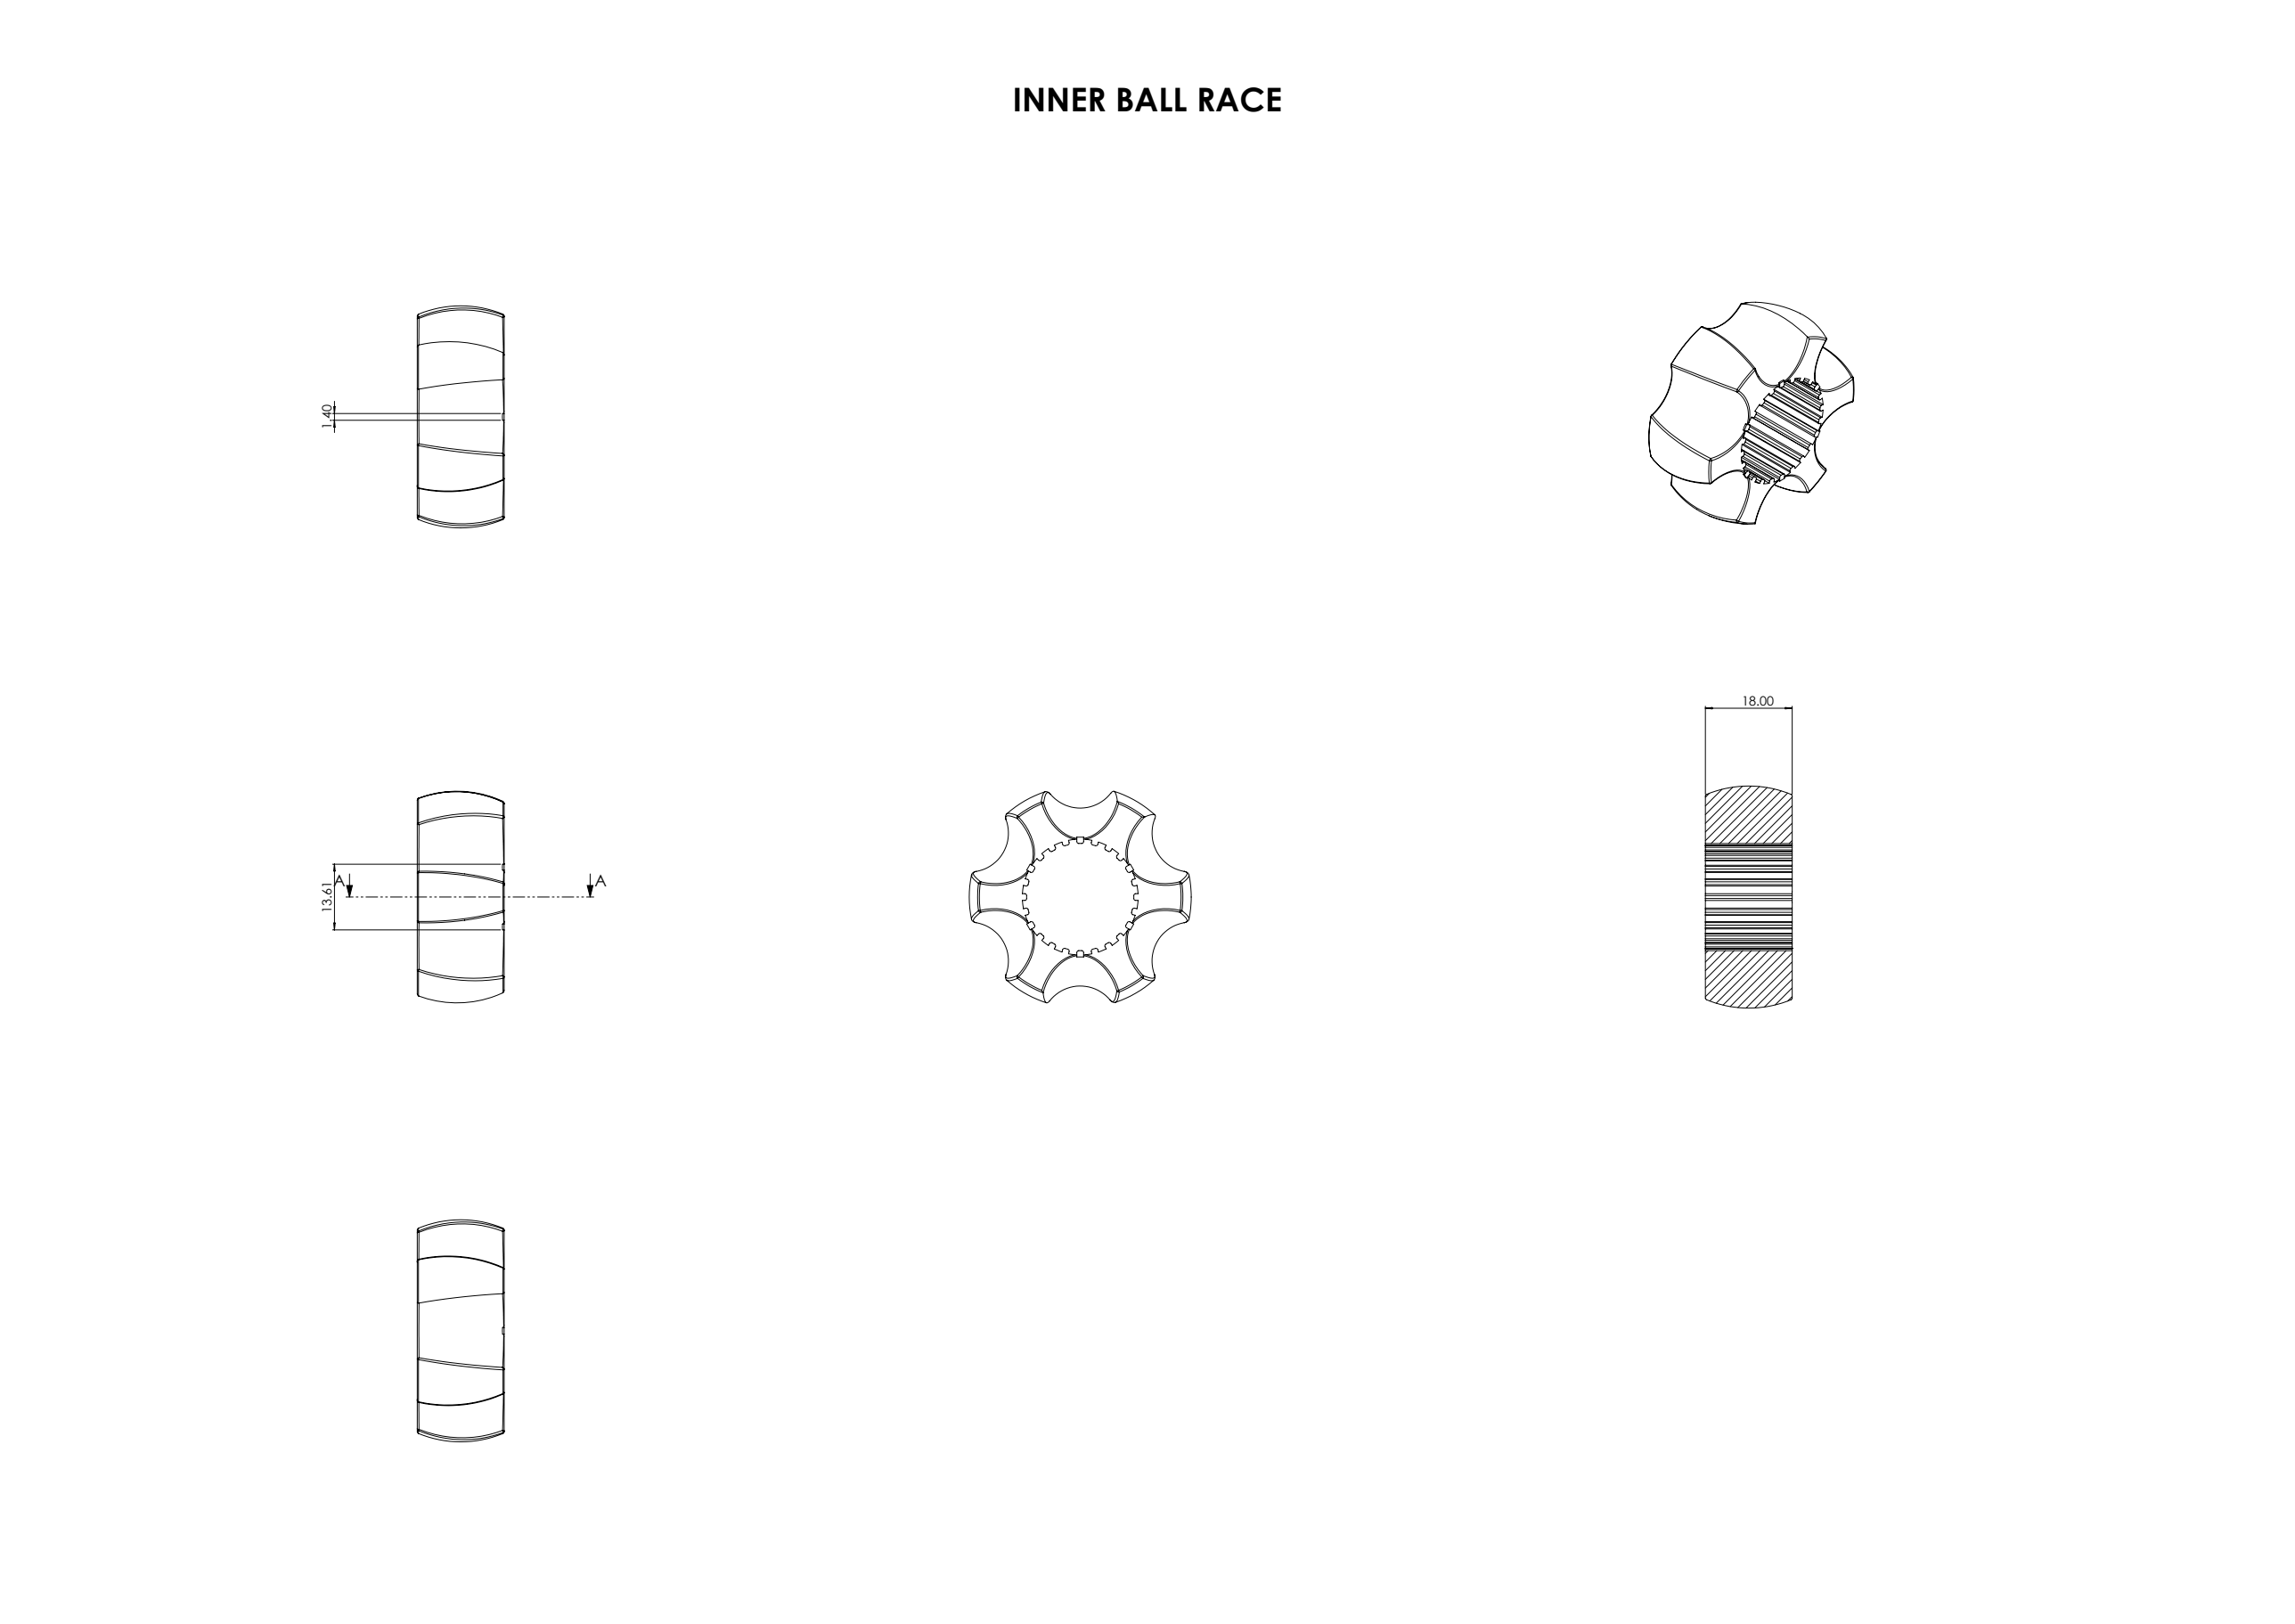
ISO-10303-21;
HEADER;
/* Generated by software containing ST-Developer
 * from STEP Tools, Inc. (www.steptools.com) 
 */

FILE_DESCRIPTION(
/* description */ (''),
/* implementation_level */ '2;1');

FILE_NAME(
/* name */ '04_Inner_Ball_Race.step',
/* time_stamp */ '2026-10-11T12:57:03-07:00',
/* author */ (''),
/* organization */ (''),
/* preprocessor_version */ 'ST-DEVELOPER v20.2',
/* originating_system */ 'Autodesk Translation Framework v15.15.0.0',
/* authorisation */ '');

FILE_SCHEMA (('AUTOMOTIVE_DESIGN { 1 0 10303 214 3 1 1 }'));
ENDSEC;

DATA;
#10=MECHANICAL_DESIGN_GEOMETRIC_PRESENTATION_REPRESENTATION('',(#259),#90374);
#225=SHAPE_REPRESENTATION_RELATIONSHIP('SRR','None',#90444,#242);
#242=ADVANCED_BREP_SHAPE_REPRESENTATION('',(#276),#90360);
#259=STYLED_ITEM('',(#90680),#276);
#276=MANIFOLD_SOLID_BREP('Body1',#40348);
#533=SPHERICAL_SURFACE('',#43538,0.4);
#534=SPHERICAL_SURFACE('',#43541,0.4);
#535=SPHERICAL_SURFACE('',#43552,0.4);
#536=SPHERICAL_SURFACE('',#43555,0.4);
#537=SPHERICAL_SURFACE('',#43561,23.);
#538=SPHERICAL_SURFACE('',#43563,0.4);
#539=SPHERICAL_SURFACE('',#43569,0.4);
#540=SPHERICAL_SURFACE('',#43581,0.4);
#541=SPHERICAL_SURFACE('',#43589,0.4);
#542=SPHERICAL_SURFACE('',#43591,0.4);
#543=SPHERICAL_SURFACE('',#43600,0.4);
#544=SPHERICAL_SURFACE('',#43603,0.4);
#545=SPHERICAL_SURFACE('',#43607,23.);
#546=SPHERICAL_SURFACE('',#43612,0.4);
#547=SPHERICAL_SURFACE('',#43616,0.399999999999991);
#548=SPHERICAL_SURFACE('',#43619,0.4);
#549=SPHERICAL_SURFACE('',#43625,0.4);
#550=SPHERICAL_SURFACE('',#43629,0.4);
#551=SPHERICAL_SURFACE('',#43632,23.);
#552=SPHERICAL_SURFACE('',#43635,0.4);
#553=SPHERICAL_SURFACE('',#43638,23.);
#554=SPHERICAL_SURFACE('',#43641,0.4);
#555=SPHERICAL_SURFACE('',#43650,23.);
#556=SPHERICAL_SURFACE('',#43653,23.);
#973=TOROIDAL_SURFACE('',#43544,20.899760764181,0.4);
#974=TOROIDAL_SURFACE('',#43547,26.4764045897475,8.05);
#975=TOROIDAL_SURFACE('',#43558,20.899760764181,0.4);
#976=TOROIDAL_SURFACE('',#43566,20.899760764181,0.4);
#977=TOROIDAL_SURFACE('',#43573,20.899760764181,0.4);
#978=TOROIDAL_SURFACE('',#43578,26.4764045897475,8.05);
#979=TOROIDAL_SURFACE('',#43584,20.899760764181,0.4);
#980=TOROIDAL_SURFACE('',#43593,20.899760764181,0.4);
#981=TOROIDAL_SURFACE('',#43596,26.4764045897475,8.05);
#982=TOROIDAL_SURFACE('',#43605,20.899760764181,0.4);
#983=TOROIDAL_SURFACE('',#43609,20.899760764181,0.4);
#984=TOROIDAL_SURFACE('',#43610,20.899760764181,0.4);
#985=TOROIDAL_SURFACE('',#43615,26.4764045897475,8.05);
#986=TOROIDAL_SURFACE('',#43623,20.899760764181,0.4);
#987=TOROIDAL_SURFACE('',#43634,26.4764045897475,8.05);
#988=TOROIDAL_SURFACE('',#43645,20.899760764181,0.4);
#989=TOROIDAL_SURFACE('',#43647,26.4764045897475,8.05);
#990=TOROIDAL_SURFACE('',#43651,20.899760764181,0.4);
#1052=FACE_BOUND('',#5964,.T.);
#1329=PLANE('',#43279);
#1330=PLANE('',#43281);
#1331=PLANE('',#43287);
#1332=PLANE('',#43288);
#1333=PLANE('',#43366);
#1334=PLANE('',#43367);
#1335=PLANE('',#43378);
#1336=PLANE('',#43381);
#1337=PLANE('',#43385);
#1338=PLANE('',#43387);
#1339=PLANE('',#43391);
#1340=PLANE('',#43402);
#1341=PLANE('',#43405);
#1342=PLANE('',#43407);
#1343=PLANE('',#43409);
#1344=PLANE('',#43411);
#1345=PLANE('',#43414);
#1346=PLANE('',#43418);
#1347=PLANE('',#43420);
#1348=PLANE('',#43423);
#1349=PLANE('',#43434);
#1350=PLANE('',#43437);
#1351=PLANE('',#43439);
#1352=PLANE('',#43441);
#1353=PLANE('',#43443);
#1354=PLANE('',#43446);
#1355=PLANE('',#43450);
#1356=PLANE('',#43452);
#1357=PLANE('',#43455);
#1358=PLANE('',#43466);
#1359=PLANE('',#43469);
#1360=PLANE('',#43471);
#1361=PLANE('',#43473);
#1362=PLANE('',#43475);
#1363=PLANE('',#43478);
#1364=PLANE('',#43482);
#1365=PLANE('',#43484);
#1366=PLANE('',#43487);
#1367=PLANE('',#43498);
#1368=PLANE('',#43501);
#1369=PLANE('',#43503);
#1370=PLANE('',#43505);
#1371=PLANE('',#43507);
#1372=PLANE('',#43510);
#1373=PLANE('',#43514);
#1374=PLANE('',#43516);
#1375=PLANE('',#43519);
#1376=PLANE('',#43530);
#1377=PLANE('',#43533);
#1378=PLANE('',#43535);
#1379=PLANE('',#43655);
#1380=PLANE('',#43657);
#1381=PLANE('',#43658);
#1382=PLANE('',#43660);
#1383=PLANE('',#43663);
#1384=PLANE('',#43664);
#1385=PLANE('',#43665);
#1386=PLANE('',#43666);
#1387=PLANE('',#43668);
#1388=PLANE('',#43670);
#1389=PLANE('',#43673);
#1390=PLANE('',#43674);
#1391=PLANE('',#43675);
#1392=PLANE('',#43676);
#1393=PLANE('',#43678);
#1394=PLANE('',#43680);
#1395=PLANE('',#43682);
#1396=PLANE('',#43683);
#1397=PLANE('',#43684);
#1398=PLANE('',#43685);
#1399=PLANE('',#43687);
#1400=PLANE('',#43689);
#1401=PLANE('',#43692);
#1402=PLANE('',#43693);
#1403=PLANE('',#43694);
#1404=PLANE('',#43695);
#1405=PLANE('',#43697);
#1406=PLANE('',#43699);
#1407=PLANE('',#43702);
#1408=PLANE('',#43703);
#1409=PLANE('',#43704);
#1410=PLANE('',#43705);
#1411=PLANE('',#43706);
#1412=PLANE('',#43708);
#1413=PLANE('',#43709);
#1414=PLANE('',#43710);
#1415=PLANE('',#43711);
#1416=PLANE('',#43713);
#1417=PLANE('',#43716);
#1418=PLANE('',#43717);
#1419=PLANE('',#43718);
#2106=B_SPLINE_SURFACE_WITH_KNOTS('',3,3,((#79480,#79481,#79482,#79483,
#79484),(#79485,#79486,#79487,#79488,#79489),(#79490,#79491,#79492,#79493,
#79494),(#79495,#79496,#79497,#79498,#79499),(#79500,#79501,#79502,#79503,
#79504)),.UNSPECIFIED.,.F.,.F.,.F.,(4,1,4),(4,1,4),(0.,0.5,1.),(0.,0.763473638149737,
1.78143848901605),.UNSPECIFIED.);
#2107=B_SPLINE_SURFACE_WITH_KNOTS('',3,3,((#79531,#79532,#79533,#79534,
#79535,#79536),(#79537,#79538,#79539,#79540,#79541,#79542),(#79543,#79544,
#79545,#79546,#79547,#79548),(#79549,#79550,#79551,#79552,#79553,#79554),
(#79555,#79556,#79557,#79558,#79559,#79560)),.UNSPECIFIED.,.F.,.F.,.F.,
(4,1,4),(4,1,1,4),(0.,0.5,1.),(0.285566041444528,0.852705185028571,1.23079794741793,
1.6088907098073),.UNSPECIFIED.);
#2108=B_SPLINE_SURFACE_WITH_KNOTS('',3,3,((#79645,#79646,#79647,#79648,
#79649),(#79650,#79651,#79652,#79653,#79654),(#79655,#79656,#79657,#79658,
#79659),(#79660,#79661,#79662,#79663,#79664),(#79665,#79666,#79667,#79668,
#79669)),.UNSPECIFIED.,.F.,.F.,.F.,(4,1,4),(4,1,4),(0.,0.5,1.),(0.,0.763473638150805,
1.78143848901855),.UNSPECIFIED.);
#2109=B_SPLINE_SURFACE_WITH_KNOTS('',3,3,((#79692,#79693,#79694,#79695,
#79696,#79697),(#79698,#79699,#79700,#79701,#79702,#79703),(#79704,#79705,
#79706,#79707,#79708,#79709),(#79710,#79711,#79712,#79713,#79714,#79715),
(#79716,#79717,#79718,#79719,#79720,#79721)),.UNSPECIFIED.,.F.,.F.,.F.,
(4,1,4),(4,1,1,4),(0.,0.5,1.),(1.29377116963159,1.60639339394931,1.91901561826703,
2.38794895474362),.UNSPECIFIED.);
#2110=B_SPLINE_SURFACE_WITH_KNOTS('',3,3,((#79782,#79783,#79784,#79785,
#79786,#79787),(#79788,#79789,#79790,#79791,#79792,#79793),(#79794,#79795,
#79796,#79797,#79798,#79799),(#79800,#79801,#79802,#79803,#79804,#79805),
(#79806,#79807,#79808,#79809,#79810,#79811)),.UNSPECIFIED.,.F.,.F.,.F.,
(4,1,4),(4,1,1,4),(0.,0.5,1.),(0.738839250765249,1.30597756136174,1.68406976842606,
2.06216197549039),.UNSPECIFIED.);
#2111=B_SPLINE_SURFACE_WITH_KNOTS('',3,3,((#79835,#79836,#79837,#79838,
#79839,#79840),(#79841,#79842,#79843,#79844,#79845,#79846),(#79847,#79848,
#79849,#79850,#79851,#79852),(#79853,#79854,#79855,#79856,#79857,#79858),
(#79859,#79860,#79861,#79862,#79863,#79864)),.UNSPECIFIED.,.F.,.F.,.F.,
(4,1,4),(4,1,1,4),(0.,0.5,1.),(0.263863277597402,0.819957327863798,1.19068669470806,
1.56141606155233),.UNSPECIFIED.);
#2112=B_SPLINE_SURFACE_WITH_KNOTS('',3,3,((#79879,#79880,#79881,#79882,
#79883),(#79884,#79885,#79886,#79887,#79888),(#79889,#79890,#79891,#79892,
#79893),(#79894,#79895,#79896,#79897,#79898),(#79899,#79900,#79901,#79902,
#79903)),.UNSPECIFIED.,.F.,.F.,.F.,(4,1,4),(4,1,4),(0.,0.5,1.),(0.805732136131231,
1.56919017940703,2.5871342371081),.UNSPECIFIED.);
#2113=B_SPLINE_SURFACE_WITH_KNOTS('',3,3,((#79949,#79950,#79951,#79952,
#79953),(#79954,#79955,#79956,#79957,#79958),(#79959,#79960,#79961,#79962,
#79963),(#79964,#79965,#79966,#79967,#79968),(#79969,#79970,#79971,#79972,
#79973)),.UNSPECIFIED.,.F.,.F.,.F.,(4,1,4),(4,1,4),(0.,0.5,1.),(0.,0.763473508304906,
1.78143818604478),.UNSPECIFIED.);
#2114=B_SPLINE_SURFACE_WITH_KNOTS('',3,3,((#80008,#80009,#80010,#80011,
#80012,#80013),(#80014,#80015,#80016,#80017,#80018,#80019),(#80020,#80021,
#80022,#80023,#80024,#80025),(#80026,#80027,#80028,#80029,#80030,#80031),
(#80032,#80033,#80034,#80035,#80036,#80037)),.UNSPECIFIED.,.F.,.F.,.F.,
(4,1,4),(4,1,1,4),(0.,0.5,1.),(0.232788919908364,0.858032407070129,1.01434327886057,
1.32696502244145),.UNSPECIFIED.);
#2115=B_SPLINE_SURFACE_WITH_KNOTS('',3,3,((#80074,#80075,#80076,#80077,
#80078,#80079),(#80080,#80081,#80082,#80083,#80084,#80085),(#80086,#80087,
#80088,#80089,#80090,#80091),(#80092,#80093,#80094,#80095,#80096,#80097),
(#80098,#80099,#80100,#80101,#80102,#80103)),.UNSPECIFIED.,.F.,.F.,.F.,
(4,1,4),(4,1,1,4),(0.,0.5,1.),(0.764611228840875,1.32070527910915,1.69143464595466,
2.06216401280017),.UNSPECIFIED.);
#2116=B_SPLINE_SURFACE_WITH_KNOTS('',3,3,((#80105,#80106,#80107,#80108,
#80109),(#80110,#80111,#80112,#80113,#80114),(#80115,#80116,#80117,#80118,
#80119),(#80120,#80121,#80122,#80123,#80124),(#80125,#80126,#80127,#80128,
#80129)),.UNSPECIFIED.,.F.,.F.,.F.,(4,1,4),(4,1,4),(0.,0.5,1.),(0.,0.763473564994705,
1.78143831832098),.UNSPECIFIED.);
#2117=B_SPLINE_SURFACE_WITH_KNOTS('',3,3,((#80144,#80145,#80146,#80147,
#80148,#80149),(#80150,#80151,#80152,#80153,#80154,#80155),(#80156,#80157,
#80158,#80159,#80160,#80161),(#80162,#80163,#80164,#80165,#80166,#80167),
(#80168,#80169,#80170,#80171,#80172,#80173)),.UNSPECIFIED.,.F.,.F.,.F.,
(4,1,4),(4,1,1,4),(0.,0.5,1.),(1.46996194814535,1.78258352306356,2.09520509798177,
2.56413746035908),.UNSPECIFIED.);
#2118=B_SPLINE_SURFACE_WITH_KNOTS('',3,3,((#80260,#80261,#80262,#80263,
#80264,#80265),(#80266,#80267,#80268,#80269,#80270,#80271),(#80272,#80273,
#80274,#80275,#80276,#80277),(#80278,#80279,#80280,#80281,#80282,#80283),
(#80284,#80285,#80286,#80287,#80288,#80289)),.UNSPECIFIED.,.F.,.F.,.F.,
(4,1,4),(4,1,1,4),(0.,0.5,1.),(0.285566041444524,0.663658803833889,1.04175156622325,
1.6088907098073),.UNSPECIFIED.);
#2119=B_SPLINE_SURFACE_WITH_KNOTS('',3,3,((#80312,#80313,#80314,#80315,
#80316,#80317),(#80318,#80319,#80320,#80321,#80322,#80323),(#80324,#80325,
#80326,#80327,#80328,#80329),(#80330,#80331,#80332,#80333,#80334,#80335),
(#80336,#80337,#80338,#80339,#80340,#80341)),.UNSPECIFIED.,.F.,.F.,.F.,
(4,1,4),(4,1,1,4),(0.,0.5,1.),(0.232788566406526,0.70171854409386,1.01433852921875,
1.32695851434364),.UNSPECIFIED.);
#2120=B_SPLINE_SURFACE_WITH_KNOTS('',3,3,((#80358,#80359,#80360,#80361,
#80362,#80363),(#80364,#80365,#80366,#80367,#80368,#80369),(#80370,#80371,
#80372,#80373,#80374,#80375),(#80376,#80377,#80378,#80379,#80380,#80381),
(#80382,#80383,#80384,#80385,#80386,#80387)),.UNSPECIFIED.,.F.,.F.,.F.,
(4,1,4),(4,1,1,4),(0.,0.5,1.),(0.263863277598129,0.819957327864215,1.19068669470827,
1.56141606155233),.UNSPECIFIED.);
#2121=B_SPLINE_SURFACE_WITH_KNOTS('',3,3,((#80394,#80395,#80396,#80397,
#80398,#80399),(#80400,#80401,#80402,#80403,#80404,#80405),(#80406,#80407,
#80408,#80409,#80410,#80411),(#80412,#80413,#80414,#80415,#80416,#80417),
(#80418,#80419,#80420,#80421,#80422,#80423)),.UNSPECIFIED.,.F.,.F.,.F.,
(4,1,4),(4,1,1,4),(0.,0.5,1.),(1.38151698616895,1.53782715631916,1.85044749661957,
2.47568817722038),.UNSPECIFIED.);
#2122=B_SPLINE_SURFACE_WITH_KNOTS('',3,3,((#80434,#80435,#80436,#80437,
#80438),(#80439,#80440,#80441,#80442,#80443),(#80444,#80445,#80446,#80447,
#80448),(#80449,#80450,#80451,#80452,#80453),(#80454,#80455,#80456,#80457,
#80458)),.UNSPECIFIED.,.F.,.F.,.F.,(4,1,4),(4,1,4),(0.,0.5,1.),(0.836467246372547,
1.5999252909985,2.61786935049977),.UNSPECIFIED.);
#2123=B_SPLINE_SURFACE_WITH_KNOTS('',3,3,((#80469,#80470,#80471,#80472,
#80473),(#80474,#80475,#80476,#80477,#80478),(#80479,#80480,#80481,#80482,
#80483),(#80484,#80485,#80486,#80487,#80488),(#80489,#80490,#80491,#80492,
#80493)),.UNSPECIFIED.,.F.,.F.,.F.,(4,1,4),(4,1,4),(0.,0.5,1.),(0.733284842491785,
1.49674691578015,2.51469634683131),.UNSPECIFIED.);
#2124=B_SPLINE_SURFACE_WITH_KNOTS('',3,3,((#80508,#80509,#80510,#80511,
#80512,#80513),(#80514,#80515,#80516,#80517,#80518,#80519),(#80520,#80521,
#80522,#80523,#80524,#80525),(#80526,#80527,#80528,#80529,#80530,#80531),
(#80532,#80533,#80534,#80535,#80536,#80537)),.UNSPECIFIED.,.F.,.F.,.F.,
(4,1,4),(4,1,1,4),(0.,0.5,1.),(1.11836314594235,1.58729550831966,1.89991708323787,
2.21253865815608),.UNSPECIFIED.);
#2125=B_SPLINE_SURFACE_WITH_KNOTS('',3,3,((#80555,#80556,#80557,#80558,
#80559,#80560),(#80561,#80562,#80563,#80564,#80565,#80566),(#80567,#80568,
#80569,#80570,#80571,#80572),(#80573,#80574,#80575,#80576,#80577,#80578),
(#80579,#80580,#80581,#80582,#80583,#80584)),.UNSPECIFIED.,.F.,.F.,.F.,
(4,1,4),(4,1,1,4),(0.,0.5,1.),(0.261933028354804,0.750578938128915,1.07634287797832,
1.40210681782773),.UNSPECIFIED.);
#2126=B_SPLINE_SURFACE_WITH_KNOTS('',3,3,((#80601,#80602,#80603,#80604,
#80605),(#80606,#80607,#80608,#80609,#80610),(#80611,#80612,#80613,#80614,
#80615),(#80616,#80617,#80618,#80619,#80620),(#80621,#80622,#80623,#80624,
#80625)),.UNSPECIFIED.,.F.,.F.,.F.,(4,1,4),(4,1,4),(0.,0.5,1.),(0.836467246372557,
1.59992529099851,2.61786935049979),.UNSPECIFIED.);
#2127=B_SPLINE_SURFACE_WITH_KNOTS('',3,3,((#80631,#80632,#80633,#80634,
#80635,#80636),(#80637,#80638,#80639,#80640,#80641,#80642),(#80643,#80644,
#80645,#80646,#80647,#80648),(#80649,#80650,#80651,#80652,#80653,#80654),
(#80655,#80656,#80657,#80658,#80659,#80660)),.UNSPECIFIED.,.F.,.F.,.F.,
(4,1,4),(4,1,1,4),(0.,0.5,1.),(1.38152124201424,1.53783209167054,1.85045379098313,
2.47569718960832),.UNSPECIFIED.);
#2128=B_SPLINE_SURFACE_WITH_KNOTS('',3,3,((#80686,#80687,#80688,#80689,
#80690),(#80691,#80692,#80693,#80694,#80695),(#80696,#80697,#80698,#80699,
#80700),(#80701,#80702,#80703,#80704,#80705),(#80706,#80707,#80708,#80709,
#80710)),.UNSPECIFIED.,.F.,.F.,.F.,(4,1,4),(4,1,4),(0.,0.5,1.),(0.733284842491785,
1.49674691578015,2.51469634683131),.UNSPECIFIED.);
#2129=B_SPLINE_SURFACE_WITH_KNOTS('',3,3,((#80730,#80731,#80732,#80733,
#80734,#80735),(#80736,#80737,#80738,#80739,#80740,#80741),(#80742,#80743,
#80744,#80745,#80746,#80747),(#80748,#80749,#80750,#80751,#80752,#80753),
(#80754,#80755,#80756,#80757,#80758,#80759)),.UNSPECIFIED.,.F.,.F.,.F.,
(4,1,4),(4,1,1,4),(0.,0.5,1.),(1.11836314594235,1.58729550831966,1.89991708323787,
2.21253865815608),.UNSPECIFIED.);
#2130=B_SPLINE_SURFACE_WITH_KNOTS('',3,3,((#80787,#80788,#80789,#80790,
#80791,#80792),(#80793,#80794,#80795,#80796,#80797,#80798),(#80799,#80800,
#80801,#80802,#80803,#80804),(#80805,#80806,#80807,#80808,#80809,#80810),
(#80811,#80812,#80813,#80814,#80815,#80816)),.UNSPECIFIED.,.F.,.F.,.F.,
(4,1,4),(4,1,1,4),(0.,0.5,1.),(1.54510505491245,1.70141616706786,2.0140383913787,
2.63928284000037),.UNSPECIFIED.);
#2131=B_SPLINE_SURFACE_WITH_KNOTS('',3,3,((#80847,#80848,#80849,#80850,
#80851,#80852),(#80853,#80854,#80855,#80856,#80857,#80858),(#80859,#80860,
#80861,#80862,#80863,#80864),(#80865,#80866,#80867,#80868,#80869,#80870),
(#80871,#80872,#80873,#80874,#80875,#80876)),.UNSPECIFIED.,.F.,.F.,.F.,
(4,1,4),(4,1,1,4),(0.,0.5,1.),(0.261933028354807,0.750578938128917,1.07634287797832,
1.40210681782773),.UNSPECIFIED.);
#2132=B_SPLINE_SURFACE_WITH_KNOTS('',3,3,((#80926,#80927,#80928,#80929,
#80930,#80931),(#80932,#80933,#80934,#80935,#80936,#80937),(#80938,#80939,
#80940,#80941,#80942,#80943),(#80944,#80945,#80946,#80947,#80948,#80949),
(#80950,#80951,#80952,#80953,#80954,#80955)),.UNSPECIFIED.,.F.,.F.,.F.,
(4,1,4),(4,1,1,4),(0.,0.5,1.),(1.46996194814535,1.79572424429708,1.95860539237294,
2.6101299846764),.UNSPECIFIED.);
#3548=FACE_OUTER_BOUND('',#5957,.T.);
#3549=FACE_OUTER_BOUND('',#5958,.T.);
#3550=FACE_OUTER_BOUND('',#5959,.T.);
#3551=FACE_OUTER_BOUND('',#5960,.T.);
#3552=FACE_OUTER_BOUND('',#5961,.T.);
#3553=FACE_OUTER_BOUND('',#5962,.T.);
#3554=FACE_OUTER_BOUND('',#5963,.T.);
#3555=FACE_OUTER_BOUND('',#5965,.T.);
#3556=FACE_OUTER_BOUND('',#5966,.T.);
#3557=FACE_OUTER_BOUND('',#5967,.T.);
#3558=FACE_OUTER_BOUND('',#5968,.T.);
#3559=FACE_OUTER_BOUND('',#5969,.T.);
#3560=FACE_OUTER_BOUND('',#5970,.T.);
#3561=FACE_OUTER_BOUND('',#5971,.T.);
#3562=FACE_OUTER_BOUND('',#5972,.T.);
#3563=FACE_OUTER_BOUND('',#5973,.T.);
#3564=FACE_OUTER_BOUND('',#5974,.T.);
#3565=FACE_OUTER_BOUND('',#5975,.T.);
#3566=FACE_OUTER_BOUND('',#5976,.T.);
#3567=FACE_OUTER_BOUND('',#5977,.T.);
#3568=FACE_OUTER_BOUND('',#5978,.T.);
#3569=FACE_OUTER_BOUND('',#5979,.T.);
#3570=FACE_OUTER_BOUND('',#5980,.T.);
#3571=FACE_OUTER_BOUND('',#5981,.T.);
#3572=FACE_OUTER_BOUND('',#5982,.T.);
#3573=FACE_OUTER_BOUND('',#5983,.T.);
#3574=FACE_OUTER_BOUND('',#5984,.T.);
#3575=FACE_OUTER_BOUND('',#5985,.T.);
#3576=FACE_OUTER_BOUND('',#5986,.T.);
#3577=FACE_OUTER_BOUND('',#5987,.T.);
#3578=FACE_OUTER_BOUND('',#5988,.T.);
#3579=FACE_OUTER_BOUND('',#5989,.T.);
#3580=FACE_OUTER_BOUND('',#5990,.T.);
#3581=FACE_OUTER_BOUND('',#5991,.T.);
#3582=FACE_OUTER_BOUND('',#5992,.T.);
#3583=FACE_OUTER_BOUND('',#5993,.T.);
#3584=FACE_OUTER_BOUND('',#5994,.T.);
#3585=FACE_OUTER_BOUND('',#5995,.T.);
#3586=FACE_OUTER_BOUND('',#5996,.T.);
#3587=FACE_OUTER_BOUND('',#5997,.T.);
#3588=FACE_OUTER_BOUND('',#5998,.T.);
#3589=FACE_OUTER_BOUND('',#5999,.T.);
#3590=FACE_OUTER_BOUND('',#6000,.T.);
#3591=FACE_OUTER_BOUND('',#6001,.T.);
#3592=FACE_OUTER_BOUND('',#6002,.T.);
#3593=FACE_OUTER_BOUND('',#6003,.T.);
#3594=FACE_OUTER_BOUND('',#6004,.T.);
#3595=FACE_OUTER_BOUND('',#6005,.T.);
#3596=FACE_OUTER_BOUND('',#6006,.T.);
#3597=FACE_OUTER_BOUND('',#6007,.T.);
#3598=FACE_OUTER_BOUND('',#6008,.T.);
#3599=FACE_OUTER_BOUND('',#6009,.T.);
#3600=FACE_OUTER_BOUND('',#6010,.T.);
#3601=FACE_OUTER_BOUND('',#6011,.T.);
#3602=FACE_OUTER_BOUND('',#6012,.T.);
#3603=FACE_OUTER_BOUND('',#6013,.T.);
#3604=FACE_OUTER_BOUND('',#6014,.T.);
#3605=FACE_OUTER_BOUND('',#6015,.T.);
#3606=FACE_OUTER_BOUND('',#6016,.T.);
#3607=FACE_OUTER_BOUND('',#6017,.T.);
#3608=FACE_OUTER_BOUND('',#6018,.T.);
#3609=FACE_OUTER_BOUND('',#6019,.T.);
#3610=FACE_OUTER_BOUND('',#6020,.T.);
#3611=FACE_OUTER_BOUND('',#6021,.T.);
#3612=FACE_OUTER_BOUND('',#6022,.T.);
#3613=FACE_OUTER_BOUND('',#6023,.T.);
#3614=FACE_OUTER_BOUND('',#6024,.T.);
#3615=FACE_OUTER_BOUND('',#6025,.T.);
#3616=FACE_OUTER_BOUND('',#6026,.T.);
#3617=FACE_OUTER_BOUND('',#6027,.T.);
#3618=FACE_OUTER_BOUND('',#6028,.T.);
#3619=FACE_OUTER_BOUND('',#6029,.T.);
#3620=FACE_OUTER_BOUND('',#6030,.T.);
#3621=FACE_OUTER_BOUND('',#6031,.T.);
#3622=FACE_OUTER_BOUND('',#6032,.T.);
#3623=FACE_OUTER_BOUND('',#6033,.T.);
#3624=FACE_OUTER_BOUND('',#6034,.T.);
#3625=FACE_OUTER_BOUND('',#6035,.T.);
#3626=FACE_OUTER_BOUND('',#6036,.T.);
#3627=FACE_OUTER_BOUND('',#6037,.T.);
#3628=FACE_OUTER_BOUND('',#6038,.T.);
#3629=FACE_OUTER_BOUND('',#6039,.T.);
#3630=FACE_OUTER_BOUND('',#6040,.T.);
#3631=FACE_OUTER_BOUND('',#6041,.T.);
#3632=FACE_OUTER_BOUND('',#6042,.T.);
#3633=FACE_OUTER_BOUND('',#6043,.T.);
#3634=FACE_OUTER_BOUND('',#6044,.T.);
#3635=FACE_OUTER_BOUND('',#6045,.T.);
#3636=FACE_OUTER_BOUND('',#6046,.T.);
#3637=FACE_OUTER_BOUND('',#6047,.T.);
#3638=FACE_OUTER_BOUND('',#6048,.T.);
#3639=FACE_OUTER_BOUND('',#6049,.T.);
#3640=FACE_OUTER_BOUND('',#6050,.T.);
#3641=FACE_OUTER_BOUND('',#6051,.T.);
#3642=FACE_OUTER_BOUND('',#6052,.T.);
#3643=FACE_OUTER_BOUND('',#6053,.T.);
#3644=FACE_OUTER_BOUND('',#6054,.T.);
#3645=FACE_OUTER_BOUND('',#6055,.T.);
#3646=FACE_OUTER_BOUND('',#6056,.T.);
#3647=FACE_OUTER_BOUND('',#6057,.T.);
#3648=FACE_OUTER_BOUND('',#6058,.T.);
#3649=FACE_OUTER_BOUND('',#6059,.T.);
#3650=FACE_OUTER_BOUND('',#6060,.T.);
#3651=FACE_OUTER_BOUND('',#6061,.T.);
#3652=FACE_OUTER_BOUND('',#6062,.T.);
#3653=FACE_OUTER_BOUND('',#6063,.T.);
#3654=FACE_OUTER_BOUND('',#6064,.T.);
#3655=FACE_OUTER_BOUND('',#6065,.T.);
#3656=FACE_OUTER_BOUND('',#6066,.T.);
#3657=FACE_OUTER_BOUND('',#6067,.T.);
#3658=FACE_OUTER_BOUND('',#6068,.T.);
#3659=FACE_OUTER_BOUND('',#6069,.T.);
#3660=FACE_OUTER_BOUND('',#6070,.T.);
#3661=FACE_OUTER_BOUND('',#6071,.T.);
#3662=FACE_OUTER_BOUND('',#6072,.T.);
#3663=FACE_OUTER_BOUND('',#6073,.T.);
#3664=FACE_OUTER_BOUND('',#6074,.T.);
#3665=FACE_OUTER_BOUND('',#6075,.T.);
#3666=FACE_OUTER_BOUND('',#6076,.T.);
#3667=FACE_OUTER_BOUND('',#6077,.T.);
#3668=FACE_OUTER_BOUND('',#6078,.T.);
#3669=FACE_OUTER_BOUND('',#6079,.T.);
#3670=FACE_OUTER_BOUND('',#6080,.T.);
#3671=FACE_OUTER_BOUND('',#6081,.T.);
#3672=FACE_OUTER_BOUND('',#6082,.T.);
#3673=FACE_OUTER_BOUND('',#6083,.T.);
#3674=FACE_OUTER_BOUND('',#6084,.T.);
#3675=FACE_OUTER_BOUND('',#6085,.T.);
#3676=FACE_OUTER_BOUND('',#6086,.T.);
#3677=FACE_OUTER_BOUND('',#6087,.T.);
#3678=FACE_OUTER_BOUND('',#6088,.T.);
#3679=FACE_OUTER_BOUND('',#6089,.T.);
#3680=FACE_OUTER_BOUND('',#6090,.T.);
#3681=FACE_OUTER_BOUND('',#6091,.T.);
#3682=FACE_OUTER_BOUND('',#6092,.T.);
#3683=FACE_OUTER_BOUND('',#6093,.T.);
#3684=FACE_OUTER_BOUND('',#6094,.T.);
#3685=FACE_OUTER_BOUND('',#6095,.T.);
#3686=FACE_OUTER_BOUND('',#6096,.T.);
#3687=FACE_OUTER_BOUND('',#6097,.T.);
#3688=FACE_OUTER_BOUND('',#6098,.T.);
#3689=FACE_OUTER_BOUND('',#6099,.T.);
#3690=FACE_OUTER_BOUND('',#6100,.T.);
#3691=FACE_OUTER_BOUND('',#6101,.T.);
#3692=FACE_OUTER_BOUND('',#6102,.T.);
#3693=FACE_OUTER_BOUND('',#6103,.T.);
#3694=FACE_OUTER_BOUND('',#6104,.T.);
#3695=FACE_OUTER_BOUND('',#6105,.T.);
#3696=FACE_OUTER_BOUND('',#6106,.T.);
#3697=FACE_OUTER_BOUND('',#6107,.T.);
#3698=FACE_OUTER_BOUND('',#6108,.T.);
#3699=FACE_OUTER_BOUND('',#6109,.T.);
#3700=FACE_OUTER_BOUND('',#6110,.T.);
#3701=FACE_OUTER_BOUND('',#6111,.T.);
#3702=FACE_OUTER_BOUND('',#6112,.T.);
#3703=FACE_OUTER_BOUND('',#6113,.T.);
#3704=FACE_OUTER_BOUND('',#6114,.T.);
#3705=FACE_OUTER_BOUND('',#6115,.T.);
#3706=FACE_OUTER_BOUND('',#6116,.T.);
#3707=FACE_OUTER_BOUND('',#6117,.T.);
#3708=FACE_OUTER_BOUND('',#6118,.T.);
#3709=FACE_OUTER_BOUND('',#6119,.T.);
#3710=FACE_OUTER_BOUND('',#6120,.T.);
#3711=FACE_OUTER_BOUND('',#6121,.T.);
#3712=FACE_OUTER_BOUND('',#6122,.T.);
#3713=FACE_OUTER_BOUND('',#6123,.T.);
#3714=FACE_OUTER_BOUND('',#6124,.T.);
#3715=FACE_OUTER_BOUND('',#6125,.T.);
#3716=FACE_OUTER_BOUND('',#6126,.T.);
#3717=FACE_OUTER_BOUND('',#6127,.T.);
#3718=FACE_OUTER_BOUND('',#6128,.T.);
#3719=FACE_OUTER_BOUND('',#6129,.T.);
#3720=FACE_OUTER_BOUND('',#6130,.T.);
#3721=FACE_OUTER_BOUND('',#6131,.T.);
#3722=FACE_OUTER_BOUND('',#6132,.T.);
#3723=FACE_OUTER_BOUND('',#6133,.T.);
#3724=FACE_OUTER_BOUND('',#6134,.T.);
#3725=FACE_OUTER_BOUND('',#6135,.T.);
#3726=FACE_OUTER_BOUND('',#6136,.T.);
#3727=FACE_OUTER_BOUND('',#6137,.T.);
#3728=FACE_OUTER_BOUND('',#6138,.T.);
#3729=FACE_OUTER_BOUND('',#6139,.T.);
#3730=FACE_OUTER_BOUND('',#6140,.T.);
#3731=FACE_OUTER_BOUND('',#6141,.T.);
#3732=FACE_OUTER_BOUND('',#6142,.T.);
#3733=FACE_OUTER_BOUND('',#6143,.T.);
#3734=FACE_OUTER_BOUND('',#6144,.T.);
#3735=FACE_OUTER_BOUND('',#6145,.T.);
#3736=FACE_OUTER_BOUND('',#6146,.T.);
#3737=FACE_OUTER_BOUND('',#6147,.T.);
#3738=FACE_OUTER_BOUND('',#6148,.T.);
#3739=FACE_OUTER_BOUND('',#6149,.T.);
#3740=FACE_OUTER_BOUND('',#6150,.T.);
#3741=FACE_OUTER_BOUND('',#6151,.T.);
#3742=FACE_OUTER_BOUND('',#6152,.T.);
#3743=FACE_OUTER_BOUND('',#6153,.T.);
#3744=FACE_OUTER_BOUND('',#6154,.T.);
#3745=FACE_OUTER_BOUND('',#6155,.T.);
#3746=FACE_OUTER_BOUND('',#6156,.T.);
#3747=FACE_OUTER_BOUND('',#6157,.T.);
#3748=FACE_OUTER_BOUND('',#6158,.T.);
#3749=FACE_OUTER_BOUND('',#6159,.T.);
#3750=FACE_OUTER_BOUND('',#6160,.T.);
#3751=FACE_OUTER_BOUND('',#6161,.T.);
#3752=FACE_OUTER_BOUND('',#6162,.T.);
#3753=FACE_OUTER_BOUND('',#6163,.T.);
#3754=FACE_OUTER_BOUND('',#6164,.T.);
#3755=FACE_OUTER_BOUND('',#6165,.T.);
#3756=FACE_OUTER_BOUND('',#6166,.T.);
#3757=FACE_OUTER_BOUND('',#6167,.T.);
#3758=FACE_OUTER_BOUND('',#6168,.T.);
#3759=FACE_OUTER_BOUND('',#6169,.T.);
#3760=FACE_OUTER_BOUND('',#6170,.T.);
#3761=FACE_OUTER_BOUND('',#6171,.T.);
#3762=FACE_OUTER_BOUND('',#6172,.T.);
#3763=FACE_OUTER_BOUND('',#6173,.T.);
#3764=FACE_OUTER_BOUND('',#6174,.T.);
#3765=FACE_OUTER_BOUND('',#6175,.T.);
#3766=FACE_OUTER_BOUND('',#6176,.T.);
#3767=FACE_OUTER_BOUND('',#6177,.T.);
#3768=FACE_OUTER_BOUND('',#6178,.T.);
#3769=FACE_OUTER_BOUND('',#6179,.T.);
#3770=FACE_OUTER_BOUND('',#6180,.T.);
#3771=FACE_OUTER_BOUND('',#6181,.T.);
#3772=FACE_OUTER_BOUND('',#6182,.T.);
#3773=FACE_OUTER_BOUND('',#6183,.T.);
#3774=FACE_OUTER_BOUND('',#6184,.T.);
#3775=FACE_OUTER_BOUND('',#6185,.T.);
#3776=FACE_OUTER_BOUND('',#6186,.T.);
#3777=FACE_OUTER_BOUND('',#6187,.T.);
#3778=FACE_OUTER_BOUND('',#6188,.T.);
#3779=FACE_OUTER_BOUND('',#6189,.T.);
#5957=EDGE_LOOP('',(#31813,#31814,#31815,#31816));
#5958=EDGE_LOOP('',(#31817,#31818,#31819,#31820,#31821,#31822));
#5959=EDGE_LOOP('',(#31823,#31824,#31825,#31826));
#5960=EDGE_LOOP('',(#31827,#31828,#31829,#31830));
#5961=EDGE_LOOP('',(#31831,#31832,#31833,#31834));
#5962=EDGE_LOOP('',(#31835,#31836,#31837,#31838));
#5963=EDGE_LOOP('',(#31839,#31840,#31841,#31842,#31843,#31844,#31845,#31846,
#31847,#31848,#31849,#31850));
#5964=EDGE_LOOP('',(#31851,#31852,#31853,#31854,#31855,#31856,#31857,#31858,
#31859,#31860,#31861,#31862,#31863,#31864,#31865,#31866,#31867,#31868,#31869,
#31870,#31871,#31872,#31873,#31874,#31875,#31876,#31877,#31878,#31879,#31880,
#31881,#31882,#31883,#31884,#31885,#31886,#31887,#31888,#31889,#31890,#31891,
#31892,#31893,#31894,#31895,#31896,#31897,#31898,#31899,#31900,#31901,#31902,
#31903,#31904,#31905,#31906,#31907,#31908,#31909,#31910,#31911,#31912,#31913,
#31914,#31915,#31916,#31917,#31918,#31919,#31920,#31921,#31922,#31923,#31924,
#31925,#31926,#31927,#31928,#31929,#31930,#31931,#31932,#31933,#31934,#31935,
#31936,#31937,#31938,#31939,#31940,#31941,#31942,#31943,#31944,#31945,#31946,
#31947,#31948,#31949,#31950,#31951,#31952,#31953,#31954,#31955,#31956,#31957,
#31958,#31959,#31960,#31961,#31962,#31963,#31964,#31965,#31966,#31967,#31968,
#31969,#31970,#31971,#31972,#31973,#31974,#31975,#31976,#31977,#31978,#31979,
#31980,#31981,#31982,#31983,#31984,#31985,#31986,#31987,#31988,#31989,#31990,
#31991,#31992,#31993,#31994));
#5965=EDGE_LOOP('',(#31995,#31996,#31997,#31998));
#5966=EDGE_LOOP('',(#31999,#32000,#32001,#32002));
#5967=EDGE_LOOP('',(#32003,#32004,#32005,#32006,#32007,#32008,#32009,#32010,
#32011,#32012,#32013,#32014,#32015,#32016,#32017,#32018,#32019,#32020,#32021,
#32022,#32023,#32024));
#5968=EDGE_LOOP('',(#32025,#32026,#32027,#32028));
#5969=EDGE_LOOP('',(#32029,#32030,#32031,#32032));
#5970=EDGE_LOOP('',(#32033,#32034,#32035,#32036));
#5971=EDGE_LOOP('',(#32037,#32038,#32039,#32040));
#5972=EDGE_LOOP('',(#32041,#32042,#32043,#32044));
#5973=EDGE_LOOP('',(#32045,#32046,#32047,#32048));
#5974=EDGE_LOOP('',(#32049,#32050,#32051,#32052));
#5975=EDGE_LOOP('',(#32053,#32054,#32055,#32056,#32057,#32058));
#5976=EDGE_LOOP('',(#32059,#32060,#32061,#32062));
#5977=EDGE_LOOP('',(#32063,#32064,#32065,#32066));
#5978=EDGE_LOOP('',(#32067,#32068,#32069,#32070));
#5979=EDGE_LOOP('',(#32071,#32072,#32073,#32074,#32075,#32076,#32077,#32078,
#32079,#32080,#32081,#32082,#32083,#32084,#32085,#32086,#32087,#32088,#32089,
#32090,#32091,#32092));
#5980=EDGE_LOOP('',(#32093,#32094,#32095,#32096));
#5981=EDGE_LOOP('',(#32097,#32098,#32099,#32100));
#5982=EDGE_LOOP('',(#32101,#32102,#32103,#32104));
#5983=EDGE_LOOP('',(#32105,#32106,#32107,#32108));
#5984=EDGE_LOOP('',(#32109,#32110,#32111,#32112));
#5985=EDGE_LOOP('',(#32113,#32114,#32115,#32116));
#5986=EDGE_LOOP('',(#32117,#32118,#32119,#32120));
#5987=EDGE_LOOP('',(#32121,#32122,#32123,#32124));
#5988=EDGE_LOOP('',(#32125,#32126,#32127,#32128));
#5989=EDGE_LOOP('',(#32129,#32130,#32131,#32132));
#5990=EDGE_LOOP('',(#32133,#32134,#32135,#32136));
#5991=EDGE_LOOP('',(#32137,#32138,#32139,#32140,#32141,#32142,#32143));
#5992=EDGE_LOOP('',(#32144,#32145,#32146,#32147));
#5993=EDGE_LOOP('',(#32148,#32149,#32150,#32151,#32152,#32153,#32154));
#5994=EDGE_LOOP('',(#32155,#32156,#32157,#32158,#32159,#32160));
#5995=EDGE_LOOP('',(#32161,#32162,#32163,#32164));
#5996=EDGE_LOOP('',(#32165,#32166,#32167,#32168,#32169,#32170,#32171,#32172,
#32173,#32174,#32175,#32176,#32177,#32178,#32179,#32180,#32181,#32182,#32183,
#32184,#32185,#32186));
#5997=EDGE_LOOP('',(#32187,#32188,#32189,#32190));
#5998=EDGE_LOOP('',(#32191,#32192,#32193,#32194));
#5999=EDGE_LOOP('',(#32195,#32196,#32197,#32198));
#6000=EDGE_LOOP('',(#32199,#32200,#32201,#32202));
#6001=EDGE_LOOP('',(#32203,#32204,#32205,#32206));
#6002=EDGE_LOOP('',(#32207,#32208,#32209,#32210));
#6003=EDGE_LOOP('',(#32211,#32212,#32213,#32214));
#6004=EDGE_LOOP('',(#32215,#32216,#32217,#32218));
#6005=EDGE_LOOP('',(#32219,#32220,#32221,#32222));
#6006=EDGE_LOOP('',(#32223,#32224,#32225,#32226));
#6007=EDGE_LOOP('',(#32227,#32228,#32229,#32230));
#6008=EDGE_LOOP('',(#32231,#32232,#32233,#32234,#32235,#32236,#32237));
#6009=EDGE_LOOP('',(#32238,#32239,#32240,#32241));
#6010=EDGE_LOOP('',(#32242,#32243,#32244,#32245,#32246,#32247,#32248));
#6011=EDGE_LOOP('',(#32249,#32250,#32251,#32252,#32253,#32254));
#6012=EDGE_LOOP('',(#32255,#32256,#32257,#32258));
#6013=EDGE_LOOP('',(#32259,#32260,#32261,#32262,#32263,#32264,#32265,#32266,
#32267,#32268,#32269,#32270,#32271,#32272,#32273,#32274,#32275,#32276,#32277,
#32278,#32279,#32280));
#6014=EDGE_LOOP('',(#32281,#32282,#32283,#32284));
#6015=EDGE_LOOP('',(#32285,#32286,#32287,#32288));
#6016=EDGE_LOOP('',(#32289,#32290,#32291,#32292));
#6017=EDGE_LOOP('',(#32293,#32294,#32295,#32296));
#6018=EDGE_LOOP('',(#32297,#32298,#32299,#32300));
#6019=EDGE_LOOP('',(#32301,#32302,#32303,#32304));
#6020=EDGE_LOOP('',(#32305,#32306,#32307,#32308));
#6021=EDGE_LOOP('',(#32309,#32310,#32311,#32312));
#6022=EDGE_LOOP('',(#32313,#32314,#32315,#32316));
#6023=EDGE_LOOP('',(#32317,#32318,#32319,#32320));
#6024=EDGE_LOOP('',(#32321,#32322,#32323,#32324));
#6025=EDGE_LOOP('',(#32325,#32326,#32327,#32328,#32329,#32330,#32331));
#6026=EDGE_LOOP('',(#32332,#32333,#32334,#32335));
#6027=EDGE_LOOP('',(#32336,#32337,#32338,#32339,#32340,#32341,#32342));
#6028=EDGE_LOOP('',(#32343,#32344,#32345,#32346,#32347,#32348));
#6029=EDGE_LOOP('',(#32349,#32350,#32351,#32352));
#6030=EDGE_LOOP('',(#32353,#32354,#32355,#32356,#32357,#32358,#32359,#32360,
#32361,#32362,#32363,#32364,#32365,#32366,#32367,#32368,#32369,#32370,#32371,
#32372,#32373,#32374));
#6031=EDGE_LOOP('',(#32375,#32376,#32377,#32378));
#6032=EDGE_LOOP('',(#32379,#32380,#32381,#32382));
#6033=EDGE_LOOP('',(#32383,#32384,#32385,#32386));
#6034=EDGE_LOOP('',(#32387,#32388,#32389,#32390));
#6035=EDGE_LOOP('',(#32391,#32392,#32393,#32394));
#6036=EDGE_LOOP('',(#32395,#32396,#32397,#32398));
#6037=EDGE_LOOP('',(#32399,#32400,#32401,#32402));
#6038=EDGE_LOOP('',(#32403,#32404,#32405,#32406));
#6039=EDGE_LOOP('',(#32407,#32408,#32409,#32410));
#6040=EDGE_LOOP('',(#32411,#32412,#32413,#32414));
#6041=EDGE_LOOP('',(#32415,#32416,#32417,#32418));
#6042=EDGE_LOOP('',(#32419,#32420,#32421,#32422,#32423,#32424,#32425));
#6043=EDGE_LOOP('',(#32426,#32427,#32428,#32429));
#6044=EDGE_LOOP('',(#32430,#32431,#32432,#32433,#32434,#32435,#32436));
#6045=EDGE_LOOP('',(#32437,#32438,#32439,#32440,#32441,#32442));
#6046=EDGE_LOOP('',(#32443,#32444,#32445,#32446));
#6047=EDGE_LOOP('',(#32447,#32448,#32449,#32450,#32451,#32452,#32453,#32454,
#32455,#32456,#32457,#32458,#32459,#32460,#32461,#32462,#32463,#32464,#32465,
#32466,#32467,#32468));
#6048=EDGE_LOOP('',(#32469,#32470,#32471,#32472));
#6049=EDGE_LOOP('',(#32473,#32474,#32475,#32476));
#6050=EDGE_LOOP('',(#32477,#32478,#32479,#32480));
#6051=EDGE_LOOP('',(#32481,#32482,#32483,#32484));
#6052=EDGE_LOOP('',(#32485,#32486,#32487,#32488));
#6053=EDGE_LOOP('',(#32489,#32490,#32491,#32492));
#6054=EDGE_LOOP('',(#32493,#32494,#32495,#32496));
#6055=EDGE_LOOP('',(#32497,#32498,#32499));
#6056=EDGE_LOOP('',(#32500,#32501,#32502));
#6057=EDGE_LOOP('',(#32503,#32504,#32505,#32506));
#6058=EDGE_LOOP('',(#32507,#32508,#32509,#32510,#32511));
#6059=EDGE_LOOP('',(#32512,#32513,#32514,#32515,#32516,#32517,#32518,#32519));
#6060=EDGE_LOOP('',(#32520,#32521,#32522,#32523));
#6061=EDGE_LOOP('',(#32524,#32525,#32526));
#6062=EDGE_LOOP('',(#32527,#32528,#32529));
#6063=EDGE_LOOP('',(#32530,#32531,#32532,#32533,#32534));
#6064=EDGE_LOOP('',(#32535,#32536,#32537,#32538));
#6065=EDGE_LOOP('',(#32539,#32540,#32541,#32542));
#6066=EDGE_LOOP('',(#32543,#32544,#32545));
#6067=EDGE_LOOP('',(#32546,#32547,#32548,#32549));
#6068=EDGE_LOOP('',(#32550,#32551,#32552,#32553,#32554));
#6069=EDGE_LOOP('',(#32555,#32556,#32557));
#6070=EDGE_LOOP('',(#32558,#32559,#32560,#32561));
#6071=EDGE_LOOP('',(#32562,#32563,#32564,#32565,#32566));
#6072=EDGE_LOOP('',(#32567,#32568,#32569,#32570));
#6073=EDGE_LOOP('',(#32571,#32572,#32573,#32574,#32575,#32576,#32577,#32578));
#6074=EDGE_LOOP('',(#32579,#32580,#32581,#32582));
#6075=EDGE_LOOP('',(#32583,#32584,#32585));
#6076=EDGE_LOOP('',(#32586,#32587,#32588,#32589,#32590));
#6077=EDGE_LOOP('',(#32591,#32592,#32593));
#6078=EDGE_LOOP('',(#32594,#32595,#32596));
#6079=EDGE_LOOP('',(#32597,#32598,#32599,#32600));
#6080=EDGE_LOOP('',(#32601,#32602,#32603,#32604,#32605));
#6081=EDGE_LOOP('',(#32606,#32607,#32608,#32609,#32610,#32611,#32612,#32613));
#6082=EDGE_LOOP('',(#32614,#32615,#32616,#32617));
#6083=EDGE_LOOP('',(#32618,#32619,#32620,#32621));
#6084=EDGE_LOOP('',(#32622,#32623,#32624));
#6085=EDGE_LOOP('',(#32625,#32626,#32627));
#6086=EDGE_LOOP('',(#32628,#32629,#32630,#32631,#32632));
#6087=EDGE_LOOP('',(#32633,#32634,#32635,#32636));
#6088=EDGE_LOOP('',(#32637,#32638,#32639,#32640,#32641,#32642));
#6089=EDGE_LOOP('',(#32643,#32644,#32645,#32646));
#6090=EDGE_LOOP('',(#32647,#32648,#32649,#32650));
#6091=EDGE_LOOP('',(#32651,#32652,#32653));
#6092=EDGE_LOOP('',(#32654,#32655,#32656,#32657,#32658));
#6093=EDGE_LOOP('',(#32659,#32660,#32661,#32662,#32663,#32664,#32665,#32666));
#6094=EDGE_LOOP('',(#32667,#32668,#32669));
#6095=EDGE_LOOP('',(#32670,#32671,#32672,#32673,#32674));
#6096=EDGE_LOOP('',(#32675,#32676,#32677));
#6097=EDGE_LOOP('',(#32678,#32679,#32680,#32681));
#6098=EDGE_LOOP('',(#32682,#32683,#32684));
#6099=EDGE_LOOP('',(#32685,#32686,#32687,#32688));
#6100=EDGE_LOOP('',(#32689,#32690,#32691,#32692,#32693));
#6101=EDGE_LOOP('',(#32694,#32695,#32696,#32697));
#6102=EDGE_LOOP('',(#32698,#32699,#32700,#32701));
#6103=EDGE_LOOP('',(#32702,#32703,#32704));
#6104=EDGE_LOOP('',(#32705,#32706,#32707,#32708,#32709));
#6105=EDGE_LOOP('',(#32710,#32711,#32712,#32713,#32714,#32715,#32716));
#6106=EDGE_LOOP('',(#32717,#32718,#32719,#32720,#32721));
#6107=EDGE_LOOP('',(#32722,#32723,#32724,#32725,#32726,#32727,#32728,#32729));
#6108=EDGE_LOOP('',(#32730,#32731,#32732,#32733,#32734,#32735));
#6109=EDGE_LOOP('',(#32736,#32737,#32738));
#6110=EDGE_LOOP('',(#32739,#32740,#32741,#32742,#32743,#32744,#32745));
#6111=EDGE_LOOP('',(#32746,#32747,#32748,#32749));
#6112=EDGE_LOOP('',(#32750,#32751,#32752,#32753,#32754));
#6113=EDGE_LOOP('',(#32755,#32756,#32757,#32758));
#6114=EDGE_LOOP('',(#32759,#32760,#32761));
#6115=EDGE_LOOP('',(#32762,#32763,#32764,#32765,#32766));
#6116=EDGE_LOOP('',(#32767,#32768,#32769,#32770,#32771));
#6117=EDGE_LOOP('',(#32772,#32773,#32774,#32775));
#6118=EDGE_LOOP('',(#32776,#32777,#32778,#32779,#32780));
#6119=EDGE_LOOP('',(#32781,#32782,#32783,#32784,#32785,#32786,#32787,#32788));
#6120=EDGE_LOOP('',(#32789,#32790,#32791,#32792));
#6121=EDGE_LOOP('',(#32793,#32794,#32795,#32796,#32797,#32798));
#6122=EDGE_LOOP('',(#32799,#32800,#32801,#32802));
#6123=EDGE_LOOP('',(#32803,#32804,#32805,#32806,#32807,#32808));
#6124=EDGE_LOOP('',(#32809,#32810,#32811,#32812,#32813,#32814,#32815,#32816));
#6125=EDGE_LOOP('',(#32817,#32818,#32819,#32820));
#6126=EDGE_LOOP('',(#32821,#32822,#32823,#32824));
#6127=EDGE_LOOP('',(#32825,#32826,#32827,#32828));
#6128=EDGE_LOOP('',(#32829,#32830,#32831,#32832));
#6129=EDGE_LOOP('',(#32833,#32834,#32835,#32836));
#6130=EDGE_LOOP('',(#32837,#32838,#32839,#32840));
#6131=EDGE_LOOP('',(#32841,#32842,#32843,#32844));
#6132=EDGE_LOOP('',(#32845,#32846,#32847,#32848,#32849));
#6133=EDGE_LOOP('',(#32850,#32851,#32852,#32853));
#6134=EDGE_LOOP('',(#32854,#32855,#32856,#32857));
#6135=EDGE_LOOP('',(#32858,#32859,#32860,#32861));
#6136=EDGE_LOOP('',(#32862,#32863,#32864,#32865));
#6137=EDGE_LOOP('',(#32866,#32867,#32868,#32869));
#6138=EDGE_LOOP('',(#32870,#32871,#32872,#32873,#32874));
#6139=EDGE_LOOP('',(#32875,#32876,#32877,#32878));
#6140=EDGE_LOOP('',(#32879,#32880,#32881,#32882));
#6141=EDGE_LOOP('',(#32883,#32884,#32885,#32886));
#6142=EDGE_LOOP('',(#32887,#32888,#32889,#32890,#32891));
#6143=EDGE_LOOP('',(#32892,#32893,#32894,#32895));
#6144=EDGE_LOOP('',(#32896,#32897,#32898,#32899));
#6145=EDGE_LOOP('',(#32900,#32901,#32902,#32903));
#6146=EDGE_LOOP('',(#32904,#32905,#32906,#32907));
#6147=EDGE_LOOP('',(#32908,#32909,#32910,#32911));
#6148=EDGE_LOOP('',(#32912,#32913,#32914,#32915,#32916));
#6149=EDGE_LOOP('',(#32917,#32918,#32919,#32920));
#6150=EDGE_LOOP('',(#32921,#32922,#32923,#32924));
#6151=EDGE_LOOP('',(#32925,#32926,#32927,#32928));
#6152=EDGE_LOOP('',(#32929,#32930,#32931,#32932));
#6153=EDGE_LOOP('',(#32933,#32934,#32935,#32936));
#6154=EDGE_LOOP('',(#32937,#32938,#32939,#32940));
#6155=EDGE_LOOP('',(#32941,#32942,#32943,#32944));
#6156=EDGE_LOOP('',(#32945,#32946,#32947,#32948));
#6157=EDGE_LOOP('',(#32949,#32950,#32951,#32952,#32953));
#6158=EDGE_LOOP('',(#32954,#32955,#32956,#32957));
#6159=EDGE_LOOP('',(#32958,#32959,#32960,#32961));
#6160=EDGE_LOOP('',(#32962,#32963,#32964,#32965));
#6161=EDGE_LOOP('',(#32966,#32967,#32968,#32969,#32970));
#6162=EDGE_LOOP('',(#32971,#32972,#32973,#32974));
#6163=EDGE_LOOP('',(#32975,#32976,#32977,#32978));
#6164=EDGE_LOOP('',(#32979,#32980,#32981,#32982));
#6165=EDGE_LOOP('',(#32983,#32984,#32985,#32986));
#6166=EDGE_LOOP('',(#32987,#32988,#32989,#32990));
#6167=EDGE_LOOP('',(#32991,#32992,#32993,#32994,#32995));
#6168=EDGE_LOOP('',(#32996,#32997,#32998,#32999));
#6169=EDGE_LOOP('',(#33000,#33001,#33002,#33003));
#6170=EDGE_LOOP('',(#33004,#33005,#33006,#33007));
#6171=EDGE_LOOP('',(#33008,#33009,#33010,#33011,#33012));
#6172=EDGE_LOOP('',(#33013,#33014,#33015,#33016));
#6173=EDGE_LOOP('',(#33017,#33018,#33019,#33020));
#6174=EDGE_LOOP('',(#33021,#33022,#33023,#33024));
#6175=EDGE_LOOP('',(#33025,#33026,#33027,#33028));
#6176=EDGE_LOOP('',(#33029,#33030,#33031,#33032,#33033,#33034,#33035));
#6177=EDGE_LOOP('',(#33036,#33037,#33038,#33039,#33040,#33041,#33042));
#6178=EDGE_LOOP('',(#33043,#33044,#33045,#33046,#33047));
#6179=EDGE_LOOP('',(#33048,#33049,#33050,#33051));
#6180=EDGE_LOOP('',(#33052,#33053,#33054,#33055));
#6181=EDGE_LOOP('',(#33056,#33057,#33058,#33059));
#6182=EDGE_LOOP('',(#33060,#33061,#33062,#33063));
#6183=EDGE_LOOP('',(#33064,#33065,#33066,#33067));
#6184=EDGE_LOOP('',(#33068,#33069,#33070,#33071));
#6185=EDGE_LOOP('',(#33072,#33073,#33074,#33075));
#6186=EDGE_LOOP('',(#33076,#33077,#33078,#33079,#33080));
#6187=EDGE_LOOP('',(#33081,#33082,#33083,#33084,#33085,#33086,#33087));
#6188=EDGE_LOOP('',(#33088,#33089,#33090,#33091));
#6189=EDGE_LOOP('',(#33092,#33093,#33094,#33095,#33096,#33097,#33098));
#8393=CIRCLE('',#43277,0.4);
#8394=CIRCLE('',#43278,0.4);
#8395=CIRCLE('',#43280,0.4);
#8396=CIRCLE('',#43283,0.4);
#8397=CIRCLE('',#43285,0.4);
#8398=CIRCLE('',#43286,0.4);
#8399=CIRCLE('',#43289,20.899760764181);
#8400=CIRCLE('',#43290,20.899760764181);
#8401=CIRCLE('',#43291,20.899760764181);
#8402=CIRCLE('',#43292,20.899760764181);
#8403=CIRCLE('',#43293,20.899760764181);
#8404=CIRCLE('',#43294,20.899760764181);
#8405=CIRCLE('',#43295,12.);
#8406=CIRCLE('',#43296,0.4);
#8407=CIRCLE('',#43297,12.);
#8408=CIRCLE('',#43298,0.4);
#8409=CIRCLE('',#43299,0.4);
#8410=CIRCLE('',#43300,12.);
#8411=CIRCLE('',#43301,0.4);
#8412=CIRCLE('',#43302,0.4);
#8413=CIRCLE('',#43303,12.);
#8414=CIRCLE('',#43304,0.4);
#8415=CIRCLE('',#43305,0.4);
#8416=CIRCLE('',#43306,12.);
#8417=CIRCLE('',#43307,0.4);
#8418=CIRCLE('',#43308,0.4);
#8419=CIRCLE('',#43309,12.);
#8420=CIRCLE('',#43310,0.4);
#8421=CIRCLE('',#43311,0.4);
#8422=CIRCLE('',#43312,12.);
#8423=CIRCLE('',#43313,0.4);
#8424=CIRCLE('',#43314,0.4);
#8425=CIRCLE('',#43315,12.);
#8426=CIRCLE('',#43316,0.4);
#8427=CIRCLE('',#43317,0.4);
#8428=CIRCLE('',#43318,12.);
#8429=CIRCLE('',#43319,0.4);
#8430=CIRCLE('',#43320,0.4);
#8431=CIRCLE('',#43321,12.);
#8432=CIRCLE('',#43322,0.4);
#8433=CIRCLE('',#43323,0.4);
#8434=CIRCLE('',#43324,12.);
#8435=CIRCLE('',#43325,0.4);
#8436=CIRCLE('',#43326,0.4);
#8437=CIRCLE('',#43327,12.);
#8438=CIRCLE('',#43328,0.4);
#8439=CIRCLE('',#43329,0.4);
#8440=CIRCLE('',#43330,12.);
#8441=CIRCLE('',#43331,0.4);
#8442=CIRCLE('',#43332,0.4);
#8443=CIRCLE('',#43333,12.);
#8444=CIRCLE('',#43334,0.4);
#8445=CIRCLE('',#43335,0.4);
#8446=CIRCLE('',#43336,12.);
#8447=CIRCLE('',#43337,0.4);
#8448=CIRCLE('',#43338,0.4);
#8449=CIRCLE('',#43339,12.);
#8450=CIRCLE('',#43340,0.4);
#8451=CIRCLE('',#43341,0.4);
#8452=CIRCLE('',#43342,12.);
#8453=CIRCLE('',#43343,0.4);
#8454=CIRCLE('',#43344,0.4);
#8455=CIRCLE('',#43345,12.);
#8456=CIRCLE('',#43346,0.4);
#8457=CIRCLE('',#43347,0.4);
#8458=CIRCLE('',#43348,12.);
#8459=CIRCLE('',#43349,0.4);
#8460=CIRCLE('',#43350,0.4);
#8461=CIRCLE('',#43351,12.);
#8462=CIRCLE('',#43352,0.4);
#8463=CIRCLE('',#43353,0.4);
#8464=CIRCLE('',#43354,12.);
#8465=CIRCLE('',#43355,0.4);
#8466=CIRCLE('',#43356,0.4);
#8467=CIRCLE('',#43357,12.);
#8468=CIRCLE('',#43358,0.4);
#8469=CIRCLE('',#43359,0.4);
#8470=CIRCLE('',#43360,12.);
#8471=CIRCLE('',#43361,0.4);
#8472=CIRCLE('',#43362,0.4);
#8473=CIRCLE('',#43363,12.);
#8474=CIRCLE('',#43365,0.4);
#8475=CIRCLE('',#43368,12.);
#8476=CIRCLE('',#43369,20.899760764181);
#8477=CIRCLE('',#43370,12.);
#8478=CIRCLE('',#43371,0.4);
#8479=CIRCLE('',#43372,0.4);
#8480=CIRCLE('',#43373,12.);
#8481=CIRCLE('',#43374,0.4);
#8482=CIRCLE('',#43375,0.4);
#8483=CIRCLE('',#43376,12.);
#8484=CIRCLE('',#43384,0.4);
#8485=CIRCLE('',#43386,0.4);
#8486=CIRCLE('',#43390,0.4);
#8487=CIRCLE('',#43392,0.4);
#8488=CIRCLE('',#43393,12.);
#8489=CIRCLE('',#43394,20.899760764181);
#8490=CIRCLE('',#43395,12.);
#8491=CIRCLE('',#43396,0.4);
#8492=CIRCLE('',#43397,0.4);
#8493=CIRCLE('',#43398,12.);
#8494=CIRCLE('',#43399,0.4);
#8495=CIRCLE('',#43400,0.4);
#8496=CIRCLE('',#43401,12.);
#8497=CIRCLE('',#43413,0.4);
#8498=CIRCLE('',#43415,18.4568971235747);
#8499=CIRCLE('',#43417,0.4);
#8500=CIRCLE('',#43419,18.4568971235747);
#8501=CIRCLE('',#43422,0.4);
#8502=CIRCLE('',#43424,0.4);
#8503=CIRCLE('',#43425,12.);
#8504=CIRCLE('',#43426,20.899760764181);
#8505=CIRCLE('',#43427,12.);
#8506=CIRCLE('',#43428,0.4);
#8507=CIRCLE('',#43429,0.4);
#8508=CIRCLE('',#43430,12.);
#8509=CIRCLE('',#43431,0.4);
#8510=CIRCLE('',#43432,0.4);
#8511=CIRCLE('',#43433,12.);
#8512=CIRCLE('',#43445,0.4);
#8513=CIRCLE('',#43447,18.4568971235747);
#8514=CIRCLE('',#43449,0.4);
#8515=CIRCLE('',#43451,18.4568971235747);
#8516=CIRCLE('',#43454,0.4);
#8517=CIRCLE('',#43456,0.4);
#8518=CIRCLE('',#43457,12.);
#8519=CIRCLE('',#43458,20.899760764181);
#8520=CIRCLE('',#43459,12.);
#8521=CIRCLE('',#43460,0.4);
#8522=CIRCLE('',#43461,0.4);
#8523=CIRCLE('',#43462,12.);
#8524=CIRCLE('',#43463,0.4);
#8525=CIRCLE('',#43464,0.4);
#8526=CIRCLE('',#43465,12.);
#8527=CIRCLE('',#43477,0.4);
#8528=CIRCLE('',#43479,18.4568971235747);
#8529=CIRCLE('',#43481,0.4);
#8530=CIRCLE('',#43483,18.4568971235747);
#8531=CIRCLE('',#43486,0.4);
#8532=CIRCLE('',#43488,0.4);
#8533=CIRCLE('',#43489,12.);
#8534=CIRCLE('',#43490,20.899760764181);
#8535=CIRCLE('',#43491,12.);
#8536=CIRCLE('',#43492,0.4);
#8537=CIRCLE('',#43493,0.4);
#8538=CIRCLE('',#43494,12.);
#8539=CIRCLE('',#43495,0.4);
#8540=CIRCLE('',#43496,0.4);
#8541=CIRCLE('',#43497,12.);
#8542=CIRCLE('',#43509,0.4);
#8543=CIRCLE('',#43511,18.4568971235747);
#8544=CIRCLE('',#43513,0.4);
#8545=CIRCLE('',#43515,18.4568971235747);
#8546=CIRCLE('',#43518,0.4);
#8547=CIRCLE('',#43520,0.4);
#8548=CIRCLE('',#43521,12.);
#8549=CIRCLE('',#43522,20.899760764181);
#8550=CIRCLE('',#43523,12.);
#8551=CIRCLE('',#43524,0.4);
#8552=CIRCLE('',#43525,0.4);
#8553=CIRCLE('',#43526,12.);
#8554=CIRCLE('',#43527,0.4);
#8555=CIRCLE('',#43528,0.4);
#8556=CIRCLE('',#43529,12.);
#8557=CIRCLE('',#43536,0.399999999999998);
#8558=CIRCLE('',#43537,0.400000000004375);
#8559=CIRCLE('',#43539,0.4);
#8560=CIRCLE('',#43540,0.399999999999995);
#8561=CIRCLE('',#43542,0.400000000000001);
#8562=CIRCLE('',#43543,0.4);
#8563=CIRCLE('',#43545,0.399999999999991);
#8564=CIRCLE('',#43546,21.2696680343435);
#8565=CIRCLE('',#43548,18.4568971235747);
#8566=CIRCLE('',#43549,18.4568971235747);
#8567=CIRCLE('',#43550,0.399999999999998);
#8568=CIRCLE('',#43551,0.40000000000001);
#8569=CIRCLE('',#43553,0.4);
#8570=CIRCLE('',#43554,0.399999999999997);
#8571=CIRCLE('',#43556,0.400000000000002);
#8572=CIRCLE('',#43557,0.4);
#8573=CIRCLE('',#43559,21.2696680343435);
#8574=CIRCLE('',#43560,0.4);
#8575=CIRCLE('',#43562,21.2696680343435);
#8576=CIRCLE('',#43564,0.399999999999996);
#8577=CIRCLE('',#43565,0.4);
#8578=CIRCLE('',#43567,21.2696680343435);
#8579=CIRCLE('',#43568,0.399999999999999);
#8580=CIRCLE('',#43570,0.399999999999999);
#8581=CIRCLE('',#43571,0.4);
#8582=CIRCLE('',#43572,0.399999999999999);
#8583=CIRCLE('',#43574,21.2696680343435);
#8584=CIRCLE('',#43575,21.2696680343435);
#8585=CIRCLE('',#43576,0.400000000000009);
#8586=CIRCLE('',#43577,0.400000000000003);
#8587=CIRCLE('',#43579,0.399999999999998);
#8588=CIRCLE('',#43580,0.399999999999998);
#8589=CIRCLE('',#43582,0.399999999999999);
#8590=CIRCLE('',#43583,0.4);
#8591=CIRCLE('',#43585,0.399999999999991);
#8592=CIRCLE('',#43586,21.2696680343435);
#8593=CIRCLE('',#43587,21.2696680343435);
#8594=CIRCLE('',#43588,0.400000000000002);
#8595=CIRCLE('',#43590,0.399999999999999);
#8596=CIRCLE('',#43592,0.399999999999999);
#8597=CIRCLE('',#43594,0.399999999999993);
#8598=CIRCLE('',#43595,21.2696680343435);
#8599=CIRCLE('',#43597,0.4);
#8600=CIRCLE('',#43598,0.399999999999998);
#8601=CIRCLE('',#43599,0.400000000000004);
#8602=CIRCLE('',#43601,0.4);
#8603=CIRCLE('',#43602,0.399999999999994);
#8604=CIRCLE('',#43604,0.4);
#8605=CIRCLE('',#43606,21.2696680343435);
#8606=CIRCLE('',#43608,21.2696680343435);
#8607=CIRCLE('',#43611,0.399999999999991);
#8608=CIRCLE('',#43613,0.4);
#8609=CIRCLE('',#43614,0.400000000000003);
#8610=CIRCLE('',#43617,0.399999999999991);
#8611=CIRCLE('',#43618,0.400000000000003);
#8612=CIRCLE('',#43620,0.399999999999993);
#8613=CIRCLE('',#43621,0.399999999999997);
#8614=CIRCLE('',#43622,0.399999999999998);
#8615=CIRCLE('',#43624,21.2696680343435);
#8616=CIRCLE('',#43626,0.4);
#8617=CIRCLE('',#43627,0.400000000000001);
#8618=CIRCLE('',#43628,0.399999999999999);
#8619=CIRCLE('',#43630,0.399999999999999);
#8620=CIRCLE('',#43633,23.);
#8621=CIRCLE('',#43636,0.399999999999996);
#8622=CIRCLE('',#43637,0.399999999999998);
#8623=CIRCLE('',#43639,23.);
#8624=CIRCLE('',#43640,0.399999999999994);
#8625=CIRCLE('',#43642,0.399999999999999);
#8626=CIRCLE('',#43643,0.4);
#8627=CIRCLE('',#43646,21.2696680343435);
#8628=CIRCLE('',#43648,18.4568971235747);
#8629=CIRCLE('',#43649,18.4568971235747);
#8630=CIRCLE('',#43652,21.2696680343435);
#10135=B_SPLINE_CURVE_WITH_KNOTS('',3,(#78429,#78430,#78431,#78432,#78433,
#78434),.UNSPECIFIED.,.F.,.F.,(4,1,1,4),(-1.58311731128069,-1.23079794741793,
-0.852705185028571,-0.285566041444528),.UNSPECIFIED.);
#10136=B_SPLINE_CURVE_WITH_KNOTS('',3,(#78438,#78439,#78440,#78441,#78442,
#78443),.UNSPECIFIED.,.F.,.F.,(4,1,1,4),(-2.06216197549039,-1.68406976842606,
-1.30597756136174,-0.764611866701079),.UNSPECIFIED.);
#10137=B_SPLINE_CURVE_WITH_KNOTS('',3,(#78447,#78448,#78449,#78450,#78451,
#78452),.UNSPECIFIED.,.F.,.F.,(4,1,1,4),(-1.56141606155233,-1.19068669470827,
-0.819957327864215,-0.263863277598129),.UNSPECIFIED.);
#10138=B_SPLINE_CURVE_WITH_KNOTS('',3,(#78456,#78457,#78458,#78459,#78460,
#78461),.UNSPECIFIED.,.F.,.F.,(4,1,1,4),(-1.58311823332826,-1.04175156622325,
-0.663658803833889,-0.285566041444524),.UNSPECIFIED.);
#10139=B_SPLINE_CURVE_WITH_KNOTS('',3,(#78465,#78466,#78467,#78468,#78469,
#78470),.UNSPECIFIED.,.F.,.F.,(4,1,1,4),(-2.06216401280017,-1.69143464595466,
-1.32070527910915,-0.764611228840875),.UNSPECIFIED.);
#10140=B_SPLINE_CURVE_WITH_KNOTS('',3,(#78473,#78474,#78475,#78476,#78477,
#78478),.UNSPECIFIED.,.F.,.F.,(4,1,1,4),(-1.56141606155233,-1.19068669470806,
-0.819957327863798,-0.263863277597402),.UNSPECIFIED.);
#10141=B_SPLINE_CURVE_WITH_KNOTS('',3,(#78769,#78770,#78771,#78772,#78773,
#78774),.UNSPECIFIED.,.F.,.F.,(4,1,1,4),(-2.63928284000037,-2.0140383913787,
-1.70141616706786,-1.58720231920435),.UNSPECIFIED.);
#10142=B_SPLINE_CURVE_WITH_KNOTS('',3,(#78778,#78779,#78780,#78781,#78782,
#78783),.UNSPECIFIED.,.F.,.F.,(4,1,1,4),(-2.17034568593159,-1.89991708323787,
-1.58729550831966,-1.11836314594235),.UNSPECIFIED.);
#10143=B_SPLINE_CURVE_WITH_KNOTS('',3,(#78860,#78861,#78862,#78863,#78864,
#78865),.UNSPECIFIED.,.F.,.F.,(4,1,1,4),(-2.47569718960832,-1.85045379098313,
-1.53783209167054,-1.42361855687056),.UNSPECIFIED.);
#10144=B_SPLINE_CURVE_WITH_KNOTS('',3,(#78869,#78870,#78871,#78872,#78873,
#78874),.UNSPECIFIED.,.F.,.F.,(4,1,1,4),(-1.284775479628,-1.01434327886057,
-0.858032407070129,-0.232788919908364),.UNSPECIFIED.);
#10145=B_SPLINE_CURVE_WITH_KNOTS('',3,(#78936,#78937,#78938,#78939,#78940,
#78941,#78942,#78943,#78944,#78945,#78946,#78947,#78948),.UNSPECIFIED.,
 .F.,.F.,(4,3,3,3,4),(0.0105027337450474,0.0145912333590045,0.0213180081986026,
0.0280164960752336,0.0291731591110207),.UNSPECIFIED.);
#10146=B_SPLINE_CURVE_WITH_KNOTS('',3,(#78968,#78969,#78970,#78971,#78972,
#78973,#78974,#78975,#78976,#78977,#78978,#78979,#78980),.UNSPECIFIED.,
 .F.,.F.,(4,3,3,3,4),(0.,0.00668972973726014,0.0134212533757443,0.0145801248518802,
0.0186681351907681),.UNSPECIFIED.);
#10147=B_SPLINE_CURVE_WITH_KNOTS('',3,(#79001,#79002,#79003,#79004,#79005,
#79006),.UNSPECIFIED.,.F.,.F.,(4,1,1,4),(-2.56413746035908,-2.09520509798177,
-1.78258352306356,-1.51215492036984),.UNSPECIFIED.);
#10148=B_SPLINE_CURVE_WITH_KNOTS('',3,(#79010,#79011,#79012,#79013,#79014,
#79015),.UNSPECIFIED.,.F.,.F.,(4,1,1,4),(-1.3599071057515,-1.07634287797832,
-0.750578938128915,-0.307931612733822),.UNSPECIFIED.);
#10149=B_SPLINE_CURVE_WITH_KNOTS('',3,(#79077,#79078,#79079,#79080,#79081,
#79082,#79083,#79084,#79085,#79086,#79087,#79088,#79089),.UNSPECIFIED.,
 .F.,.F.,(4,3,3,3,4),(0.0104839491302103,0.0145705936737829,0.0194264046381681,
0.026158009214639,0.0291307560165951),.UNSPECIFIED.);
#10150=B_SPLINE_CURVE_WITH_KNOTS('',3,(#79109,#79110,#79111,#79112,#79113,
#79114,#79115,#79116,#79117,#79118,#79119,#79120,#79121),.UNSPECIFIED.,
 .F.,.F.,(4,3,3,3,4),(0.,0.00668973417377084,0.0134212540675091,0.0145801130032157,
0.0186681351443382),.UNSPECIFIED.);
#10151=B_SPLINE_CURVE_WITH_KNOTS('',3,(#79142,#79143,#79144,#79145,#79146,
#79147),.UNSPECIFIED.,.F.,.F.,(4,1,1,4),(-2.38794895474362,-1.91901561826703,
-1.60639339394931,-1.33596409609193),.UNSPECIFIED.);
#10152=B_SPLINE_CURVE_WITH_KNOTS('',3,(#79151,#79152,#79153,#79154,#79155,
#79156),.UNSPECIFIED.,.F.,.F.,(4,1,1,4),(-2.17034568593159,-1.89991708323787,
-1.58729550831966,-1.11836314594235),.UNSPECIFIED.);
#10153=B_SPLINE_CURVE_WITH_KNOTS('',3,(#79218,#79219,#79220,#79221,#79222,
#79223,#79224,#79225,#79226,#79227,#79228,#79229,#79230),.UNSPECIFIED.,
 .F.,.F.,(4,3,3,3,4),(0.0105027337450297,0.0145912333589661,0.0213179561731519,
0.0280163477738522,0.0291731591109597),.UNSPECIFIED.);
#10154=B_SPLINE_CURVE_WITH_KNOTS('',3,(#79250,#79251,#79252,#79253,#79254,
#79255,#79256,#79257,#79258,#79259,#79260,#79261,#79262),.UNSPECIFIED.,
 .F.,.F.,(4,3,3,3,4),(0.,0.00668995938833792,0.0134216137859652,0.0145801214848642,
0.0186681351775866),.UNSPECIFIED.);
#10155=B_SPLINE_CURVE_WITH_KNOTS('',3,(#79283,#79284,#79285,#79286,#79287,
#79288),.UNSPECIFIED.,.F.,.F.,(4,1,1,4),(-2.47568817722038,-1.85044749661957,
-1.53782715631916,-1.42361433373037),.UNSPECIFIED.);
#10156=B_SPLINE_CURVE_WITH_KNOTS('',3,(#79292,#79293,#79294,#79295,#79296,
#79297),.UNSPECIFIED.,.F.,.F.,(4,1,1,4),(-1.2847655540421,-1.01433852921875,
-0.70171854409386,-0.232788566406526),.UNSPECIFIED.);
#10157=B_SPLINE_CURVE_WITH_KNOTS('',3,(#79359,#79360,#79361,#79362,#79363,
#79364,#79365,#79366,#79367,#79368,#79369,#79370,#79371),.UNSPECIFIED.,
 .F.,.F.,(4,3,3,3,4),(0.0105027337276142,0.0145912289237958,0.0213179515980425,
0.0280163554588487,0.0291731591115961),.UNSPECIFIED.);
#10158=B_SPLINE_CURVE_WITH_KNOTS('',3,(#79391,#79392,#79393,#79394,#79395,
#79396,#79397,#79398,#79399,#79400,#79401,#79402,#79403),.UNSPECIFIED.,
 .F.,.F.,(4,3,3,3,4),(0.,0.00668980548898492,0.0134213909862664,0.0145801248518791,
0.0186681351907661),.UNSPECIFIED.);
#10159=B_SPLINE_CURVE_WITH_KNOTS('',3,(#79424,#79425,#79426,#79427,#79428,
#79429),.UNSPECIFIED.,.F.,.F.,(4,1,1,4),(-2.56415695446836,-1.95860539237294,
-1.79572424429708,-1.51215685703286),.UNSPECIFIED.);
#10160=B_SPLINE_CURVE_WITH_KNOTS('',3,(#79433,#79434,#79435,#79436,#79437,
#79438),.UNSPECIFIED.,.F.,.F.,(4,1,1,4),(-1.35990710575149,-1.07634287797832,
-0.750578938128917,-0.307931612733825),.UNSPECIFIED.);
#10161=B_SPLINE_CURVE_WITH_KNOTS('',3,(#79509,#79510,#79511,#79512,#79513),
 .UNSPECIFIED.,.F.,.F.,(4,1,4),(-1.78143848901605,-0.763473638149737,0.),
 .UNSPECIFIED.);
#10162=B_SPLINE_CURVE_WITH_KNOTS('',3,(#79516,#79517,#79518,#79519,#79520),
 .UNSPECIFIED.,.F.,.F.,(4,1,4),(0.,0.763473638149737,1.78143848901605),
 .UNSPECIFIED.);
#10163=B_SPLINE_CURVE_WITH_KNOTS('',3,(#79562,#79563,#79564,#79565,#79566,
#79567),.UNSPECIFIED.,.F.,.F.,(4,1,1,4),(0.285566041444528,0.852705185028571,
1.23079794741793,1.6088907098073),.UNSPECIFIED.);
#10164=B_SPLINE_CURVE_WITH_KNOTS('',3,(#79569,#79570,#79571,#79572,#79573,
#79574,#79575),.UNSPECIFIED.,.F.,.F.,(4,3,4),(0.,0.00663328573812816,0.0112828850428469),
 .UNSPECIFIED.);
#10165=B_SPLINE_CURVE_WITH_KNOTS('',3,(#79576,#79577,#79578,#79579,#79580,
#79581,#79582,#79583,#79584,#79585,#79586,#79587,#79588,#79589,#79590,#79591,
#79592,#79593,#79594,#79595,#79596,#79597,#79598,#79599,#79600,#79601,#79602,
#79603,#79604,#79605,#79606),.UNSPECIFIED.,.F.,.F.,(4,3,3,3,3,3,3,3,3,3,
4),(0.,0.00637154645979595,0.0131156955971514,0.0148241842185563,0.0193928616961542,
0.0261518983038848,0.0320292760531256,0.0394205065706234,0.0470086761742551,
0.0518402511587753,0.0521489961176007),.UNSPECIFIED.);
#10166=B_SPLINE_CURVE_WITH_KNOTS('',3,(#79609,#79610,#79611,#79612,#79613,
#79614),.UNSPECIFIED.,.F.,.F.,(4,1,1,4),(1.54728972325333,1.70141616706786,
2.0140383913787,2.63928284000037),.UNSPECIFIED.);
#10167=B_SPLINE_CURVE_WITH_KNOTS('',3,(#79618,#79619,#79620,#79621,#79622,
#79623),.UNSPECIFIED.,.F.,.F.,(4,2,4),(2.49842406090827,2.56616169967075,
2.63389933843322),.UNSPECIFIED.);
#10168=B_SPLINE_CURVE_WITH_KNOTS('',3,(#79627,#79628,#79629,#79630,#79631,
#79632),.UNSPECIFIED.,.F.,.F.,(4,1,1,4),(0.261933028354807,0.750578938128917,
1.07634287797832,1.39992181764611),.UNSPECIFIED.);
#10169=B_SPLINE_CURVE_WITH_KNOTS('',3,(#79633,#79634,#79635,#79636,#79637,
#79638,#79639,#79640,#79641,#79642,#79643,#79644),.UNSPECIFIED.,.F.,.F.,
(4,2,2,2,2,4),(19.4435968556707,19.7442925972667,20.064736080688,20.4210982332895,
20.7774603858911,21.1293548879221),.UNSPECIFIED.);
#10170=B_SPLINE_CURVE_WITH_KNOTS('',3,(#79674,#79675,#79676,#79677,#79678),
 .UNSPECIFIED.,.F.,.F.,(4,1,4),(-1.78143848901855,-0.763473638150805,0.),
 .UNSPECIFIED.);
#10171=B_SPLINE_CURVE_WITH_KNOTS('',3,(#79681,#79682,#79683,#79684,#79685),
 .UNSPECIFIED.,.F.,.F.,(4,1,4),(0.,0.763473638150805,1.78143848901855),
 .UNSPECIFIED.);
#10172=B_SPLINE_CURVE_WITH_KNOTS('',3,(#79722,#79723,#79724,#79725),
 .UNSPECIFIED.,.F.,.F.,(4,4),(0.,0.0418633800522656),.UNSPECIFIED.);
#10173=B_SPLINE_CURVE_WITH_KNOTS('',3,(#79726,#79727,#79728,#79729,#79730,
#79731),.UNSPECIFIED.,.F.,.F.,(4,1,1,4),(1.29595614936969,1.60639339394931,
1.91901561826703,2.38794895474362),.UNSPECIFIED.);
#10174=B_SPLINE_CURVE_WITH_KNOTS('',3,(#79739,#79740,#79741,#79742,#79743),
 .UNSPECIFIED.,.F.,.F.,(4,1,4),(-2.51469634683131,-1.49674691578015,-0.733284842491785),
 .UNSPECIFIED.);
#10175=B_SPLINE_CURVE_WITH_KNOTS('',3,(#79751,#79752,#79753,#79754,#79755,
#79756,#79757,#79758,#79759,#79760,#79761,#79762,#79763,#79764,#79765,#79766,
#79767,#79768,#79769,#79770,#79771,#79772,#79773,#79774,#79775,#79776,#79777,
#79778,#79779,#79780,#79781),.UNSPECIFIED.,.F.,.F.,(4,3,3,3,3,3,3,3,3,3,
4),(-0.0520947056315157,-0.0456917383750113,-0.0389151295335283,-0.0371977052785187,
-0.0326066524906523,-0.0258157677072658,-0.0199080821245583,-0.0124819132463451,
-0.00485717179978691,0.,0.000310267175257624),.UNSPECIFIED.);
#10176=B_SPLINE_CURVE_WITH_KNOTS('',3,(#79814,#79815,#79816,#79817,#79818,
#79819),.UNSPECIFIED.,.F.,.F.,(4,1,1,4),(0.738839250765249,1.30597756136174,
1.68406976842606,2.06216197549039),.UNSPECIFIED.);
#10177=B_SPLINE_CURVE_WITH_KNOTS('',3,(#79821,#79822,#79823,#79824,#79825,
#79826,#79827,#79828,#79829,#79830),.UNSPECIFIED.,.F.,.F.,(4,3,3,4),(0.0492862965832315,
0.0519911064607945,0.0586129067543968,0.0605552986795682),.UNSPECIFIED.);
#10178=B_SPLINE_CURVE_WITH_KNOTS('',3,(#79867,#79868,#79869,#79870,#79871,
#79872),.UNSPECIFIED.,.F.,.F.,(4,1,1,4),(0.263863277597402,0.819957327863798,
1.19068669470806,1.56141606155233),.UNSPECIFIED.);
#10179=B_SPLINE_CURVE_WITH_KNOTS('',3,(#79905,#79906,#79907,#79908,#79909),
 .UNSPECIFIED.,.F.,.F.,(4,1,4),(0.805732136131231,1.56919017940703,2.5871342371081),
 .UNSPECIFIED.);
#10180=B_SPLINE_CURVE_WITH_KNOTS('',3,(#79912,#79913,#79914,#79915,#79916),
 .UNSPECIFIED.,.F.,.F.,(4,1,4),(-2.5871342371081,-1.56919017940703,-0.805732136131231),
 .UNSPECIFIED.);
#10181=B_SPLINE_CURVE_WITH_KNOTS('',3,(#79919,#79920,#79921,#79922,#79923,
#79924,#79925,#79926,#79927,#79928,#79929,#79930),.UNSPECIFIED.,.F.,.F.,
(4,2,2,2,2,4),(14.0969491012437,14.4488436032748,14.8052057558763,15.1615679084779,
15.4820113918991,15.7827071334951),.UNSPECIFIED.);
#10182=B_SPLINE_CURVE_WITH_KNOTS('',3,(#79931,#79932,#79933,#79934,#79935,
#79936),.UNSPECIFIED.,.F.,.F.,(4,1,1,4),(1.47214692939812,1.79572424429708,
1.95860539237294,2.6101299846764),.UNSPECIFIED.);
#10183=B_SPLINE_CURVE_WITH_KNOTS('',3,(#79937,#79938,#79939,#79940,#79941,
#79942),.UNSPECIFIED.,.F.,.F.,(4,2,4),(2.49842406090827,2.56616169967075,
2.63389933843322),.UNSPECIFIED.);
#10184=B_SPLINE_CURVE_WITH_KNOTS('',3,(#79943,#79944,#79945,#79946,#79947,
#79948),.UNSPECIFIED.,.F.,.F.,(4,1,1,4),(0.232788566406526,0.70171854409386,
1.01433852921875,1.32477353114902),.UNSPECIFIED.);
#10185=B_SPLINE_CURVE_WITH_KNOTS('',3,(#79978,#79979,#79980,#79981,#79982),
 .UNSPECIFIED.,.F.,.F.,(4,1,4),(-1.78143818604478,-0.763473508304906,0.),
 .UNSPECIFIED.);
#10186=B_SPLINE_CURVE_WITH_KNOTS('',3,(#79985,#79986,#79987,#79988,#79989),
 .UNSPECIFIED.,.F.,.F.,(4,1,4),(0.,0.763473508304906,1.78143818604478),
 .UNSPECIFIED.);
#10187=B_SPLINE_CURVE_WITH_KNOTS('',3,(#80038,#80039,#80040,#80041,#80042,
#80043),.UNSPECIFIED.,.F.,.F.,(4,1,1,4),(0.232788919908364,0.858032407070129,
1.01434327886057,1.32478005791959),.UNSPECIFIED.);
#10188=B_SPLINE_CURVE_WITH_KNOTS('',3,(#80044,#80045,#80046,#80047),
 .UNSPECIFIED.,.F.,.F.,(4,4),(0.124305417715433,0.168802697943275),
 .UNSPECIFIED.);
#10189=B_SPLINE_CURVE_WITH_KNOTS('',3,(#80050,#80051,#80052,#80053,#80054,
#80055),.UNSPECIFIED.,.F.,.F.,(4,1,1,4),(0.764611228840875,1.32070527910915,
1.69143464595466,2.06216401280017),.UNSPECIFIED.);
#10190=B_SPLINE_CURVE_WITH_KNOTS('',3,(#80057,#80058,#80059,#80060,#80061),
 .UNSPECIFIED.,.F.,.F.,(4,1,4),(0.,0.763473564994705,1.78143831832098),
 .UNSPECIFIED.);
#10191=B_SPLINE_CURVE_WITH_KNOTS('',3,(#80062,#80063,#80064,#80065,#80066,
#80067),.UNSPECIFIED.,.F.,.F.,(4,1,1,4),(1.472146927952,1.78258352306356,
2.09520509798177,2.56413746035908),.UNSPECIFIED.);
#10192=B_SPLINE_CURVE_WITH_KNOTS('',3,(#80068,#80069,#80070,#80071,#80072,
#80073),.UNSPECIFIED.,.F.,.F.,(4,2,4),(2.49842406090827,2.56616169967075,
2.63389933843323),.UNSPECIFIED.);
#10193=B_SPLINE_CURVE_WITH_KNOTS('',3,(#80133,#80134,#80135,#80136,#80137),
 .UNSPECIFIED.,.F.,.F.,(4,1,4),(-1.78143831832098,-0.763473564994705,0.),
 .UNSPECIFIED.);
#10194=B_SPLINE_CURVE_WITH_KNOTS('',3,(#80174,#80175,#80176,#80177),
 .UNSPECIFIED.,.F.,.F.,(4,4),(0.,0.0426050470946485),.UNSPECIFIED.);
#10195=B_SPLINE_CURVE_WITH_KNOTS('',3,(#80181,#80182,#80183,#80184,#80185,
#80186,#80187,#80188,#80189,#80190),.UNSPECIFIED.,.F.,.F.,(4,2,2,2,4),(-0.000382011303364944,
0.,0.0277433047160686,0.050141080254642,0.0665301715005073),
 .UNSPECIFIED.);
#10196=B_SPLINE_CURVE_WITH_KNOTS('',3,(#80195,#80196,#80197,#80198,#80199,
#80200,#80201),.UNSPECIFIED.,.F.,.F.,(4,3,4),(0.,0.00663332599231404,0.0112828850428522),
 .UNSPECIFIED.);
#10197=B_SPLINE_CURVE_WITH_KNOTS('',3,(#80203,#80204,#80205,#80206,#80207,
#80208,#80209,#80210,#80211,#80212,#80213,#80214),.UNSPECIFIED.,.F.,.F.,
(4,2,2,2,2,4),(19.4435968556708,19.7442925972668,20.064736080688,20.4210982332895,
20.7774603858911,21.1293548879222),.UNSPECIFIED.);
#10198=B_SPLINE_CURVE_WITH_KNOTS('',3,(#80215,#80216,#80217,#80218,#80219,
#80220,#80221),.UNSPECIFIED.,.F.,.F.,(4,3,4),(0.0497344367184578,0.0569822959606559,
0.0594305801700341),.UNSPECIFIED.);
#10199=B_SPLINE_CURVE_WITH_KNOTS('',3,(#80223,#80224,#80225,#80226,#80227,
#80228,#80229,#80230,#80231,#80232,#80233,#80234,#80235,#80236,#80237,#80238,
#80239,#80240,#80241,#80242,#80243,#80244,#80245,#80246,#80247,#80248,#80249,
#80250,#80251,#80252,#80253),.UNSPECIFIED.,.F.,.F.,(4,3,3,3,3,3,3,3,3,3,
4),(-0.0521489961175902,-0.0518402511587632,-0.0442584790581709,-0.0368221065001725,
-0.032029276053133,-0.0252715959769294,-0.0193928616961597,-0.0148241842185593,
-0.00805615521802194,-0.00166617749197499,0.),.UNSPECIFIED.);
#10200=B_SPLINE_CURVE_WITH_KNOTS('',3,(#80290,#80291,#80292,#80293,#80294,
#80295),.UNSPECIFIED.,.F.,.F.,(4,1,1,4),(0.285566041444524,0.663658803833889,
1.04175156622325,1.6088907098073),.UNSPECIFIED.);
#10201=B_SPLINE_CURVE_WITH_KNOTS('',3,(#80297,#80298,#80299,#80300,#80301,
#80302),.UNSPECIFIED.,.F.,.F.,(4,2,4),(2.49842406090827,2.56616169967075,
2.63389933843322),.UNSPECIFIED.);
#10202=B_SPLINE_CURVE_WITH_KNOTS('',3,(#80303,#80304,#80305,#80306,#80307,
#80308),.UNSPECIFIED.,.F.,.F.,(4,1,1,4),(0.261933028354804,0.750578938128915,
1.07634287797832,1.39992181764611),.UNSPECIFIED.);
#10203=B_SPLINE_CURVE_WITH_KNOTS('',3,(#80342,#80343,#80344,#80345),
 .UNSPECIFIED.,.F.,.F.,(4,4),(0.124414169098186,0.169128330998943),
 .UNSPECIFIED.);
#10204=B_SPLINE_CURVE_WITH_KNOTS('',3,(#80388,#80389,#80390,#80391,#80392,
#80393),.UNSPECIFIED.,.F.,.F.,(4,1,1,4),(0.263863277598129,0.819957327864215,
1.19068669470827,1.56141606155233),.UNSPECIFIED.);
#10205=B_SPLINE_CURVE_WITH_KNOTS('',3,(#80424,#80425,#80426,#80427),
 .UNSPECIFIED.,.F.,.F.,(4,4),(0.,0.0426050742017022),.UNSPECIFIED.);
#10206=B_SPLINE_CURVE_WITH_KNOTS('',3,(#80428,#80429,#80430,#80431,#80432,
#80433),.UNSPECIFIED.,.F.,.F.,(4,1,1,4),(1.38370165660982,1.53782715631916,
1.85044749661957,2.47568817722038),.UNSPECIFIED.);
#10207=B_SPLINE_CURVE_WITH_KNOTS('',3,(#80459,#80460,#80461,#80462,#80463),
 .UNSPECIFIED.,.F.,.F.,(4,1,4),(0.836467246372547,1.5999252909985,2.61786935049977),
 .UNSPECIFIED.);
#10208=B_SPLINE_CURVE_WITH_KNOTS('',3,(#80464,#80465,#80466,#80467,#80468),
 .UNSPECIFIED.,.F.,.F.,(4,1,4),(-2.61786935049977,-1.5999252909985,-0.836467246372547),
 .UNSPECIFIED.);
#10209=B_SPLINE_CURVE_WITH_KNOTS('',3,(#80495,#80496,#80497,#80498,#80499),
 .UNSPECIFIED.,.F.,.F.,(4,1,4),(0.733284842491785,1.49674691578015,2.51469634683131),
 .UNSPECIFIED.);
#10210=B_SPLINE_CURVE_WITH_KNOTS('',3,(#80538,#80539,#80540,#80541,#80542,
#80543),.UNSPECIFIED.,.F.,.F.,(4,1,1,4),(1.11836314594235,1.58729550831966,
1.89991708323787,2.21035367834943),.UNSPECIFIED.);
#10211=B_SPLINE_CURVE_WITH_KNOTS('',3,(#80544,#80545,#80546,#80547),
 .UNSPECIFIED.,.F.,.F.,(4,4),(0.124301071545834,0.168799110597043),
 .UNSPECIFIED.);
#10212=B_SPLINE_CURVE_WITH_KNOTS('',3,(#80549,#80550,#80551,#80552,#80553,
#80554),.UNSPECIFIED.,.F.,.F.,(4,2,4),(2.49842406090827,2.56616169967075,
2.63389933843322),.UNSPECIFIED.);
#10213=B_SPLINE_CURVE_WITH_KNOTS('',3,(#80585,#80586,#80587,#80588),
 .UNSPECIFIED.,.F.,.F.,(4,4),(0.117772194752307,0.161941500778177),
 .UNSPECIFIED.);
#10214=B_SPLINE_CURVE_WITH_KNOTS('',3,(#80594,#80595,#80596,#80597,#80598),
 .UNSPECIFIED.,.F.,.F.,(4,1,4),(-2.61786935049979,-1.59992529099851,-0.836467246372557),
 .UNSPECIFIED.);
#10215=B_SPLINE_CURVE_WITH_KNOTS('',3,(#80626,#80627,#80628,#80629,#80630),
 .UNSPECIFIED.,.F.,.F.,(4,1,4),(0.836467246372557,1.59992529099851,2.61786935049979),
 .UNSPECIFIED.);
#10216=B_SPLINE_CURVE_WITH_KNOTS('',3,(#80662,#80663,#80664,#80665),
 .UNSPECIFIED.,.F.,.F.,(4,4),(0.,0.0426050742067116),.UNSPECIFIED.);
#10217=B_SPLINE_CURVE_WITH_KNOTS('',3,(#80667,#80668,#80669,#80670,#80671,
#80672,#80673,#80674,#80675,#80676,#80677,#80678,#80679),.UNSPECIFIED.,
 .F.,.F.,(4,3,3,3,4),(0.,0.00668995933612563,0.0134216136901844,0.0145801214849255,
0.0186681351775812),.UNSPECIFIED.);
#10218=B_SPLINE_CURVE_WITH_KNOTS('',3,(#80680,#80681,#80682,#80683,#80684,
#80685),.UNSPECIFIED.,.F.,.F.,(4,1,1,4),(1.383705910458,1.53783209167054,
1.85045379098313,2.47569718960832),.UNSPECIFIED.);
#10219=B_SPLINE_CURVE_WITH_KNOTS('',3,(#80712,#80713,#80714,#80715,#80716),
 .UNSPECIFIED.,.F.,.F.,(4,1,4),(0.733284842491785,1.49674691578015,2.51469634683131),
 .UNSPECIFIED.);
#10220=B_SPLINE_CURVE_WITH_KNOTS('',3,(#80719,#80720,#80721,#80722,#80723),
 .UNSPECIFIED.,.F.,.F.,(4,1,4),(-2.51469634683131,-1.49674691578015,-0.733284842491785),
 .UNSPECIFIED.);
#10221=B_SPLINE_CURVE_WITH_KNOTS('',3,(#80761,#80762,#80763,#80764,#80765,
#80766),.UNSPECIFIED.,.F.,.F.,(4,1,1,4),(1.11836314594235,1.58729550831966,
1.89991708323787,2.21035367834943),.UNSPECIFIED.);
#10222=B_SPLINE_CURVE_WITH_KNOTS('',3,(#80768,#80769,#80770,#80771,#80772,
#80773,#80774,#80775,#80776,#80777,#80778,#80779,#80780),.UNSPECIFIED.,
 .F.,.F.,(4,3,3,3,4),(0.0105027337450464,0.0145912333589941,0.0213179561732657,
0.0280163477739932,0.0291731591110282),.UNSPECIFIED.);
#10223=B_SPLINE_CURVE_WITH_KNOTS('',3,(#80781,#80782,#80783,#80784),
 .UNSPECIFIED.,.F.,.F.,(4,4),(0.124301070545925,0.168799108950048),
 .UNSPECIFIED.);
#10224=B_SPLINE_CURVE_WITH_KNOTS('',3,(#80818,#80819,#80820,#80821),
 .UNSPECIFIED.,.F.,.F.,(4,4),(0.,0.0418633800463106),.UNSPECIFIED.);
#10225=B_SPLINE_CURVE_WITH_KNOTS('',3,(#80822,#80823,#80824,#80825,#80826,
#80827,#80828,#80829,#80830,#80831,#80832,#80833,#80834),.UNSPECIFIED.,
 .F.,.F.,(4,3,3,3,4),(0.,0.00668995077308426,0.0134216120032876,0.0145801130032437,
0.0186681351443671),.UNSPECIFIED.);
#10226=B_SPLINE_CURVE_WITH_KNOTS('',3,(#80839,#80840,#80841,#80842,#80843,
#80844),.UNSPECIFIED.,.F.,.F.,(4,2,4),(2.49842406090827,2.56616169967075,
2.63389933843322),.UNSPECIFIED.);
#10227=B_SPLINE_CURVE_WITH_KNOTS('',3,(#80878,#80879,#80880,#80881,#80882,
#80883,#80884,#80885,#80886,#80887,#80888,#80889,#80890),.UNSPECIFIED.,
 .F.,.F.,(4,3,3,3,4),(0.01048394913021,0.014570593673781,0.0194264046381645,
0.0261580092146828,0.0291307560165872),.UNSPECIFIED.);
#10228=B_SPLINE_CURVE_WITH_KNOTS('',3,(#80891,#80892,#80893,#80894),
 .UNSPECIFIED.,.F.,.F.,(4,4),(0.117772194557587,0.161941500466076),
 .UNSPECIFIED.);
#10229=B_SPLINE_CURVE_WITH_KNOTS('',3,(#80896,#80897,#80898,#80899,#80900,
#80901,#80902,#80903,#80904,#80905),.UNSPECIFIED.,.F.,.F.,(4,2,2,2,4),(-0.000382011302730862,
0.,0.0277433047156941,0.0501410802538888,0.0665301714994503),
 .UNSPECIFIED.);
#10230=B_SPLINE_CURVE_WITH_KNOTS('',3,(#80906,#80907,#80908,#80909,#80910,
#80911,#80912),.UNSPECIFIED.,.F.,.F.,(4,3,4),(0.0497344367184662,0.0569822959607033,
0.059430580170041),.UNSPECIFIED.);
#10231=B_SPLINE_CURVE_WITH_KNOTS('',3,(#80915,#80916,#80917,#80918,#80919,
#80920,#80921,#80922,#80923,#80924),.UNSPECIFIED.,.F.,.F.,(4,2,2,2,4),(-0.0578449501866477,
-0.0575146564880824,-0.0335318637466033,-0.0141685076513094,0.),
 .UNSPECIFIED.);
#10232=B_SPLINE_CURVE_WITH_KNOTS('',3,(#80956,#80957,#80958,#80959),
 .UNSPECIFIED.,.F.,.F.,(4,4),(0.,0.0426050470946472),.UNSPECIFIED.);
#10233=B_SPLINE_CURVE_WITH_KNOTS('',3,(#80960,#80961,#80962,#80963,#80964,
#80965,#80966),.UNSPECIFIED.,.F.,.F.,(4,3,4),(0.,0.00724674346847173,0.00972691805001191),
 .UNSPECIFIED.);
#11499=LINE('',#78387,#13993);
#11500=LINE('',#78390,#13994);
#11501=LINE('',#78393,#13995);
#11502=LINE('',#78397,#13996);
#11503=LINE('',#78399,#13997);
#11504=LINE('',#78400,#13998);
#11505=LINE('',#78403,#13999);
#11506=LINE('',#78404,#14000);
#11507=LINE('',#78408,#14001);
#11508=LINE('',#78414,#14002);
#11509=LINE('',#78417,#14003);
#11510=LINE('',#78420,#14004);
#11511=LINE('',#78422,#14005);
#11512=LINE('',#78423,#14006);
#11513=LINE('',#78480,#14007);
#11514=LINE('',#78483,#14008);
#11515=LINE('',#78487,#14009);
#11516=LINE('',#78491,#14010);
#11517=LINE('',#78495,#14011);
#11518=LINE('',#78499,#14012);
#11519=LINE('',#78503,#14013);
#11520=LINE('',#78507,#14014);
#11521=LINE('',#78511,#14015);
#11522=LINE('',#78515,#14016);
#11523=LINE('',#78519,#14017);
#11524=LINE('',#78523,#14018);
#11525=LINE('',#78527,#14019);
#11526=LINE('',#78531,#14020);
#11527=LINE('',#78535,#14021);
#11528=LINE('',#78539,#14022);
#11529=LINE('',#78543,#14023);
#11530=LINE('',#78547,#14024);
#11531=LINE('',#78551,#14025);
#11532=LINE('',#78555,#14026);
#11533=LINE('',#78559,#14027);
#11534=LINE('',#78563,#14028);
#11535=LINE('',#78567,#14029);
#11536=LINE('',#78571,#14030);
#11537=LINE('',#78575,#14031);
#11538=LINE('',#78579,#14032);
#11539=LINE('',#78583,#14033);
#11540=LINE('',#78587,#14034);
#11541=LINE('',#78591,#14035);
#11542=LINE('',#78595,#14036);
#11543=LINE('',#78599,#14037);
#11544=LINE('',#78603,#14038);
#11545=LINE('',#78607,#14039);
#11546=LINE('',#78611,#14040);
#11547=LINE('',#78615,#14041);
#11548=LINE('',#78619,#14042);
#11549=LINE('',#78623,#14043);
#11550=LINE('',#78627,#14044);
#11551=LINE('',#78631,#14045);
#11552=LINE('',#78635,#14046);
#11553=LINE('',#78639,#14047);
#11554=LINE('',#78643,#14048);
#11555=LINE('',#78647,#14049);
#11556=LINE('',#78651,#14050);
#11557=LINE('',#78655,#14051);
#11558=LINE('',#78659,#14052);
#11559=LINE('',#78663,#14053);
#11560=LINE('',#78667,#14054);
#11561=LINE('',#78671,#14055);
#11562=LINE('',#78675,#14056);
#11563=LINE('',#78679,#14057);
#11564=LINE('',#78683,#14058);
#11565=LINE('',#78687,#14059);
#11566=LINE('',#78691,#14060);
#11567=LINE('',#78695,#14061);
#11568=LINE('',#78699,#14062);
#11569=LINE('',#78703,#14063);
#11570=LINE('',#78707,#14064);
#11571=LINE('',#78711,#14065);
#11572=LINE('',#78715,#14066);
#11573=LINE('',#78719,#14067);
#11574=LINE('',#78723,#14068);
#11575=LINE('',#78727,#14069);
#11576=LINE('',#78731,#14070);
#11577=LINE('',#78735,#14071);
#11578=LINE('',#78739,#14072);
#11579=LINE('',#78743,#14073);
#11580=LINE('',#78747,#14074);
#11581=LINE('',#78751,#14075);
#11582=LINE('',#78754,#14076);
#11583=LINE('',#78759,#14077);
#11584=LINE('',#78760,#14078);
#11585=LINE('',#78763,#14079);
#11586=LINE('',#78764,#14080);
#11587=LINE('',#78787,#14081);
#11588=LINE('',#78791,#14082);
#11589=LINE('',#78795,#14083);
#11590=LINE('',#78799,#14084);
#11591=LINE('',#78803,#14085);
#11592=LINE('',#78807,#14086);
#11593=LINE('',#78809,#14087);
#11594=LINE('',#78811,#14088);
#11595=LINE('',#78812,#14089);
#11596=LINE('',#78814,#14090);
#11597=LINE('',#78816,#14091);
#11598=LINE('',#78818,#14092);
#11599=LINE('',#78819,#14093);
#11600=LINE('',#78821,#14094);
#11601=LINE('',#78823,#14095);
#11602=LINE('',#78828,#14096);
#11603=LINE('',#78829,#14097);
#11604=LINE('',#78832,#14098);
#11605=LINE('',#78836,#14099);
#11606=LINE('',#78838,#14100);
#11607=LINE('',#78839,#14101);
#11608=LINE('',#78841,#14102);
#11609=LINE('',#78843,#14103);
#11610=LINE('',#78848,#14104);
#11611=LINE('',#78849,#14105);
#11612=LINE('',#78852,#14106);
#11613=LINE('',#78856,#14107);
#11614=LINE('',#78878,#14108);
#11615=LINE('',#78882,#14109);
#11616=LINE('',#78886,#14110);
#11617=LINE('',#78890,#14111);
#11618=LINE('',#78894,#14112);
#11619=LINE('',#78898,#14113);
#11620=LINE('',#78901,#14114);
#11621=LINE('',#78903,#14115);
#11622=LINE('',#78905,#14116);
#11623=LINE('',#78907,#14117);
#11624=LINE('',#78908,#14118);
#11625=LINE('',#78910,#14119);
#11626=LINE('',#78912,#14120);
#11627=LINE('',#78913,#14121);
#11628=LINE('',#78915,#14122);
#11629=LINE('',#78917,#14123);
#11630=LINE('',#78918,#14124);
#11631=LINE('',#78920,#14125);
#11632=LINE('',#78922,#14126);
#11633=LINE('',#78923,#14127);
#11634=LINE('',#78925,#14128);
#11635=LINE('',#78930,#14129);
#11636=LINE('',#78931,#14130);
#11637=LINE('',#78934,#14131);
#11638=LINE('',#78952,#14132);
#11639=LINE('',#78953,#14133);
#11640=LINE('',#78958,#14134);
#11641=LINE('',#78959,#14135);
#11642=LINE('',#78962,#14136);
#11643=LINE('',#78964,#14137);
#11644=LINE('',#78981,#14138);
#11645=LINE('',#78983,#14139);
#11646=LINE('',#78984,#14140);
#11647=LINE('',#78989,#14141);
#11648=LINE('',#78990,#14142);
#11649=LINE('',#78993,#14143);
#11650=LINE('',#78997,#14144);
#11651=LINE('',#79019,#14145);
#11652=LINE('',#79023,#14146);
#11653=LINE('',#79027,#14147);
#11654=LINE('',#79031,#14148);
#11655=LINE('',#79035,#14149);
#11656=LINE('',#79039,#14150);
#11657=LINE('',#79042,#14151);
#11658=LINE('',#79044,#14152);
#11659=LINE('',#79046,#14153);
#11660=LINE('',#79048,#14154);
#11661=LINE('',#79049,#14155);
#11662=LINE('',#79051,#14156);
#11663=LINE('',#79053,#14157);
#11664=LINE('',#79054,#14158);
#11665=LINE('',#79056,#14159);
#11666=LINE('',#79058,#14160);
#11667=LINE('',#79059,#14161);
#11668=LINE('',#79061,#14162);
#11669=LINE('',#79063,#14163);
#11670=LINE('',#79064,#14164);
#11671=LINE('',#79066,#14165);
#11672=LINE('',#79071,#14166);
#11673=LINE('',#79072,#14167);
#11674=LINE('',#79075,#14168);
#11675=LINE('',#79093,#14169);
#11676=LINE('',#79094,#14170);
#11677=LINE('',#79099,#14171);
#11678=LINE('',#79100,#14172);
#11679=LINE('',#79103,#14173);
#11680=LINE('',#79105,#14174);
#11681=LINE('',#79122,#14175);
#11682=LINE('',#79124,#14176);
#11683=LINE('',#79125,#14177);
#11684=LINE('',#79130,#14178);
#11685=LINE('',#79131,#14179);
#11686=LINE('',#79134,#14180);
#11687=LINE('',#79138,#14181);
#11688=LINE('',#79160,#14182);
#11689=LINE('',#79164,#14183);
#11690=LINE('',#79168,#14184);
#11691=LINE('',#79172,#14185);
#11692=LINE('',#79176,#14186);
#11693=LINE('',#79180,#14187);
#11694=LINE('',#79183,#14188);
#11695=LINE('',#79185,#14189);
#11696=LINE('',#79187,#14190);
#11697=LINE('',#79189,#14191);
#11698=LINE('',#79190,#14192);
#11699=LINE('',#79192,#14193);
#11700=LINE('',#79194,#14194);
#11701=LINE('',#79195,#14195);
#11702=LINE('',#79197,#14196);
#11703=LINE('',#79199,#14197);
#11704=LINE('',#79200,#14198);
#11705=LINE('',#79202,#14199);
#11706=LINE('',#79204,#14200);
#11707=LINE('',#79205,#14201);
#11708=LINE('',#79207,#14202);
#11709=LINE('',#79212,#14203);
#11710=LINE('',#79213,#14204);
#11711=LINE('',#79216,#14205);
#11712=LINE('',#79234,#14206);
#11713=LINE('',#79235,#14207);
#11714=LINE('',#79240,#14208);
#11715=LINE('',#79241,#14209);
#11716=LINE('',#79244,#14210);
#11717=LINE('',#79246,#14211);
#11718=LINE('',#79263,#14212);
#11719=LINE('',#79265,#14213);
#11720=LINE('',#79266,#14214);
#11721=LINE('',#79271,#14215);
#11722=LINE('',#79272,#14216);
#11723=LINE('',#79275,#14217);
#11724=LINE('',#79279,#14218);
#11725=LINE('',#79301,#14219);
#11726=LINE('',#79305,#14220);
#11727=LINE('',#79309,#14221);
#11728=LINE('',#79313,#14222);
#11729=LINE('',#79317,#14223);
#11730=LINE('',#79321,#14224);
#11731=LINE('',#79324,#14225);
#11732=LINE('',#79326,#14226);
#11733=LINE('',#79328,#14227);
#11734=LINE('',#79330,#14228);
#11735=LINE('',#79331,#14229);
#11736=LINE('',#79333,#14230);
#11737=LINE('',#79335,#14231);
#11738=LINE('',#79336,#14232);
#11739=LINE('',#79338,#14233);
#11740=LINE('',#79340,#14234);
#11741=LINE('',#79341,#14235);
#11742=LINE('',#79343,#14236);
#11743=LINE('',#79345,#14237);
#11744=LINE('',#79346,#14238);
#11745=LINE('',#79348,#14239);
#11746=LINE('',#79353,#14240);
#11747=LINE('',#79354,#14241);
#11748=LINE('',#79357,#14242);
#11749=LINE('',#79375,#14243);
#11750=LINE('',#79376,#14244);
#11751=LINE('',#79381,#14245);
#11752=LINE('',#79382,#14246);
#11753=LINE('',#79385,#14247);
#11754=LINE('',#79387,#14248);
#11755=LINE('',#79404,#14249);
#11756=LINE('',#79406,#14250);
#11757=LINE('',#79407,#14251);
#11758=LINE('',#79412,#14252);
#11759=LINE('',#79413,#14253);
#11760=LINE('',#79416,#14254);
#11761=LINE('',#79420,#14255);
#11762=LINE('',#79442,#14256);
#11763=LINE('',#79446,#14257);
#11764=LINE('',#79450,#14258);
#11765=LINE('',#79454,#14259);
#11766=LINE('',#79458,#14260);
#11767=LINE('',#79462,#14261);
#11768=LINE('',#79465,#14262);
#11769=LINE('',#79467,#14263);
#11770=LINE('',#79469,#14264);
#11771=LINE('',#79471,#14265);
#11772=LINE('',#79472,#14266);
#11773=LINE('',#79474,#14267);
#11774=LINE('',#79476,#14268);
#11775=LINE('',#79477,#14269);
#11776=LINE('',#79479,#14270);
#11777=LINE('',#80504,#14271);
#11778=LINE('',#80728,#14272);
#11779=LINE('',#80729,#14273);
#11780=LINE('',#80969,#14274);
#11781=LINE('',#80970,#14275);
#11782=LINE('',#80972,#14276);
#11783=LINE('',#80974,#14277);
#11784=LINE('',#80976,#14278);
#11785=LINE('',#80978,#14279);
#11786=LINE('',#80982,#14280);
#11787=LINE('',#80984,#14281);
#11788=LINE('',#80986,#14282);
#11789=LINE('',#80996,#14283);
#11790=LINE('',#81006,#14284);
#11791=LINE('',#81008,#14285);
#11792=LINE('',#81018,#14286);
#11793=LINE('',#81020,#14287);
#11794=LINE('',#81030,#14288);
#11795=LINE('',#81034,#14289);
#11796=LINE('',#81035,#14290);
#11797=LINE('',#81037,#14291);
#11798=LINE('',#81040,#14292);
#11799=LINE('',#81042,#14293);
#11800=LINE('',#81045,#14294);
#11801=LINE('',#81047,#14295);
#11802=LINE('',#81052,#14296);
#11803=LINE('',#81054,#14297);
#11804=LINE('',#81056,#14298);
#13993=VECTOR('',#51893,10.);
#13994=VECTOR('',#51896,10.);
#13995=VECTOR('',#51899,10.);
#13996=VECTOR('',#51902,10.);
#13997=VECTOR('',#51903,10.);
#13998=VECTOR('',#51904,10.);
#13999=VECTOR('',#51907,10.);
#14000=VECTOR('',#51908,10.);
#14001=VECTOR('',#51913,10.);
#14002=VECTOR('',#51918,10.);
#14003=VECTOR('',#51921,10.);
#14004=VECTOR('',#51924,10.);
#14005=VECTOR('',#51925,10.);
#14006=VECTOR('',#51926,10.);
#14007=VECTOR('',#51941,10.);
#14008=VECTOR('',#51944,10.);
#14009=VECTOR('',#51947,10.);
#14010=VECTOR('',#51950,10.);
#14011=VECTOR('',#51953,10.);
#14012=VECTOR('',#51956,10.);
#14013=VECTOR('',#51959,10.);
#14014=VECTOR('',#51962,10.);
#14015=VECTOR('',#51965,10.);
#14016=VECTOR('',#51968,10.);
#14017=VECTOR('',#51971,10.);
#14018=VECTOR('',#51974,10.);
#14019=VECTOR('',#51977,10.);
#14020=VECTOR('',#51980,10.);
#14021=VECTOR('',#51983,10.);
#14022=VECTOR('',#51986,10.);
#14023=VECTOR('',#51989,10.);
#14024=VECTOR('',#51992,10.);
#14025=VECTOR('',#51995,10.);
#14026=VECTOR('',#51998,10.);
#14027=VECTOR('',#52001,10.);
#14028=VECTOR('',#52004,10.);
#14029=VECTOR('',#52007,10.);
#14030=VECTOR('',#52010,10.);
#14031=VECTOR('',#52013,10.);
#14032=VECTOR('',#52016,10.);
#14033=VECTOR('',#52019,10.);
#14034=VECTOR('',#52022,10.);
#14035=VECTOR('',#52025,10.);
#14036=VECTOR('',#52028,10.);
#14037=VECTOR('',#52031,10.);
#14038=VECTOR('',#52034,10.);
#14039=VECTOR('',#52037,10.);
#14040=VECTOR('',#52040,10.);
#14041=VECTOR('',#52043,10.);
#14042=VECTOR('',#52046,10.);
#14043=VECTOR('',#52049,10.);
#14044=VECTOR('',#52052,10.);
#14045=VECTOR('',#52055,10.);
#14046=VECTOR('',#52058,10.);
#14047=VECTOR('',#52061,10.);
#14048=VECTOR('',#52064,10.);
#14049=VECTOR('',#52067,10.);
#14050=VECTOR('',#52070,10.);
#14051=VECTOR('',#52073,10.);
#14052=VECTOR('',#52076,10.);
#14053=VECTOR('',#52079,10.);
#14054=VECTOR('',#52082,10.);
#14055=VECTOR('',#52085,10.);
#14056=VECTOR('',#52088,10.);
#14057=VECTOR('',#52091,10.);
#14058=VECTOR('',#52094,10.);
#14059=VECTOR('',#52097,10.);
#14060=VECTOR('',#52100,10.);
#14061=VECTOR('',#52103,10.);
#14062=VECTOR('',#52106,10.);
#14063=VECTOR('',#52109,10.);
#14064=VECTOR('',#52112,10.);
#14065=VECTOR('',#52115,10.);
#14066=VECTOR('',#52118,10.);
#14067=VECTOR('',#52121,10.);
#14068=VECTOR('',#52124,10.);
#14069=VECTOR('',#52127,10.);
#14070=VECTOR('',#52130,10.);
#14071=VECTOR('',#52133,10.);
#14072=VECTOR('',#52136,10.);
#14073=VECTOR('',#52139,10.);
#14074=VECTOR('',#52142,10.);
#14075=VECTOR('',#52145,10.);
#14076=VECTOR('',#52148,10.);
#14077=VECTOR('',#52153,10.);
#14078=VECTOR('',#52154,10.);
#14079=VECTOR('',#52157,10.);
#14080=VECTOR('',#52158,10.);
#14081=VECTOR('',#52167,10.);
#14082=VECTOR('',#52170,10.);
#14083=VECTOR('',#52173,10.);
#14084=VECTOR('',#52176,10.);
#14085=VECTOR('',#52179,10.);
#14086=VECTOR('',#52182,10.);
#14087=VECTOR('',#52185,10.);
#14088=VECTOR('',#52188,10.);
#14089=VECTOR('',#52189,10.);
#14090=VECTOR('',#52192,10.);
#14091=VECTOR('',#52195,10.);
#14092=VECTOR('',#52198,10.);
#14093=VECTOR('',#52199,10.);
#14094=VECTOR('',#52202,10.);
#14095=VECTOR('',#52205,10.);
#14096=VECTOR('',#52210,10.);
#14097=VECTOR('',#52211,10.);
#14098=VECTOR('',#52214,10.);
#14099=VECTOR('',#52217,10.);
#14100=VECTOR('',#52218,10.);
#14101=VECTOR('',#52219,10.);
#14102=VECTOR('',#52222,10.);
#14103=VECTOR('',#52225,10.);
#14104=VECTOR('',#52230,10.);
#14105=VECTOR('',#52231,10.);
#14106=VECTOR('',#52234,10.);
#14107=VECTOR('',#52237,10.);
#14108=VECTOR('',#52244,10.);
#14109=VECTOR('',#52247,10.);
#14110=VECTOR('',#52250,10.);
#14111=VECTOR('',#52253,10.);
#14112=VECTOR('',#52256,10.);
#14113=VECTOR('',#52259,10.);
#14114=VECTOR('',#52262,10.);
#14115=VECTOR('',#52265,10.);
#14116=VECTOR('',#52268,10.);
#14117=VECTOR('',#52271,10.);
#14118=VECTOR('',#52272,10.);
#14119=VECTOR('',#52275,10.);
#14120=VECTOR('',#52278,10.);
#14121=VECTOR('',#52279,10.);
#14122=VECTOR('',#52282,10.);
#14123=VECTOR('',#52285,10.);
#14124=VECTOR('',#52286,10.);
#14125=VECTOR('',#52289,10.);
#14126=VECTOR('',#52292,10.);
#14127=VECTOR('',#52293,10.);
#14128=VECTOR('',#52296,10.);
#14129=VECTOR('',#52301,10.);
#14130=VECTOR('',#52302,10.);
#14131=VECTOR('',#52305,10.);
#14132=VECTOR('',#52308,10.);
#14133=VECTOR('',#52309,10.);
#14134=VECTOR('',#52314,10.);
#14135=VECTOR('',#52315,10.);
#14136=VECTOR('',#52318,10.);
#14137=VECTOR('',#52319,10.);
#14138=VECTOR('',#52322,10.);
#14139=VECTOR('',#52325,10.);
#14140=VECTOR('',#52326,10.);
#14141=VECTOR('',#52331,10.);
#14142=VECTOR('',#52332,10.);
#14143=VECTOR('',#52335,10.);
#14144=VECTOR('',#52338,10.);
#14145=VECTOR('',#52345,10.);
#14146=VECTOR('',#52348,10.);
#14147=VECTOR('',#52351,10.);
#14148=VECTOR('',#52354,10.);
#14149=VECTOR('',#52357,10.);
#14150=VECTOR('',#52360,10.);
#14151=VECTOR('',#52363,10.);
#14152=VECTOR('',#52366,10.);
#14153=VECTOR('',#52369,10.);
#14154=VECTOR('',#52372,10.);
#14155=VECTOR('',#52373,10.);
#14156=VECTOR('',#52376,10.);
#14157=VECTOR('',#52379,10.);
#14158=VECTOR('',#52380,10.);
#14159=VECTOR('',#52383,10.);
#14160=VECTOR('',#52386,10.);
#14161=VECTOR('',#52387,10.);
#14162=VECTOR('',#52390,10.);
#14163=VECTOR('',#52393,10.);
#14164=VECTOR('',#52394,10.);
#14165=VECTOR('',#52397,10.);
#14166=VECTOR('',#52402,10.);
#14167=VECTOR('',#52403,10.);
#14168=VECTOR('',#52406,10.);
#14169=VECTOR('',#52409,10.);
#14170=VECTOR('',#52410,10.);
#14171=VECTOR('',#52415,10.);
#14172=VECTOR('',#52416,10.);
#14173=VECTOR('',#52419,10.);
#14174=VECTOR('',#52420,10.);
#14175=VECTOR('',#52423,10.);
#14176=VECTOR('',#52426,10.);
#14177=VECTOR('',#52427,10.);
#14178=VECTOR('',#52432,10.);
#14179=VECTOR('',#52433,10.);
#14180=VECTOR('',#52436,10.);
#14181=VECTOR('',#52439,10.);
#14182=VECTOR('',#52446,10.);
#14183=VECTOR('',#52449,10.);
#14184=VECTOR('',#52452,10.);
#14185=VECTOR('',#52455,10.);
#14186=VECTOR('',#52458,10.);
#14187=VECTOR('',#52461,10.);
#14188=VECTOR('',#52464,10.);
#14189=VECTOR('',#52467,10.);
#14190=VECTOR('',#52470,10.);
#14191=VECTOR('',#52473,10.);
#14192=VECTOR('',#52474,10.);
#14193=VECTOR('',#52477,10.);
#14194=VECTOR('',#52480,10.);
#14195=VECTOR('',#52481,10.);
#14196=VECTOR('',#52484,10.);
#14197=VECTOR('',#52487,10.);
#14198=VECTOR('',#52488,10.);
#14199=VECTOR('',#52491,10.);
#14200=VECTOR('',#52494,10.);
#14201=VECTOR('',#52495,10.);
#14202=VECTOR('',#52498,10.);
#14203=VECTOR('',#52503,10.);
#14204=VECTOR('',#52504,10.);
#14205=VECTOR('',#52507,10.);
#14206=VECTOR('',#52510,10.);
#14207=VECTOR('',#52511,10.);
#14208=VECTOR('',#52516,10.);
#14209=VECTOR('',#52517,10.);
#14210=VECTOR('',#52520,10.);
#14211=VECTOR('',#52521,10.);
#14212=VECTOR('',#52524,10.);
#14213=VECTOR('',#52527,10.);
#14214=VECTOR('',#52528,10.);
#14215=VECTOR('',#52533,10.);
#14216=VECTOR('',#52534,10.);
#14217=VECTOR('',#52537,10.);
#14218=VECTOR('',#52540,10.);
#14219=VECTOR('',#52547,10.);
#14220=VECTOR('',#52550,10.);
#14221=VECTOR('',#52553,10.);
#14222=VECTOR('',#52556,10.);
#14223=VECTOR('',#52559,10.);
#14224=VECTOR('',#52562,10.);
#14225=VECTOR('',#52565,10.);
#14226=VECTOR('',#52568,10.);
#14227=VECTOR('',#52571,10.);
#14228=VECTOR('',#52574,10.);
#14229=VECTOR('',#52575,10.);
#14230=VECTOR('',#52578,10.);
#14231=VECTOR('',#52581,10.);
#14232=VECTOR('',#52582,10.);
#14233=VECTOR('',#52585,10.);
#14234=VECTOR('',#52588,10.);
#14235=VECTOR('',#52589,10.);
#14236=VECTOR('',#52592,10.);
#14237=VECTOR('',#52595,10.);
#14238=VECTOR('',#52596,10.);
#14239=VECTOR('',#52599,10.);
#14240=VECTOR('',#52604,10.);
#14241=VECTOR('',#52605,10.);
#14242=VECTOR('',#52608,10.);
#14243=VECTOR('',#52611,10.);
#14244=VECTOR('',#52612,10.);
#14245=VECTOR('',#52617,10.);
#14246=VECTOR('',#52618,10.);
#14247=VECTOR('',#52621,10.);
#14248=VECTOR('',#52622,10.);
#14249=VECTOR('',#52625,10.);
#14250=VECTOR('',#52628,10.);
#14251=VECTOR('',#52629,10.);
#14252=VECTOR('',#52634,10.);
#14253=VECTOR('',#52635,10.);
#14254=VECTOR('',#52638,10.);
#14255=VECTOR('',#52641,10.);
#14256=VECTOR('',#52648,10.);
#14257=VECTOR('',#52651,10.);
#14258=VECTOR('',#52654,10.);
#14259=VECTOR('',#52657,10.);
#14260=VECTOR('',#52660,10.);
#14261=VECTOR('',#52663,10.);
#14262=VECTOR('',#52666,10.);
#14263=VECTOR('',#52669,10.);
#14264=VECTOR('',#52672,10.);
#14265=VECTOR('',#52675,10.);
#14266=VECTOR('',#52676,10.);
#14267=VECTOR('',#52679,10.);
#14268=VECTOR('',#52682,10.);
#14269=VECTOR('',#52683,10.);
#14270=VECTOR('',#52686,10.);
#14271=VECTOR('',#52879,10.);
#14272=VECTOR('',#52906,10.);
#14273=VECTOR('',#52907,10.);
#14274=VECTOR('',#52928,10.);
#14275=VECTOR('',#52929,10.);
#14276=VECTOR('',#52932,10.);
#14277=VECTOR('',#52935,10.);
#14278=VECTOR('',#52938,10.);
#14279=VECTOR('',#52941,10.);
#14280=VECTOR('',#52948,10.);
#14281=VECTOR('',#52951,10.);
#14282=VECTOR('',#52954,10.);
#14283=VECTOR('',#52973,10.);
#14284=VECTOR('',#52992,10.);
#14285=VECTOR('',#52995,10.);
#14286=VECTOR('',#53014,10.);
#14287=VECTOR('',#53017,10.);
#14288=VECTOR('',#53036,10.);
#14289=VECTOR('',#53043,10.);
#14290=VECTOR('',#53044,10.);
#14291=VECTOR('',#53047,10.);
#14292=VECTOR('',#53052,10.);
#14293=VECTOR('',#53055,10.);
#14294=VECTOR('',#53060,10.);
#14295=VECTOR('',#53063,10.);
#14296=VECTOR('',#53072,10.);
#14297=VECTOR('',#53075,10.);
#14298=VECTOR('',#53078,10.);
#17301=VERTEX_POINT('',#78383);
#17302=VERTEX_POINT('',#78384);
#17303=VERTEX_POINT('',#78386);
#17304=VERTEX_POINT('',#78388);
#17305=VERTEX_POINT('',#78392);
#17306=VERTEX_POINT('',#78394);
#17307=VERTEX_POINT('',#78396);
#17308=VERTEX_POINT('',#78398);
#17309=VERTEX_POINT('',#78402);
#17310=VERTEX_POINT('',#78406);
#17311=VERTEX_POINT('',#78410);
#17312=VERTEX_POINT('',#78411);
#17313=VERTEX_POINT('',#78413);
#17314=VERTEX_POINT('',#78415);
#17315=VERTEX_POINT('',#78419);
#17316=VERTEX_POINT('',#78421);
#17317=VERTEX_POINT('',#78425);
#17318=VERTEX_POINT('',#78426);
#17319=VERTEX_POINT('',#78428);
#17320=VERTEX_POINT('',#78435);
#17321=VERTEX_POINT('',#78437);
#17322=VERTEX_POINT('',#78444);
#17323=VERTEX_POINT('',#78446);
#17324=VERTEX_POINT('',#78453);
#17325=VERTEX_POINT('',#78455);
#17326=VERTEX_POINT('',#78462);
#17327=VERTEX_POINT('',#78464);
#17328=VERTEX_POINT('',#78471);
#17329=VERTEX_POINT('',#78479);
#17330=VERTEX_POINT('',#78482);
#17331=VERTEX_POINT('',#78484);
#17332=VERTEX_POINT('',#78486);
#17333=VERTEX_POINT('',#78488);
#17334=VERTEX_POINT('',#78490);
#17335=VERTEX_POINT('',#78492);
#17336=VERTEX_POINT('',#78494);
#17337=VERTEX_POINT('',#78496);
#17338=VERTEX_POINT('',#78498);
#17339=VERTEX_POINT('',#78500);
#17340=VERTEX_POINT('',#78502);
#17341=VERTEX_POINT('',#78504);
#17342=VERTEX_POINT('',#78506);
#17343=VERTEX_POINT('',#78508);
#17344=VERTEX_POINT('',#78510);
#17345=VERTEX_POINT('',#78512);
#17346=VERTEX_POINT('',#78514);
#17347=VERTEX_POINT('',#78516);
#17348=VERTEX_POINT('',#78518);
#17349=VERTEX_POINT('',#78520);
#17350=VERTEX_POINT('',#78522);
#17351=VERTEX_POINT('',#78524);
#17352=VERTEX_POINT('',#78526);
#17353=VERTEX_POINT('',#78528);
#17354=VERTEX_POINT('',#78530);
#17355=VERTEX_POINT('',#78532);
#17356=VERTEX_POINT('',#78534);
#17357=VERTEX_POINT('',#78536);
#17358=VERTEX_POINT('',#78538);
#17359=VERTEX_POINT('',#78540);
#17360=VERTEX_POINT('',#78542);
#17361=VERTEX_POINT('',#78544);
#17362=VERTEX_POINT('',#78546);
#17363=VERTEX_POINT('',#78548);
#17364=VERTEX_POINT('',#78550);
#17365=VERTEX_POINT('',#78552);
#17366=VERTEX_POINT('',#78554);
#17367=VERTEX_POINT('',#78556);
#17368=VERTEX_POINT('',#78558);
#17369=VERTEX_POINT('',#78560);
#17370=VERTEX_POINT('',#78562);
#17371=VERTEX_POINT('',#78564);
#17372=VERTEX_POINT('',#78566);
#17373=VERTEX_POINT('',#78568);
#17374=VERTEX_POINT('',#78570);
#17375=VERTEX_POINT('',#78572);
#17376=VERTEX_POINT('',#78574);
#17377=VERTEX_POINT('',#78576);
#17378=VERTEX_POINT('',#78578);
#17379=VERTEX_POINT('',#78580);
#17380=VERTEX_POINT('',#78582);
#17381=VERTEX_POINT('',#78584);
#17382=VERTEX_POINT('',#78586);
#17383=VERTEX_POINT('',#78588);
#17384=VERTEX_POINT('',#78590);
#17385=VERTEX_POINT('',#78592);
#17386=VERTEX_POINT('',#78594);
#17387=VERTEX_POINT('',#78596);
#17388=VERTEX_POINT('',#78598);
#17389=VERTEX_POINT('',#78600);
#17390=VERTEX_POINT('',#78602);
#17391=VERTEX_POINT('',#78604);
#17392=VERTEX_POINT('',#78606);
#17393=VERTEX_POINT('',#78608);
#17394=VERTEX_POINT('',#78610);
#17395=VERTEX_POINT('',#78612);
#17396=VERTEX_POINT('',#78614);
#17397=VERTEX_POINT('',#78616);
#17398=VERTEX_POINT('',#78618);
#17399=VERTEX_POINT('',#78620);
#17400=VERTEX_POINT('',#78622);
#17401=VERTEX_POINT('',#78624);
#17402=VERTEX_POINT('',#78626);
#17403=VERTEX_POINT('',#78628);
#17404=VERTEX_POINT('',#78630);
#17405=VERTEX_POINT('',#78632);
#17406=VERTEX_POINT('',#78634);
#17407=VERTEX_POINT('',#78636);
#17408=VERTEX_POINT('',#78638);
#17409=VERTEX_POINT('',#78640);
#17410=VERTEX_POINT('',#78642);
#17411=VERTEX_POINT('',#78644);
#17412=VERTEX_POINT('',#78646);
#17413=VERTEX_POINT('',#78648);
#17414=VERTEX_POINT('',#78650);
#17415=VERTEX_POINT('',#78652);
#17416=VERTEX_POINT('',#78654);
#17417=VERTEX_POINT('',#78656);
#17418=VERTEX_POINT('',#78658);
#17419=VERTEX_POINT('',#78660);
#17420=VERTEX_POINT('',#78662);
#17421=VERTEX_POINT('',#78664);
#17422=VERTEX_POINT('',#78666);
#17423=VERTEX_POINT('',#78668);
#17424=VERTEX_POINT('',#78670);
#17425=VERTEX_POINT('',#78672);
#17426=VERTEX_POINT('',#78674);
#17427=VERTEX_POINT('',#78676);
#17428=VERTEX_POINT('',#78678);
#17429=VERTEX_POINT('',#78680);
#17430=VERTEX_POINT('',#78682);
#17431=VERTEX_POINT('',#78684);
#17432=VERTEX_POINT('',#78686);
#17433=VERTEX_POINT('',#78688);
#17434=VERTEX_POINT('',#78690);
#17435=VERTEX_POINT('',#78692);
#17436=VERTEX_POINT('',#78694);
#17437=VERTEX_POINT('',#78696);
#17438=VERTEX_POINT('',#78698);
#17439=VERTEX_POINT('',#78700);
#17440=VERTEX_POINT('',#78702);
#17441=VERTEX_POINT('',#78704);
#17442=VERTEX_POINT('',#78706);
#17443=VERTEX_POINT('',#78708);
#17444=VERTEX_POINT('',#78710);
#17445=VERTEX_POINT('',#78712);
#17446=VERTEX_POINT('',#78714);
#17447=VERTEX_POINT('',#78716);
#17448=VERTEX_POINT('',#78718);
#17449=VERTEX_POINT('',#78720);
#17450=VERTEX_POINT('',#78722);
#17451=VERTEX_POINT('',#78724);
#17452=VERTEX_POINT('',#78726);
#17453=VERTEX_POINT('',#78728);
#17454=VERTEX_POINT('',#78730);
#17455=VERTEX_POINT('',#78732);
#17456=VERTEX_POINT('',#78734);
#17457=VERTEX_POINT('',#78736);
#17458=VERTEX_POINT('',#78738);
#17459=VERTEX_POINT('',#78740);
#17460=VERTEX_POINT('',#78742);
#17461=VERTEX_POINT('',#78744);
#17462=VERTEX_POINT('',#78746);
#17463=VERTEX_POINT('',#78748);
#17464=VERTEX_POINT('',#78750);
#17465=VERTEX_POINT('',#78752);
#17466=VERTEX_POINT('',#78756);
#17467=VERTEX_POINT('',#78757);
#17468=VERTEX_POINT('',#78762);
#17469=VERTEX_POINT('',#78766);
#17470=VERTEX_POINT('',#78768);
#17471=VERTEX_POINT('',#78775);
#17472=VERTEX_POINT('',#78777);
#17473=VERTEX_POINT('',#78784);
#17474=VERTEX_POINT('',#78786);
#17475=VERTEX_POINT('',#78788);
#17476=VERTEX_POINT('',#78790);
#17477=VERTEX_POINT('',#78792);
#17478=VERTEX_POINT('',#78794);
#17479=VERTEX_POINT('',#78796);
#17480=VERTEX_POINT('',#78798);
#17481=VERTEX_POINT('',#78800);
#17482=VERTEX_POINT('',#78802);
#17483=VERTEX_POINT('',#78804);
#17484=VERTEX_POINT('',#78806);
#17485=VERTEX_POINT('',#78825);
#17486=VERTEX_POINT('',#78826);
#17487=VERTEX_POINT('',#78831);
#17488=VERTEX_POINT('',#78833);
#17489=VERTEX_POINT('',#78835);
#17490=VERTEX_POINT('',#78837);
#17491=VERTEX_POINT('',#78845);
#17492=VERTEX_POINT('',#78846);
#17493=VERTEX_POINT('',#78851);
#17494=VERTEX_POINT('',#78853);
#17495=VERTEX_POINT('',#78855);
#17496=VERTEX_POINT('',#78857);
#17497=VERTEX_POINT('',#78859);
#17498=VERTEX_POINT('',#78866);
#17499=VERTEX_POINT('',#78868);
#17500=VERTEX_POINT('',#78875);
#17501=VERTEX_POINT('',#78877);
#17502=VERTEX_POINT('',#78879);
#17503=VERTEX_POINT('',#78881);
#17504=VERTEX_POINT('',#78883);
#17505=VERTEX_POINT('',#78885);
#17506=VERTEX_POINT('',#78887);
#17507=VERTEX_POINT('',#78889);
#17508=VERTEX_POINT('',#78891);
#17509=VERTEX_POINT('',#78893);
#17510=VERTEX_POINT('',#78895);
#17511=VERTEX_POINT('',#78897);
#17512=VERTEX_POINT('',#78899);
#17513=VERTEX_POINT('',#78927);
#17514=VERTEX_POINT('',#78928);
#17515=VERTEX_POINT('',#78933);
#17516=VERTEX_POINT('',#78935);
#17517=VERTEX_POINT('',#78949);
#17518=VERTEX_POINT('',#78951);
#17519=VERTEX_POINT('',#78955);
#17520=VERTEX_POINT('',#78956);
#17521=VERTEX_POINT('',#78961);
#17522=VERTEX_POINT('',#78963);
#17523=VERTEX_POINT('',#78965);
#17524=VERTEX_POINT('',#78967);
#17525=VERTEX_POINT('',#78986);
#17526=VERTEX_POINT('',#78987);
#17527=VERTEX_POINT('',#78992);
#17528=VERTEX_POINT('',#78994);
#17529=VERTEX_POINT('',#78996);
#17530=VERTEX_POINT('',#78998);
#17531=VERTEX_POINT('',#79000);
#17532=VERTEX_POINT('',#79007);
#17533=VERTEX_POINT('',#79009);
#17534=VERTEX_POINT('',#79016);
#17535=VERTEX_POINT('',#79018);
#17536=VERTEX_POINT('',#79020);
#17537=VERTEX_POINT('',#79022);
#17538=VERTEX_POINT('',#79024);
#17539=VERTEX_POINT('',#79026);
#17540=VERTEX_POINT('',#79028);
#17541=VERTEX_POINT('',#79030);
#17542=VERTEX_POINT('',#79032);
#17543=VERTEX_POINT('',#79034);
#17544=VERTEX_POINT('',#79036);
#17545=VERTEX_POINT('',#79038);
#17546=VERTEX_POINT('',#79040);
#17547=VERTEX_POINT('',#79068);
#17548=VERTEX_POINT('',#79069);
#17549=VERTEX_POINT('',#79074);
#17550=VERTEX_POINT('',#79076);
#17551=VERTEX_POINT('',#79090);
#17552=VERTEX_POINT('',#79092);
#17553=VERTEX_POINT('',#79096);
#17554=VERTEX_POINT('',#79097);
#17555=VERTEX_POINT('',#79102);
#17556=VERTEX_POINT('',#79104);
#17557=VERTEX_POINT('',#79106);
#17558=VERTEX_POINT('',#79108);
#17559=VERTEX_POINT('',#79127);
#17560=VERTEX_POINT('',#79128);
#17561=VERTEX_POINT('',#79133);
#17562=VERTEX_POINT('',#79135);
#17563=VERTEX_POINT('',#79137);
#17564=VERTEX_POINT('',#79139);
#17565=VERTEX_POINT('',#79141);
#17566=VERTEX_POINT('',#79148);
#17567=VERTEX_POINT('',#79150);
#17568=VERTEX_POINT('',#79157);
#17569=VERTEX_POINT('',#79159);
#17570=VERTEX_POINT('',#79161);
#17571=VERTEX_POINT('',#79163);
#17572=VERTEX_POINT('',#79165);
#17573=VERTEX_POINT('',#79167);
#17574=VERTEX_POINT('',#79169);
#17575=VERTEX_POINT('',#79171);
#17576=VERTEX_POINT('',#79173);
#17577=VERTEX_POINT('',#79175);
#17578=VERTEX_POINT('',#79177);
#17579=VERTEX_POINT('',#79179);
#17580=VERTEX_POINT('',#79181);
#17581=VERTEX_POINT('',#79209);
#17582=VERTEX_POINT('',#79210);
#17583=VERTEX_POINT('',#79215);
#17584=VERTEX_POINT('',#79217);
#17585=VERTEX_POINT('',#79231);
#17586=VERTEX_POINT('',#79233);
#17587=VERTEX_POINT('',#79237);
#17588=VERTEX_POINT('',#79238);
#17589=VERTEX_POINT('',#79243);
#17590=VERTEX_POINT('',#79245);
#17591=VERTEX_POINT('',#79247);
#17592=VERTEX_POINT('',#79249);
#17593=VERTEX_POINT('',#79268);
#17594=VERTEX_POINT('',#79269);
#17595=VERTEX_POINT('',#79274);
#17596=VERTEX_POINT('',#79276);
#17597=VERTEX_POINT('',#79278);
#17598=VERTEX_POINT('',#79280);
#17599=VERTEX_POINT('',#79282);
#17600=VERTEX_POINT('',#79289);
#17601=VERTEX_POINT('',#79291);
#17602=VERTEX_POINT('',#79298);
#17603=VERTEX_POINT('',#79300);
#17604=VERTEX_POINT('',#79302);
#17605=VERTEX_POINT('',#79304);
#17606=VERTEX_POINT('',#79306);
#17607=VERTEX_POINT('',#79308);
#17608=VERTEX_POINT('',#79310);
#17609=VERTEX_POINT('',#79312);
#17610=VERTEX_POINT('',#79314);
#17611=VERTEX_POINT('',#79316);
#17612=VERTEX_POINT('',#79318);
#17613=VERTEX_POINT('',#79320);
#17614=VERTEX_POINT('',#79322);
#17615=VERTEX_POINT('',#79350);
#17616=VERTEX_POINT('',#79351);
#17617=VERTEX_POINT('',#79356);
#17618=VERTEX_POINT('',#79358);
#17619=VERTEX_POINT('',#79372);
#17620=VERTEX_POINT('',#79374);
#17621=VERTEX_POINT('',#79378);
#17622=VERTEX_POINT('',#79379);
#17623=VERTEX_POINT('',#79384);
#17624=VERTEX_POINT('',#79386);
#17625=VERTEX_POINT('',#79388);
#17626=VERTEX_POINT('',#79390);
#17627=VERTEX_POINT('',#79409);
#17628=VERTEX_POINT('',#79410);
#17629=VERTEX_POINT('',#79415);
#17630=VERTEX_POINT('',#79417);
#17631=VERTEX_POINT('',#79419);
#17632=VERTEX_POINT('',#79421);
#17633=VERTEX_POINT('',#79423);
#17634=VERTEX_POINT('',#79430);
#17635=VERTEX_POINT('',#79432);
#17636=VERTEX_POINT('',#79439);
#17637=VERTEX_POINT('',#79441);
#17638=VERTEX_POINT('',#79443);
#17639=VERTEX_POINT('',#79445);
#17640=VERTEX_POINT('',#79447);
#17641=VERTEX_POINT('',#79449);
#17642=VERTEX_POINT('',#79451);
#17643=VERTEX_POINT('',#79453);
#17644=VERTEX_POINT('',#79455);
#17645=VERTEX_POINT('',#79457);
#17646=VERTEX_POINT('',#79459);
#17647=VERTEX_POINT('',#79461);
#17648=VERTEX_POINT('',#79463);
#17649=VERTEX_POINT('',#79505);
#17650=VERTEX_POINT('',#79506);
#17651=VERTEX_POINT('',#79508);
#17652=VERTEX_POINT('',#79514);
#17653=VERTEX_POINT('',#79528);
#17654=VERTEX_POINT('',#79561);
#17655=VERTEX_POINT('',#79568);
#17656=VERTEX_POINT('',#79608);
#17657=VERTEX_POINT('',#79615);
#17658=VERTEX_POINT('',#79617);
#17659=VERTEX_POINT('',#79624);
#17660=VERTEX_POINT('',#79626);
#17661=VERTEX_POINT('',#79670);
#17662=VERTEX_POINT('',#79671);
#17663=VERTEX_POINT('',#79673);
#17664=VERTEX_POINT('',#79679);
#17665=VERTEX_POINT('',#79733);
#17666=VERTEX_POINT('',#79737);
#17667=VERTEX_POINT('',#79745);
#17668=VERTEX_POINT('',#79749);
#17669=VERTEX_POINT('',#79812);
#17670=VERTEX_POINT('',#79813);
#17671=VERTEX_POINT('',#79832);
#17672=VERTEX_POINT('',#79865);
#17673=VERTEX_POINT('',#79874);
#17674=VERTEX_POINT('',#79876);
#17675=VERTEX_POINT('',#79904);
#17676=VERTEX_POINT('',#79910);
#17677=VERTEX_POINT('',#79918);
#17678=VERTEX_POINT('',#79974);
#17679=VERTEX_POINT('',#79975);
#17680=VERTEX_POINT('',#79977);
#17681=VERTEX_POINT('',#79983);
#17682=VERTEX_POINT('',#79995);
#17683=VERTEX_POINT('',#79997);
#17684=VERTEX_POINT('',#80005);
#17685=VERTEX_POINT('',#80049);
#17686=VERTEX_POINT('',#80056);
#17687=VERTEX_POINT('',#80130);
#17688=VERTEX_POINT('',#80132);
#17689=VERTEX_POINT('',#80179);
#17690=VERTEX_POINT('',#80192);
#17691=VERTEX_POINT('',#80194);
#17692=VERTEX_POINT('',#80202);
#17693=VERTEX_POINT('',#80257);
#17694=VERTEX_POINT('',#80347);
#17695=VERTEX_POINT('',#80349);
#17696=VERTEX_POINT('',#80355);
#17697=VERTEX_POINT('',#80494);
#17698=VERTEX_POINT('',#80506);
#17699=VERTEX_POINT('',#80590);
#17700=VERTEX_POINT('',#80599);
#17701=VERTEX_POINT('',#80661);
#17702=VERTEX_POINT('',#80666);
#17703=VERTEX_POINT('',#80711);
#17704=VERTEX_POINT('',#80717);
#17705=VERTEX_POINT('',#80760);
#17706=VERTEX_POINT('',#80767);
#17707=VERTEX_POINT('',#80817);
#17708=VERTEX_POINT('',#80836);
#17709=VERTEX_POINT('',#80838);
#17710=VERTEX_POINT('',#80877);
#17711=VERTEX_POINT('',#80895);
#17712=VERTEX_POINT('',#80914);
#22418=EDGE_CURVE('',#17301,#17302,#8393,.T.);
#22419=EDGE_CURVE('',#17302,#17303,#11499,.T.);
#22420=EDGE_CURVE('',#17303,#17304,#8394,.T.);
#22421=EDGE_CURVE('',#17304,#17301,#11500,.T.);
#22422=EDGE_CURVE('',#17301,#17305,#11501,.T.);
#22423=EDGE_CURVE('',#17306,#17305,#8395,.T.);
#22424=EDGE_CURVE('',#17306,#17307,#11502,.T.);
#22425=EDGE_CURVE('',#17307,#17308,#11503,.T.);
#22426=EDGE_CURVE('',#17302,#17308,#11504,.T.);
#22427=EDGE_CURVE('',#17304,#17309,#11505,.T.);
#22428=EDGE_CURVE('',#17305,#17309,#11506,.T.);
#22429=EDGE_CURVE('',#17309,#17310,#8396,.T.);
#22430=EDGE_CURVE('',#17310,#17306,#11507,.T.);
#22431=EDGE_CURVE('',#17311,#17312,#8397,.T.);
#22432=EDGE_CURVE('',#17312,#17313,#11508,.T.);
#22433=EDGE_CURVE('',#17313,#17314,#8398,.T.);
#22434=EDGE_CURVE('',#17314,#17311,#11509,.T.);
#22435=EDGE_CURVE('',#17314,#17315,#11510,.T.);
#22436=EDGE_CURVE('',#17316,#17315,#11511,.T.);
#22437=EDGE_CURVE('',#17311,#17316,#11512,.T.);
#22438=EDGE_CURVE('',#17317,#17318,#8399,.T.);
#22439=EDGE_CURVE('',#17319,#17317,#10135,.T.);
#22440=EDGE_CURVE('',#17320,#17319,#8400,.T.);
#22441=EDGE_CURVE('',#17321,#17320,#10136,.T.);
#22442=EDGE_CURVE('',#17322,#17321,#8401,.T.);
#22443=EDGE_CURVE('',#17323,#17322,#10137,.T.);
#22444=EDGE_CURVE('',#17324,#17323,#8402,.T.);
#22445=EDGE_CURVE('',#17325,#17324,#10138,.T.);
#22446=EDGE_CURVE('',#17326,#17325,#8403,.T.);
#22447=EDGE_CURVE('',#17327,#17326,#10139,.T.);
#22448=EDGE_CURVE('',#17328,#17327,#8404,.T.);
#22449=EDGE_CURVE('',#17318,#17328,#10140,.T.);
#22450=EDGE_CURVE('',#17329,#17303,#11513,.T.);
#22451=EDGE_CURVE('',#17329,#17315,#8405,.T.);
#22452=EDGE_CURVE('',#17330,#17313,#11514,.T.);
#22453=EDGE_CURVE('',#17331,#17330,#8406,.T.);
#22454=EDGE_CURVE('',#17332,#17331,#11515,.T.);
#22455=EDGE_CURVE('',#17332,#17333,#8407,.T.);
#22456=EDGE_CURVE('',#17334,#17333,#11516,.T.);
#22457=EDGE_CURVE('',#17335,#17334,#8408,.T.);
#22458=EDGE_CURVE('',#17336,#17335,#11517,.T.);
#22459=EDGE_CURVE('',#17337,#17336,#8409,.T.);
#22460=EDGE_CURVE('',#17338,#17337,#11518,.T.);
#22461=EDGE_CURVE('',#17338,#17339,#8410,.T.);
#22462=EDGE_CURVE('',#17340,#17339,#11519,.T.);
#22463=EDGE_CURVE('',#17341,#17340,#8411,.T.);
#22464=EDGE_CURVE('',#17342,#17341,#11520,.T.);
#22465=EDGE_CURVE('',#17343,#17342,#8412,.T.);
#22466=EDGE_CURVE('',#17344,#17343,#11521,.T.);
#22467=EDGE_CURVE('',#17344,#17345,#8413,.T.);
#22468=EDGE_CURVE('',#17346,#17345,#11522,.T.);
#22469=EDGE_CURVE('',#17347,#17346,#8414,.T.);
#22470=EDGE_CURVE('',#17348,#17347,#11523,.T.);
#22471=EDGE_CURVE('',#17349,#17348,#8415,.T.);
#22472=EDGE_CURVE('',#17350,#17349,#11524,.T.);
#22473=EDGE_CURVE('',#17350,#17351,#8416,.T.);
#22474=EDGE_CURVE('',#17352,#17351,#11525,.T.);
#22475=EDGE_CURVE('',#17353,#17352,#8417,.T.);
#22476=EDGE_CURVE('',#17354,#17353,#11526,.T.);
#22477=EDGE_CURVE('',#17355,#17354,#8418,.T.);
#22478=EDGE_CURVE('',#17356,#17355,#11527,.T.);
#22479=EDGE_CURVE('',#17356,#17357,#8419,.T.);
#22480=EDGE_CURVE('',#17358,#17357,#11528,.T.);
#22481=EDGE_CURVE('',#17359,#17358,#8420,.T.);
#22482=EDGE_CURVE('',#17360,#17359,#11529,.T.);
#22483=EDGE_CURVE('',#17361,#17360,#8421,.T.);
#22484=EDGE_CURVE('',#17362,#17361,#11530,.T.);
#22485=EDGE_CURVE('',#17362,#17363,#8422,.T.);
#22486=EDGE_CURVE('',#17364,#17363,#11531,.T.);
#22487=EDGE_CURVE('',#17365,#17364,#8423,.T.);
#22488=EDGE_CURVE('',#17366,#17365,#11532,.T.);
#22489=EDGE_CURVE('',#17367,#17366,#8424,.T.);
#22490=EDGE_CURVE('',#17368,#17367,#11533,.T.);
#22491=EDGE_CURVE('',#17368,#17369,#8425,.T.);
#22492=EDGE_CURVE('',#17370,#17369,#11534,.T.);
#22493=EDGE_CURVE('',#17371,#17370,#8426,.T.);
#22494=EDGE_CURVE('',#17372,#17371,#11535,.T.);
#22495=EDGE_CURVE('',#17373,#17372,#8427,.T.);
#22496=EDGE_CURVE('',#17374,#17373,#11536,.T.);
#22497=EDGE_CURVE('',#17374,#17375,#8428,.T.);
#22498=EDGE_CURVE('',#17376,#17375,#11537,.T.);
#22499=EDGE_CURVE('',#17377,#17376,#8429,.T.);
#22500=EDGE_CURVE('',#17378,#17377,#11538,.T.);
#22501=EDGE_CURVE('',#17379,#17378,#8430,.T.);
#22502=EDGE_CURVE('',#17380,#17379,#11539,.T.);
#22503=EDGE_CURVE('',#17380,#17381,#8431,.T.);
#22504=EDGE_CURVE('',#17382,#17381,#11540,.T.);
#22505=EDGE_CURVE('',#17383,#17382,#8432,.T.);
#22506=EDGE_CURVE('',#17384,#17383,#11541,.T.);
#22507=EDGE_CURVE('',#17385,#17384,#8433,.T.);
#22508=EDGE_CURVE('',#17386,#17385,#11542,.T.);
#22509=EDGE_CURVE('',#17386,#17387,#8434,.T.);
#22510=EDGE_CURVE('',#17388,#17387,#11543,.T.);
#22511=EDGE_CURVE('',#17389,#17388,#8435,.T.);
#22512=EDGE_CURVE('',#17390,#17389,#11544,.T.);
#22513=EDGE_CURVE('',#17391,#17390,#8436,.T.);
#22514=EDGE_CURVE('',#17392,#17391,#11545,.T.);
#22515=EDGE_CURVE('',#17392,#17393,#8437,.T.);
#22516=EDGE_CURVE('',#17394,#17393,#11546,.T.);
#22517=EDGE_CURVE('',#17395,#17394,#8438,.T.);
#22518=EDGE_CURVE('',#17396,#17395,#11547,.T.);
#22519=EDGE_CURVE('',#17397,#17396,#8439,.T.);
#22520=EDGE_CURVE('',#17398,#17397,#11548,.T.);
#22521=EDGE_CURVE('',#17398,#17399,#8440,.T.);
#22522=EDGE_CURVE('',#17400,#17399,#11549,.T.);
#22523=EDGE_CURVE('',#17401,#17400,#8441,.T.);
#22524=EDGE_CURVE('',#17402,#17401,#11550,.T.);
#22525=EDGE_CURVE('',#17403,#17402,#8442,.T.);
#22526=EDGE_CURVE('',#17404,#17403,#11551,.T.);
#22527=EDGE_CURVE('',#17404,#17405,#8443,.T.);
#22528=EDGE_CURVE('',#17406,#17405,#11552,.T.);
#22529=EDGE_CURVE('',#17407,#17406,#8444,.T.);
#22530=EDGE_CURVE('',#17408,#17407,#11553,.T.);
#22531=EDGE_CURVE('',#17409,#17408,#8445,.T.);
#22532=EDGE_CURVE('',#17410,#17409,#11554,.T.);
#22533=EDGE_CURVE('',#17410,#17411,#8446,.T.);
#22534=EDGE_CURVE('',#17412,#17411,#11555,.T.);
#22535=EDGE_CURVE('',#17413,#17412,#8447,.T.);
#22536=EDGE_CURVE('',#17414,#17413,#11556,.T.);
#22537=EDGE_CURVE('',#17415,#17414,#8448,.T.);
#22538=EDGE_CURVE('',#17416,#17415,#11557,.T.);
#22539=EDGE_CURVE('',#17416,#17417,#8449,.T.);
#22540=EDGE_CURVE('',#17418,#17417,#11558,.T.);
#22541=EDGE_CURVE('',#17419,#17418,#8450,.T.);
#22542=EDGE_CURVE('',#17420,#17419,#11559,.T.);
#22543=EDGE_CURVE('',#17421,#17420,#8451,.T.);
#22544=EDGE_CURVE('',#17422,#17421,#11560,.T.);
#22545=EDGE_CURVE('',#17422,#17423,#8452,.T.);
#22546=EDGE_CURVE('',#17424,#17423,#11561,.T.);
#22547=EDGE_CURVE('',#17425,#17424,#8453,.T.);
#22548=EDGE_CURVE('',#17426,#17425,#11562,.T.);
#22549=EDGE_CURVE('',#17427,#17426,#8454,.T.);
#22550=EDGE_CURVE('',#17428,#17427,#11563,.T.);
#22551=EDGE_CURVE('',#17428,#17429,#8455,.T.);
#22552=EDGE_CURVE('',#17430,#17429,#11564,.T.);
#22553=EDGE_CURVE('',#17431,#17430,#8456,.T.);
#22554=EDGE_CURVE('',#17432,#17431,#11565,.T.);
#22555=EDGE_CURVE('',#17433,#17432,#8457,.T.);
#22556=EDGE_CURVE('',#17434,#17433,#11566,.T.);
#22557=EDGE_CURVE('',#17434,#17435,#8458,.T.);
#22558=EDGE_CURVE('',#17436,#17435,#11567,.T.);
#22559=EDGE_CURVE('',#17437,#17436,#8459,.T.);
#22560=EDGE_CURVE('',#17438,#17437,#11568,.T.);
#22561=EDGE_CURVE('',#17439,#17438,#8460,.T.);
#22562=EDGE_CURVE('',#17440,#17439,#11569,.T.);
#22563=EDGE_CURVE('',#17440,#17441,#8461,.T.);
#22564=EDGE_CURVE('',#17442,#17441,#11570,.T.);
#22565=EDGE_CURVE('',#17443,#17442,#8462,.T.);
#22566=EDGE_CURVE('',#17444,#17443,#11571,.T.);
#22567=EDGE_CURVE('',#17445,#17444,#8463,.T.);
#22568=EDGE_CURVE('',#17446,#17445,#11572,.T.);
#22569=EDGE_CURVE('',#17446,#17447,#8464,.T.);
#22570=EDGE_CURVE('',#17448,#17447,#11573,.T.);
#22571=EDGE_CURVE('',#17449,#17448,#8465,.T.);
#22572=EDGE_CURVE('',#17450,#17449,#11574,.T.);
#22573=EDGE_CURVE('',#17451,#17450,#8466,.T.);
#22574=EDGE_CURVE('',#17452,#17451,#11575,.T.);
#22575=EDGE_CURVE('',#17452,#17453,#8467,.T.);
#22576=EDGE_CURVE('',#17454,#17453,#11576,.T.);
#22577=EDGE_CURVE('',#17455,#17454,#8468,.T.);
#22578=EDGE_CURVE('',#17456,#17455,#11577,.T.);
#22579=EDGE_CURVE('',#17457,#17456,#8469,.T.);
#22580=EDGE_CURVE('',#17458,#17457,#11578,.T.);
#22581=EDGE_CURVE('',#17458,#17459,#8470,.T.);
#22582=EDGE_CURVE('',#17460,#17459,#11579,.T.);
#22583=EDGE_CURVE('',#17461,#17460,#8471,.T.);
#22584=EDGE_CURVE('',#17462,#17461,#11580,.T.);
#22585=EDGE_CURVE('',#17463,#17462,#8472,.T.);
#22586=EDGE_CURVE('',#17464,#17463,#11581,.T.);
#22587=EDGE_CURVE('',#17464,#17465,#8473,.T.);
#22588=EDGE_CURVE('',#17310,#17465,#11582,.T.);
#22589=EDGE_CURVE('',#17466,#17467,#8474,.T.);
#22590=EDGE_CURVE('',#17467,#17331,#11583,.T.);
#22591=EDGE_CURVE('',#17330,#17466,#11584,.T.);
#22592=EDGE_CURVE('',#17468,#17467,#11585,.T.);
#22593=EDGE_CURVE('',#17332,#17468,#11586,.T.);
#22594=EDGE_CURVE('',#17469,#17316,#8475,.T.);
#22595=EDGE_CURVE('',#17470,#17469,#10141,.T.);
#22596=EDGE_CURVE('',#17471,#17470,#8476,.T.);
#22597=EDGE_CURVE('',#17472,#17471,#10142,.T.);
#22598=EDGE_CURVE('',#17473,#17472,#8477,.T.);
#22599=EDGE_CURVE('',#17473,#17474,#11587,.T.);
#22600=EDGE_CURVE('',#17475,#17474,#8478,.T.);
#22601=EDGE_CURVE('',#17475,#17476,#11588,.T.);
#22602=EDGE_CURVE('',#17477,#17476,#8479,.T.);
#22603=EDGE_CURVE('',#17477,#17478,#11589,.T.);
#22604=EDGE_CURVE('',#17479,#17478,#8480,.T.);
#22605=EDGE_CURVE('',#17479,#17480,#11590,.T.);
#22606=EDGE_CURVE('',#17481,#17480,#8481,.T.);
#22607=EDGE_CURVE('',#17481,#17482,#11591,.T.);
#22608=EDGE_CURVE('',#17483,#17482,#8482,.T.);
#22609=EDGE_CURVE('',#17483,#17484,#11592,.T.);
#22610=EDGE_CURVE('',#17468,#17484,#8483,.T.);
#22611=EDGE_CURVE('',#17466,#17312,#11593,.T.);
#22612=EDGE_CURVE('',#17482,#17335,#11594,.T.);
#22613=EDGE_CURVE('',#17334,#17483,#11595,.T.);
#22614=EDGE_CURVE('',#17336,#17481,#11596,.T.);
#22615=EDGE_CURVE('',#17480,#17337,#11597,.T.);
#22616=EDGE_CURVE('',#17474,#17343,#11598,.T.);
#22617=EDGE_CURVE('',#17342,#17475,#11599,.T.);
#22618=EDGE_CURVE('',#17476,#17341,#11600,.T.);
#22619=EDGE_CURVE('',#17340,#17477,#11601,.T.);
#22620=EDGE_CURVE('',#17485,#17486,#8484,.T.);
#22621=EDGE_CURVE('',#17486,#17349,#11602,.T.);
#22622=EDGE_CURVE('',#17348,#17485,#11603,.T.);
#22623=EDGE_CURVE('',#17485,#17487,#11604,.T.);
#22624=EDGE_CURVE('',#17488,#17487,#8485,.T.);
#22625=EDGE_CURVE('',#17488,#17489,#11605,.T.);
#22626=EDGE_CURVE('',#17489,#17490,#11606,.T.);
#22627=EDGE_CURVE('',#17486,#17490,#11607,.T.);
#22628=EDGE_CURVE('',#17487,#17347,#11608,.T.);
#22629=EDGE_CURVE('',#17346,#17488,#11609,.T.);
#22630=EDGE_CURVE('',#17491,#17492,#8486,.T.);
#22631=EDGE_CURVE('',#17492,#17355,#11610,.T.);
#22632=EDGE_CURVE('',#17354,#17491,#11611,.T.);
#22633=EDGE_CURVE('',#17491,#17493,#11612,.T.);
#22634=EDGE_CURVE('',#17494,#17493,#8487,.T.);
#22635=EDGE_CURVE('',#17494,#17495,#11613,.T.);
#22636=EDGE_CURVE('',#17496,#17495,#8488,.T.);
#22637=EDGE_CURVE('',#17497,#17496,#10143,.T.);
#22638=EDGE_CURVE('',#17498,#17497,#8489,.T.);
#22639=EDGE_CURVE('',#17499,#17498,#10144,.T.);
#22640=EDGE_CURVE('',#17500,#17499,#8490,.T.);
#22641=EDGE_CURVE('',#17500,#17501,#11614,.T.);
#22642=EDGE_CURVE('',#17502,#17501,#8491,.T.);
#22643=EDGE_CURVE('',#17502,#17503,#11615,.T.);
#22644=EDGE_CURVE('',#17504,#17503,#8492,.T.);
#22645=EDGE_CURVE('',#17504,#17505,#11616,.T.);
#22646=EDGE_CURVE('',#17506,#17505,#8493,.T.);
#22647=EDGE_CURVE('',#17506,#17507,#11617,.T.);
#22648=EDGE_CURVE('',#17508,#17507,#8494,.T.);
#22649=EDGE_CURVE('',#17508,#17509,#11618,.T.);
#22650=EDGE_CURVE('',#17510,#17509,#8495,.T.);
#22651=EDGE_CURVE('',#17510,#17511,#11619,.T.);
#22652=EDGE_CURVE('',#17512,#17511,#8496,.T.);
#22653=EDGE_CURVE('',#17512,#17492,#11620,.T.);
#22654=EDGE_CURVE('',#17493,#17353,#11621,.T.);
#22655=EDGE_CURVE('',#17352,#17494,#11622,.T.);
#22656=EDGE_CURVE('',#17509,#17359,#11623,.T.);
#22657=EDGE_CURVE('',#17358,#17510,#11624,.T.);
#22658=EDGE_CURVE('',#17511,#17357,#11625,.T.);
#22659=EDGE_CURVE('',#17507,#17361,#11626,.T.);
#22660=EDGE_CURVE('',#17360,#17508,#11627,.T.);
#22661=EDGE_CURVE('',#17362,#17506,#11628,.T.);
#22662=EDGE_CURVE('',#17503,#17365,#11629,.T.);
#22663=EDGE_CURVE('',#17364,#17504,#11630,.T.);
#22664=EDGE_CURVE('',#17505,#17363,#11631,.T.);
#22665=EDGE_CURVE('',#17501,#17367,#11632,.T.);
#22666=EDGE_CURVE('',#17366,#17502,#11633,.T.);
#22667=EDGE_CURVE('',#17368,#17500,#11634,.T.);
#22668=EDGE_CURVE('',#17513,#17514,#8497,.T.);
#22669=EDGE_CURVE('',#17514,#17371,#11635,.T.);
#22670=EDGE_CURVE('',#17370,#17513,#11636,.T.);
#22671=EDGE_CURVE('',#17515,#17369,#11637,.T.);
#22672=EDGE_CURVE('',#17516,#17515,#10145,.F.);
#22673=EDGE_CURVE('',#17517,#17516,#8498,.T.);
#22674=EDGE_CURVE('',#17517,#17518,#11638,.T.);
#22675=EDGE_CURVE('',#17513,#17518,#11639,.T.);
#22676=EDGE_CURVE('',#17519,#17520,#8499,.T.);
#22677=EDGE_CURVE('',#17520,#17373,#11640,.T.);
#22678=EDGE_CURVE('',#17372,#17519,#11641,.T.);
#22679=EDGE_CURVE('',#17520,#17521,#11642,.T.);
#22680=EDGE_CURVE('',#17522,#17521,#11643,.T.);
#22681=EDGE_CURVE('',#17523,#17522,#8500,.T.);
#22682=EDGE_CURVE('',#17523,#17524,#10146,.T.);
#22683=EDGE_CURVE('',#17374,#17524,#11644,.T.);
#22684=EDGE_CURVE('',#17518,#17521,#11645,.T.);
#22685=EDGE_CURVE('',#17519,#17514,#11646,.T.);
#22686=EDGE_CURVE('',#17525,#17526,#8501,.T.);
#22687=EDGE_CURVE('',#17526,#17379,#11647,.T.);
#22688=EDGE_CURVE('',#17378,#17525,#11648,.T.);
#22689=EDGE_CURVE('',#17525,#17527,#11649,.T.);
#22690=EDGE_CURVE('',#17528,#17527,#8502,.T.);
#22691=EDGE_CURVE('',#17528,#17529,#11650,.T.);
#22692=EDGE_CURVE('',#17530,#17529,#8503,.T.);
#22693=EDGE_CURVE('',#17531,#17530,#10147,.T.);
#22694=EDGE_CURVE('',#17532,#17531,#8504,.T.);
#22695=EDGE_CURVE('',#17533,#17532,#10148,.T.);
#22696=EDGE_CURVE('',#17534,#17533,#8505,.T.);
#22697=EDGE_CURVE('',#17534,#17535,#11651,.T.);
#22698=EDGE_CURVE('',#17536,#17535,#8506,.T.);
#22699=EDGE_CURVE('',#17536,#17537,#11652,.T.);
#22700=EDGE_CURVE('',#17538,#17537,#8507,.T.);
#22701=EDGE_CURVE('',#17538,#17539,#11653,.T.);
#22702=EDGE_CURVE('',#17540,#17539,#8508,.T.);
#22703=EDGE_CURVE('',#17540,#17541,#11654,.T.);
#22704=EDGE_CURVE('',#17542,#17541,#8509,.T.);
#22705=EDGE_CURVE('',#17542,#17543,#11655,.T.);
#22706=EDGE_CURVE('',#17544,#17543,#8510,.T.);
#22707=EDGE_CURVE('',#17544,#17545,#11656,.T.);
#22708=EDGE_CURVE('',#17546,#17545,#8511,.T.);
#22709=EDGE_CURVE('',#17546,#17526,#11657,.T.);
#22710=EDGE_CURVE('',#17527,#17377,#11658,.T.);
#22711=EDGE_CURVE('',#17376,#17528,#11659,.T.);
#22712=EDGE_CURVE('',#17543,#17383,#11660,.T.);
#22713=EDGE_CURVE('',#17382,#17544,#11661,.T.);
#22714=EDGE_CURVE('',#17545,#17381,#11662,.T.);
#22715=EDGE_CURVE('',#17541,#17385,#11663,.T.);
#22716=EDGE_CURVE('',#17384,#17542,#11664,.T.);
#22717=EDGE_CURVE('',#17386,#17540,#11665,.T.);
#22718=EDGE_CURVE('',#17537,#17389,#11666,.T.);
#22719=EDGE_CURVE('',#17388,#17538,#11667,.T.);
#22720=EDGE_CURVE('',#17539,#17387,#11668,.T.);
#22721=EDGE_CURVE('',#17535,#17391,#11669,.T.);
#22722=EDGE_CURVE('',#17390,#17536,#11670,.T.);
#22723=EDGE_CURVE('',#17392,#17534,#11671,.T.);
#22724=EDGE_CURVE('',#17547,#17548,#8512,.T.);
#22725=EDGE_CURVE('',#17548,#17395,#11672,.T.);
#22726=EDGE_CURVE('',#17394,#17547,#11673,.T.);
#22727=EDGE_CURVE('',#17549,#17393,#11674,.T.);
#22728=EDGE_CURVE('',#17550,#17549,#10149,.F.);
#22729=EDGE_CURVE('',#17551,#17550,#8513,.T.);
#22730=EDGE_CURVE('',#17551,#17552,#11675,.T.);
#22731=EDGE_CURVE('',#17547,#17552,#11676,.T.);
#22732=EDGE_CURVE('',#17553,#17554,#8514,.T.);
#22733=EDGE_CURVE('',#17554,#17397,#11677,.T.);
#22734=EDGE_CURVE('',#17396,#17553,#11678,.T.);
#22735=EDGE_CURVE('',#17554,#17555,#11679,.T.);
#22736=EDGE_CURVE('',#17556,#17555,#11680,.T.);
#22737=EDGE_CURVE('',#17557,#17556,#8515,.T.);
#22738=EDGE_CURVE('',#17557,#17558,#10150,.T.);
#22739=EDGE_CURVE('',#17398,#17558,#11681,.T.);
#22740=EDGE_CURVE('',#17552,#17555,#11682,.T.);
#22741=EDGE_CURVE('',#17553,#17548,#11683,.T.);
#22742=EDGE_CURVE('',#17559,#17560,#8516,.T.);
#22743=EDGE_CURVE('',#17560,#17403,#11684,.T.);
#22744=EDGE_CURVE('',#17402,#17559,#11685,.T.);
#22745=EDGE_CURVE('',#17559,#17561,#11686,.T.);
#22746=EDGE_CURVE('',#17562,#17561,#8517,.T.);
#22747=EDGE_CURVE('',#17562,#17563,#11687,.T.);
#22748=EDGE_CURVE('',#17564,#17563,#8518,.T.);
#22749=EDGE_CURVE('',#17565,#17564,#10151,.T.);
#22750=EDGE_CURVE('',#17566,#17565,#8519,.T.);
#22751=EDGE_CURVE('',#17567,#17566,#10152,.T.);
#22752=EDGE_CURVE('',#17568,#17567,#8520,.T.);
#22753=EDGE_CURVE('',#17568,#17569,#11688,.T.);
#22754=EDGE_CURVE('',#17570,#17569,#8521,.T.);
#22755=EDGE_CURVE('',#17570,#17571,#11689,.T.);
#22756=EDGE_CURVE('',#17572,#17571,#8522,.T.);
#22757=EDGE_CURVE('',#17572,#17573,#11690,.T.);
#22758=EDGE_CURVE('',#17574,#17573,#8523,.T.);
#22759=EDGE_CURVE('',#17574,#17575,#11691,.T.);
#22760=EDGE_CURVE('',#17576,#17575,#8524,.T.);
#22761=EDGE_CURVE('',#17576,#17577,#11692,.T.);
#22762=EDGE_CURVE('',#17578,#17577,#8525,.T.);
#22763=EDGE_CURVE('',#17578,#17579,#11693,.T.);
#22764=EDGE_CURVE('',#17580,#17579,#8526,.T.);
#22765=EDGE_CURVE('',#17580,#17560,#11694,.T.);
#22766=EDGE_CURVE('',#17561,#17401,#11695,.T.);
#22767=EDGE_CURVE('',#17400,#17562,#11696,.T.);
#22768=EDGE_CURVE('',#17577,#17407,#11697,.T.);
#22769=EDGE_CURVE('',#17406,#17578,#11698,.T.);
#22770=EDGE_CURVE('',#17579,#17405,#11699,.T.);
#22771=EDGE_CURVE('',#17575,#17409,#11700,.T.);
#22772=EDGE_CURVE('',#17408,#17576,#11701,.T.);
#22773=EDGE_CURVE('',#17410,#17574,#11702,.T.);
#22774=EDGE_CURVE('',#17571,#17413,#11703,.T.);
#22775=EDGE_CURVE('',#17412,#17572,#11704,.T.);
#22776=EDGE_CURVE('',#17573,#17411,#11705,.T.);
#22777=EDGE_CURVE('',#17569,#17415,#11706,.T.);
#22778=EDGE_CURVE('',#17414,#17570,#11707,.T.);
#22779=EDGE_CURVE('',#17416,#17568,#11708,.T.);
#22780=EDGE_CURVE('',#17581,#17582,#8527,.T.);
#22781=EDGE_CURVE('',#17582,#17419,#11709,.T.);
#22782=EDGE_CURVE('',#17418,#17581,#11710,.T.);
#22783=EDGE_CURVE('',#17583,#17417,#11711,.T.);
#22784=EDGE_CURVE('',#17584,#17583,#10153,.F.);
#22785=EDGE_CURVE('',#17585,#17584,#8528,.T.);
#22786=EDGE_CURVE('',#17585,#17586,#11712,.T.);
#22787=EDGE_CURVE('',#17581,#17586,#11713,.T.);
#22788=EDGE_CURVE('',#17587,#17588,#8529,.T.);
#22789=EDGE_CURVE('',#17588,#17421,#11714,.T.);
#22790=EDGE_CURVE('',#17420,#17587,#11715,.T.);
#22791=EDGE_CURVE('',#17588,#17589,#11716,.T.);
#22792=EDGE_CURVE('',#17590,#17589,#11717,.T.);
#22793=EDGE_CURVE('',#17591,#17590,#8530,.T.);
#22794=EDGE_CURVE('',#17591,#17592,#10154,.T.);
#22795=EDGE_CURVE('',#17422,#17592,#11718,.T.);
#22796=EDGE_CURVE('',#17586,#17589,#11719,.T.);
#22797=EDGE_CURVE('',#17587,#17582,#11720,.T.);
#22798=EDGE_CURVE('',#17593,#17594,#8531,.T.);
#22799=EDGE_CURVE('',#17594,#17427,#11721,.T.);
#22800=EDGE_CURVE('',#17426,#17593,#11722,.T.);
#22801=EDGE_CURVE('',#17593,#17595,#11723,.T.);
#22802=EDGE_CURVE('',#17596,#17595,#8532,.T.);
#22803=EDGE_CURVE('',#17596,#17597,#11724,.T.);
#22804=EDGE_CURVE('',#17598,#17597,#8533,.T.);
#22805=EDGE_CURVE('',#17599,#17598,#10155,.T.);
#22806=EDGE_CURVE('',#17600,#17599,#8534,.T.);
#22807=EDGE_CURVE('',#17601,#17600,#10156,.T.);
#22808=EDGE_CURVE('',#17602,#17601,#8535,.T.);
#22809=EDGE_CURVE('',#17602,#17603,#11725,.T.);
#22810=EDGE_CURVE('',#17604,#17603,#8536,.T.);
#22811=EDGE_CURVE('',#17604,#17605,#11726,.T.);
#22812=EDGE_CURVE('',#17606,#17605,#8537,.T.);
#22813=EDGE_CURVE('',#17606,#17607,#11727,.T.);
#22814=EDGE_CURVE('',#17608,#17607,#8538,.T.);
#22815=EDGE_CURVE('',#17608,#17609,#11728,.T.);
#22816=EDGE_CURVE('',#17610,#17609,#8539,.T.);
#22817=EDGE_CURVE('',#17610,#17611,#11729,.T.);
#22818=EDGE_CURVE('',#17612,#17611,#8540,.T.);
#22819=EDGE_CURVE('',#17612,#17613,#11730,.T.);
#22820=EDGE_CURVE('',#17614,#17613,#8541,.T.);
#22821=EDGE_CURVE('',#17614,#17594,#11731,.T.);
#22822=EDGE_CURVE('',#17595,#17425,#11732,.T.);
#22823=EDGE_CURVE('',#17424,#17596,#11733,.T.);
#22824=EDGE_CURVE('',#17611,#17431,#11734,.T.);
#22825=EDGE_CURVE('',#17430,#17612,#11735,.T.);
#22826=EDGE_CURVE('',#17613,#17429,#11736,.T.);
#22827=EDGE_CURVE('',#17609,#17433,#11737,.T.);
#22828=EDGE_CURVE('',#17432,#17610,#11738,.T.);
#22829=EDGE_CURVE('',#17434,#17608,#11739,.T.);
#22830=EDGE_CURVE('',#17605,#17437,#11740,.T.);
#22831=EDGE_CURVE('',#17436,#17606,#11741,.T.);
#22832=EDGE_CURVE('',#17607,#17435,#11742,.T.);
#22833=EDGE_CURVE('',#17603,#17439,#11743,.T.);
#22834=EDGE_CURVE('',#17438,#17604,#11744,.T.);
#22835=EDGE_CURVE('',#17440,#17602,#11745,.T.);
#22836=EDGE_CURVE('',#17615,#17616,#8542,.T.);
#22837=EDGE_CURVE('',#17616,#17443,#11746,.T.);
#22838=EDGE_CURVE('',#17442,#17615,#11747,.T.);
#22839=EDGE_CURVE('',#17617,#17441,#11748,.T.);
#22840=EDGE_CURVE('',#17618,#17617,#10157,.F.);
#22841=EDGE_CURVE('',#17619,#17618,#8543,.T.);
#22842=EDGE_CURVE('',#17619,#17620,#11749,.T.);
#22843=EDGE_CURVE('',#17615,#17620,#11750,.T.);
#22844=EDGE_CURVE('',#17621,#17622,#8544,.T.);
#22845=EDGE_CURVE('',#17622,#17445,#11751,.T.);
#22846=EDGE_CURVE('',#17444,#17621,#11752,.T.);
#22847=EDGE_CURVE('',#17622,#17623,#11753,.T.);
#22848=EDGE_CURVE('',#17624,#17623,#11754,.T.);
#22849=EDGE_CURVE('',#17625,#17624,#8545,.T.);
#22850=EDGE_CURVE('',#17625,#17626,#10158,.T.);
#22851=EDGE_CURVE('',#17446,#17626,#11755,.T.);
#22852=EDGE_CURVE('',#17620,#17623,#11756,.T.);
#22853=EDGE_CURVE('',#17621,#17616,#11757,.T.);
#22854=EDGE_CURVE('',#17627,#17628,#8546,.T.);
#22855=EDGE_CURVE('',#17628,#17451,#11758,.T.);
#22856=EDGE_CURVE('',#17450,#17627,#11759,.T.);
#22857=EDGE_CURVE('',#17627,#17629,#11760,.T.);
#22858=EDGE_CURVE('',#17630,#17629,#8547,.T.);
#22859=EDGE_CURVE('',#17630,#17631,#11761,.T.);
#22860=EDGE_CURVE('',#17632,#17631,#8548,.T.);
#22861=EDGE_CURVE('',#17633,#17632,#10159,.T.);
#22862=EDGE_CURVE('',#17634,#17633,#8549,.T.);
#22863=EDGE_CURVE('',#17635,#17634,#10160,.T.);
#22864=EDGE_CURVE('',#17636,#17635,#8550,.T.);
#22865=EDGE_CURVE('',#17636,#17637,#11762,.T.);
#22866=EDGE_CURVE('',#17638,#17637,#8551,.T.);
#22867=EDGE_CURVE('',#17638,#17639,#11763,.T.);
#22868=EDGE_CURVE('',#17640,#17639,#8552,.T.);
#22869=EDGE_CURVE('',#17640,#17641,#11764,.T.);
#22870=EDGE_CURVE('',#17642,#17641,#8553,.T.);
#22871=EDGE_CURVE('',#17642,#17643,#11765,.T.);
#22872=EDGE_CURVE('',#17644,#17643,#8554,.T.);
#22873=EDGE_CURVE('',#17644,#17645,#11766,.T.);
#22874=EDGE_CURVE('',#17646,#17645,#8555,.T.);
#22875=EDGE_CURVE('',#17646,#17647,#11767,.T.);
#22876=EDGE_CURVE('',#17648,#17647,#8556,.T.);
#22877=EDGE_CURVE('',#17648,#17628,#11768,.T.);
#22878=EDGE_CURVE('',#17629,#17449,#11769,.T.);
#22879=EDGE_CURVE('',#17448,#17630,#11770,.T.);
#22880=EDGE_CURVE('',#17645,#17455,#11771,.T.);
#22881=EDGE_CURVE('',#17454,#17646,#11772,.T.);
#22882=EDGE_CURVE('',#17647,#17453,#11773,.T.);
#22883=EDGE_CURVE('',#17643,#17457,#11774,.T.);
#22884=EDGE_CURVE('',#17456,#17644,#11775,.T.);
#22885=EDGE_CURVE('',#17458,#17642,#11776,.T.);
#22886=EDGE_CURVE('',#17649,#17650,#8557,.T.);
#22887=EDGE_CURVE('',#17650,#17651,#10161,.T.);
#22888=EDGE_CURVE('',#17651,#17652,#8558,.T.);
#22889=EDGE_CURVE('',#17652,#17649,#10162,.T.);
#22890=EDGE_CURVE('',#17651,#17470,#8559,.T.);
#22891=EDGE_CURVE('',#17470,#17652,#8560,.T.);
#22892=EDGE_CURVE('',#17649,#17317,#8561,.T.);
#22893=EDGE_CURVE('',#17317,#17650,#8562,.T.);
#22894=EDGE_CURVE('',#17318,#17653,#8563,.T.);
#22895=EDGE_CURVE('',#17653,#17650,#8564,.T.);
#22896=EDGE_CURVE('',#17649,#17654,#10163,.T.);
#22897=EDGE_CURVE('',#17654,#17655,#10164,.T.);
#22898=EDGE_CURVE('',#17655,#17319,#10165,.T.);
#22899=EDGE_CURVE('',#17656,#17652,#10166,.T.);
#22900=EDGE_CURVE('',#17656,#17657,#8565,.T.);
#22901=EDGE_CURVE('',#17657,#17658,#10167,.T.);
#22902=EDGE_CURVE('',#17658,#17659,#8566,.T.);
#22903=EDGE_CURVE('',#17660,#17659,#10168,.T.);
#22904=EDGE_CURVE('',#17654,#17660,#10169,.T.);
#22905=EDGE_CURVE('',#17661,#17662,#8567,.T.);
#22906=EDGE_CURVE('',#17662,#17663,#10170,.T.);
#22907=EDGE_CURVE('',#17663,#17664,#8568,.T.);
#22908=EDGE_CURVE('',#17664,#17661,#10171,.T.);
#22909=EDGE_CURVE('',#17663,#17565,#8569,.T.);
#22910=EDGE_CURVE('',#17565,#17664,#8570,.T.);
#22911=EDGE_CURVE('',#17661,#17324,#8571,.T.);
#22912=EDGE_CURVE('',#17324,#17662,#8572,.T.);
#22913=EDGE_CURVE('',#17564,#17558,#10172,.T.);
#22914=EDGE_CURVE('',#17557,#17664,#10173,.T.);
#22915=EDGE_CURVE('',#17663,#17665,#8573,.T.);
#22916=EDGE_CURVE('',#17566,#17665,#8574,.T.);
#22917=EDGE_CURVE('',#17666,#17662,#8575,.T.);
#22918=EDGE_CURVE('',#17665,#17666,#10174,.T.);
#22919=EDGE_CURVE('',#17318,#17667,#8576,.T.);
#22920=EDGE_CURVE('',#17667,#17653,#8577,.T.);
#22921=EDGE_CURVE('',#17655,#17668,#8578,.T.);
#22922=EDGE_CURVE('',#17668,#17320,#10175,.T.);
#22923=EDGE_CURVE('',#17669,#17670,#10176,.T.);
#22924=EDGE_CURVE('',#17670,#17321,#8579,.T.);
#22925=EDGE_CURVE('',#17668,#17669,#10177,.T.);
#22926=EDGE_CURVE('',#17670,#17671,#8580,.T.);
#22927=EDGE_CURVE('',#17671,#17321,#8581,.T.);
#22928=EDGE_CURVE('',#17672,#17328,#8582,.T.);
#22929=EDGE_CURVE('',#17672,#17667,#10178,.T.);
#22930=EDGE_CURVE('',#17671,#17673,#8583,.T.);
#22931=EDGE_CURVE('',#17673,#17674,#8584,.T.);
#22932=EDGE_CURVE('',#17322,#17674,#8585,.T.);
#22933=EDGE_CURVE('',#17670,#17675,#10179,.T.);
#22934=EDGE_CURVE('',#17675,#17676,#8586,.F.);
#22935=EDGE_CURVE('',#17676,#17671,#10180,.T.);
#22936=EDGE_CURVE('',#17677,#17669,#10181,.T.);
#22937=EDGE_CURVE('',#17625,#17677,#10182,.T.);
#22938=EDGE_CURVE('',#17624,#17619,#10183,.T.);
#22939=EDGE_CURVE('',#17675,#17618,#10184,.T.);
#22940=EDGE_CURVE('',#17678,#17679,#8587,.T.);
#22941=EDGE_CURVE('',#17679,#17680,#10185,.T.);
#22942=EDGE_CURVE('',#17680,#17681,#8588,.T.);
#22943=EDGE_CURVE('',#17681,#17678,#10186,.T.);
#22944=EDGE_CURVE('',#17678,#17498,#8589,.T.);
#22945=EDGE_CURVE('',#17498,#17679,#8590,.T.);
#22946=EDGE_CURVE('',#17327,#17680,#8591,.T.);
#22947=EDGE_CURVE('',#17680,#17682,#8592,.T.);
#22948=EDGE_CURVE('',#17682,#17683,#8593,.T.);
#22949=EDGE_CURVE('',#17683,#17328,#8594,.T.);
#22950=EDGE_CURVE('',#17683,#17672,#8595,.T.);
#22951=EDGE_CURVE('',#17327,#17681,#8596,.T.);
#22952=EDGE_CURVE('',#17684,#17497,#8597,.T.);
#22953=EDGE_CURVE('',#17684,#17679,#8598,.T.);
#22954=EDGE_CURVE('',#17678,#17516,#10187,.T.);
#22955=EDGE_CURVE('',#17515,#17499,#10188,.T.);
#22956=EDGE_CURVE('',#17685,#17681,#10189,.T.);
#22957=EDGE_CURVE('',#17686,#17685,#10190,.T.);
#22958=EDGE_CURVE('',#17523,#17686,#10191,.T.);
#22959=EDGE_CURVE('',#17522,#17517,#10192,.T.);
#22960=EDGE_CURVE('',#17685,#17326,#8599,.T.);
#22961=EDGE_CURVE('',#17685,#17687,#8600,.T.);
#22962=EDGE_CURVE('',#17687,#17688,#10193,.T.);
#22963=EDGE_CURVE('',#17688,#17686,#8601,.T.);
#22964=EDGE_CURVE('',#17688,#17531,#8602,.T.);
#22965=EDGE_CURVE('',#17531,#17686,#8603,.T.);
#22966=EDGE_CURVE('',#17326,#17687,#8604,.T.);
#22967=EDGE_CURVE('',#17530,#17524,#10194,.T.);
#22968=EDGE_CURVE('',#17688,#17689,#8605,.T.);
#22969=EDGE_CURVE('',#17532,#17689,#10195,.T.);
#22970=EDGE_CURVE('',#17690,#17687,#8606,.T.);
#22971=EDGE_CURVE('',#17691,#17690,#10196,.T.);
#22972=EDGE_CURVE('',#17691,#17692,#10197,.T.);
#22973=EDGE_CURVE('',#17689,#17692,#10198,.T.);
#22974=EDGE_CURVE('',#17325,#17690,#10199,.T.);
#22975=EDGE_CURVE('',#17323,#17666,#8607,.T.);
#22976=EDGE_CURVE('',#17323,#17693,#8608,.T.);
#22977=EDGE_CURVE('',#17693,#17666,#8609,.T.);
#22978=EDGE_CURVE('',#17661,#17691,#10200,.T.);
#22979=EDGE_CURVE('',#17556,#17551,#10201,.T.);
#22980=EDGE_CURVE('',#17692,#17550,#10202,.T.);
#22981=EDGE_CURVE('',#17600,#17675,#8610,.F.);
#22982=EDGE_CURVE('',#17676,#17600,#8611,.F.);
#22983=EDGE_CURVE('',#17617,#17601,#10203,.T.);
#22984=EDGE_CURVE('',#17694,#17599,#8612,.T.);
#22985=EDGE_CURVE('',#17599,#17695,#8613,.T.);
#22986=EDGE_CURVE('',#17695,#17694,#8614,.T.);
#22987=EDGE_CURVE('',#17694,#17676,#8615,.T.);
#22988=EDGE_CURVE('',#17674,#17696,#8616,.T.);
#22989=EDGE_CURVE('',#17696,#17322,#8617,.T.);
#22990=EDGE_CURVE('',#17696,#17693,#10204,.T.);
#22991=EDGE_CURVE('',#17598,#17592,#10205,.T.);
#22992=EDGE_CURVE('',#17591,#17695,#10206,.T.);
#22993=EDGE_CURVE('',#17695,#17696,#10207,.T.);
#22994=EDGE_CURVE('',#17674,#17694,#10208,.T.);
#22995=EDGE_CURVE('',#17693,#17697,#10209,.T.);
#22996=EDGE_CURVE('',#17697,#17665,#8618,.T.);
#22997=EDGE_CURVE('',#17697,#17566,#8619,.T.);
#22998=EDGE_CURVE('',#17597,#17423,#11777,.T.);
#22999=EDGE_CURVE('',#17673,#17698,#8620,.T.);
#23000=EDGE_CURVE('',#17697,#17584,#10210,.T.);
#23001=EDGE_CURVE('',#17583,#17567,#10211,.T.);
#23002=EDGE_CURVE('',#17590,#17585,#10212,.T.);
#23003=EDGE_CURVE('',#17549,#17533,#10213,.T.);
#23004=EDGE_CURVE('',#17497,#17699,#8621,.T.);
#23005=EDGE_CURVE('',#17699,#17684,#8622,.T.);
#23006=EDGE_CURVE('',#17683,#17684,#10214,.T.);
#23007=EDGE_CURVE('',#17700,#17682,#8623,.T.);
#23008=EDGE_CURVE('',#17699,#17672,#10215,.T.);
#23009=EDGE_CURVE('',#17496,#17701,#10216,.T.);
#23010=EDGE_CURVE('',#17702,#17701,#10217,.T.);
#23011=EDGE_CURVE('',#17702,#17699,#10218,.T.);
#23012=EDGE_CURVE('',#17667,#17703,#10219,.T.);
#23013=EDGE_CURVE('',#17703,#17704,#8624,.T.);
#23014=EDGE_CURVE('',#17704,#17653,#10220,.T.);
#23015=EDGE_CURVE('',#17703,#17471,#8625,.T.);
#23016=EDGE_CURVE('',#17471,#17704,#8626,.T.);
#23017=EDGE_CURVE('',#17495,#17351,#11778,.T.);
#23018=EDGE_CURVE('',#17350,#17701,#11779,.T.);
#23019=EDGE_CURVE('',#17703,#17705,#10221,.T.);
#23020=EDGE_CURVE('',#17705,#17706,#10222,.F.);
#23021=EDGE_CURVE('',#17706,#17472,#10223,.T.);
#23022=EDGE_CURVE('',#17651,#17704,#8627,.T.);
#23023=EDGE_CURVE('',#17469,#17707,#10224,.T.);
#23024=EDGE_CURVE('',#17656,#17707,#10225,.T.);
#23025=EDGE_CURVE('',#17702,#17708,#8628,.T.);
#23026=EDGE_CURVE('',#17708,#17709,#10226,.T.);
#23027=EDGE_CURVE('',#17709,#17705,#8629,.T.);
#23028=EDGE_CURVE('',#17659,#17710,#10227,.F.);
#23029=EDGE_CURVE('',#17710,#17635,#10228,.T.);
#23030=EDGE_CURVE('',#17634,#17711,#10229,.T.);
#23031=EDGE_CURVE('',#17711,#17660,#10230,.T.);
#23032=EDGE_CURVE('',#17633,#17712,#10231,.T.);
#23033=EDGE_CURVE('',#17712,#17711,#8630,.T.);
#23034=EDGE_CURVE('',#17632,#17626,#10232,.T.);
#23035=EDGE_CURVE('',#17677,#17712,#10233,.T.);
#23036=EDGE_CURVE('',#17639,#17461,#11780,.T.);
#23037=EDGE_CURVE('',#17460,#17640,#11781,.T.);
#23038=EDGE_CURVE('',#17462,#17638,#11782,.T.);
#23039=EDGE_CURVE('',#17637,#17463,#11783,.T.);
#23040=EDGE_CURVE('',#17464,#17636,#11784,.T.);
#23041=EDGE_CURVE('',#17641,#17459,#11785,.T.);
#23042=EDGE_CURVE('',#17710,#17465,#11786,.T.);
#23043=EDGE_CURVE('',#17452,#17648,#11787,.T.);
#23044=EDGE_CURVE('',#17631,#17447,#11788,.T.);
#23045=EDGE_CURVE('',#17428,#17614,#11789,.T.);
#23046=EDGE_CURVE('',#17404,#17580,#11790,.T.);
#23047=EDGE_CURVE('',#17563,#17399,#11791,.T.);
#23048=EDGE_CURVE('',#17380,#17546,#11792,.T.);
#23049=EDGE_CURVE('',#17529,#17375,#11793,.T.);
#23050=EDGE_CURVE('',#17356,#17512,#11794,.T.);
#23051=EDGE_CURVE('',#17708,#17490,#11795,.T.);
#23052=EDGE_CURVE('',#17709,#17489,#11796,.T.);
#23053=EDGE_CURVE('',#17706,#17345,#11797,.T.);
#23054=EDGE_CURVE('',#17344,#17473,#11798,.T.);
#23055=EDGE_CURVE('',#17478,#17339,#11799,.T.);
#23056=EDGE_CURVE('',#17338,#17479,#11800,.T.);
#23057=EDGE_CURVE('',#17484,#17333,#11801,.T.);
#23058=EDGE_CURVE('',#17329,#17707,#11802,.T.);
#23059=EDGE_CURVE('',#17658,#17307,#11803,.T.);
#23060=EDGE_CURVE('',#17657,#17308,#11804,.T.);
#31813=ORIENTED_EDGE('',*,*,#22418,.T.);
#31814=ORIENTED_EDGE('',*,*,#22419,.T.);
#31815=ORIENTED_EDGE('',*,*,#22420,.T.);
#31816=ORIENTED_EDGE('',*,*,#22421,.T.);
#31817=ORIENTED_EDGE('',*,*,#22418,.F.);
#31818=ORIENTED_EDGE('',*,*,#22422,.T.);
#31819=ORIENTED_EDGE('',*,*,#22423,.F.);
#31820=ORIENTED_EDGE('',*,*,#22424,.T.);
#31821=ORIENTED_EDGE('',*,*,#22425,.T.);
#31822=ORIENTED_EDGE('',*,*,#22426,.F.);
#31823=ORIENTED_EDGE('',*,*,#22421,.F.);
#31824=ORIENTED_EDGE('',*,*,#22427,.T.);
#31825=ORIENTED_EDGE('',*,*,#22428,.F.);
#31826=ORIENTED_EDGE('',*,*,#22422,.F.);
#31827=ORIENTED_EDGE('',*,*,#22423,.T.);
#31828=ORIENTED_EDGE('',*,*,#22428,.T.);
#31829=ORIENTED_EDGE('',*,*,#22429,.T.);
#31830=ORIENTED_EDGE('',*,*,#22430,.T.);
#31831=ORIENTED_EDGE('',*,*,#22431,.T.);
#31832=ORIENTED_EDGE('',*,*,#22432,.T.);
#31833=ORIENTED_EDGE('',*,*,#22433,.T.);
#31834=ORIENTED_EDGE('',*,*,#22434,.T.);
#31835=ORIENTED_EDGE('',*,*,#22434,.F.);
#31836=ORIENTED_EDGE('',*,*,#22435,.T.);
#31837=ORIENTED_EDGE('',*,*,#22436,.F.);
#31838=ORIENTED_EDGE('',*,*,#22437,.F.);
#31839=ORIENTED_EDGE('',*,*,#22438,.F.);
#31840=ORIENTED_EDGE('',*,*,#22439,.F.);
#31841=ORIENTED_EDGE('',*,*,#22440,.F.);
#31842=ORIENTED_EDGE('',*,*,#22441,.F.);
#31843=ORIENTED_EDGE('',*,*,#22442,.F.);
#31844=ORIENTED_EDGE('',*,*,#22443,.F.);
#31845=ORIENTED_EDGE('',*,*,#22444,.F.);
#31846=ORIENTED_EDGE('',*,*,#22445,.F.);
#31847=ORIENTED_EDGE('',*,*,#22446,.F.);
#31848=ORIENTED_EDGE('',*,*,#22447,.F.);
#31849=ORIENTED_EDGE('',*,*,#22448,.F.);
#31850=ORIENTED_EDGE('',*,*,#22449,.F.);
#31851=ORIENTED_EDGE('',*,*,#22420,.F.);
#31852=ORIENTED_EDGE('',*,*,#22450,.F.);
#31853=ORIENTED_EDGE('',*,*,#22451,.T.);
#31854=ORIENTED_EDGE('',*,*,#22435,.F.);
#31855=ORIENTED_EDGE('',*,*,#22433,.F.);
#31856=ORIENTED_EDGE('',*,*,#22452,.F.);
#31857=ORIENTED_EDGE('',*,*,#22453,.F.);
#31858=ORIENTED_EDGE('',*,*,#22454,.F.);
#31859=ORIENTED_EDGE('',*,*,#22455,.T.);
#31860=ORIENTED_EDGE('',*,*,#22456,.F.);
#31861=ORIENTED_EDGE('',*,*,#22457,.F.);
#31862=ORIENTED_EDGE('',*,*,#22458,.F.);
#31863=ORIENTED_EDGE('',*,*,#22459,.F.);
#31864=ORIENTED_EDGE('',*,*,#22460,.F.);
#31865=ORIENTED_EDGE('',*,*,#22461,.T.);
#31866=ORIENTED_EDGE('',*,*,#22462,.F.);
#31867=ORIENTED_EDGE('',*,*,#22463,.F.);
#31868=ORIENTED_EDGE('',*,*,#22464,.F.);
#31869=ORIENTED_EDGE('',*,*,#22465,.F.);
#31870=ORIENTED_EDGE('',*,*,#22466,.F.);
#31871=ORIENTED_EDGE('',*,*,#22467,.T.);
#31872=ORIENTED_EDGE('',*,*,#22468,.F.);
#31873=ORIENTED_EDGE('',*,*,#22469,.F.);
#31874=ORIENTED_EDGE('',*,*,#22470,.F.);
#31875=ORIENTED_EDGE('',*,*,#22471,.F.);
#31876=ORIENTED_EDGE('',*,*,#22472,.F.);
#31877=ORIENTED_EDGE('',*,*,#22473,.T.);
#31878=ORIENTED_EDGE('',*,*,#22474,.F.);
#31879=ORIENTED_EDGE('',*,*,#22475,.F.);
#31880=ORIENTED_EDGE('',*,*,#22476,.F.);
#31881=ORIENTED_EDGE('',*,*,#22477,.F.);
#31882=ORIENTED_EDGE('',*,*,#22478,.F.);
#31883=ORIENTED_EDGE('',*,*,#22479,.T.);
#31884=ORIENTED_EDGE('',*,*,#22480,.F.);
#31885=ORIENTED_EDGE('',*,*,#22481,.F.);
#31886=ORIENTED_EDGE('',*,*,#22482,.F.);
#31887=ORIENTED_EDGE('',*,*,#22483,.F.);
#31888=ORIENTED_EDGE('',*,*,#22484,.F.);
#31889=ORIENTED_EDGE('',*,*,#22485,.T.);
#31890=ORIENTED_EDGE('',*,*,#22486,.F.);
#31891=ORIENTED_EDGE('',*,*,#22487,.F.);
#31892=ORIENTED_EDGE('',*,*,#22488,.F.);
#31893=ORIENTED_EDGE('',*,*,#22489,.F.);
#31894=ORIENTED_EDGE('',*,*,#22490,.F.);
#31895=ORIENTED_EDGE('',*,*,#22491,.T.);
#31896=ORIENTED_EDGE('',*,*,#22492,.F.);
#31897=ORIENTED_EDGE('',*,*,#22493,.F.);
#31898=ORIENTED_EDGE('',*,*,#22494,.F.);
#31899=ORIENTED_EDGE('',*,*,#22495,.F.);
#31900=ORIENTED_EDGE('',*,*,#22496,.F.);
#31901=ORIENTED_EDGE('',*,*,#22497,.T.);
#31902=ORIENTED_EDGE('',*,*,#22498,.F.);
#31903=ORIENTED_EDGE('',*,*,#22499,.F.);
#31904=ORIENTED_EDGE('',*,*,#22500,.F.);
#31905=ORIENTED_EDGE('',*,*,#22501,.F.);
#31906=ORIENTED_EDGE('',*,*,#22502,.F.);
#31907=ORIENTED_EDGE('',*,*,#22503,.T.);
#31908=ORIENTED_EDGE('',*,*,#22504,.F.);
#31909=ORIENTED_EDGE('',*,*,#22505,.F.);
#31910=ORIENTED_EDGE('',*,*,#22506,.F.);
#31911=ORIENTED_EDGE('',*,*,#22507,.F.);
#31912=ORIENTED_EDGE('',*,*,#22508,.F.);
#31913=ORIENTED_EDGE('',*,*,#22509,.T.);
#31914=ORIENTED_EDGE('',*,*,#22510,.F.);
#31915=ORIENTED_EDGE('',*,*,#22511,.F.);
#31916=ORIENTED_EDGE('',*,*,#22512,.F.);
#31917=ORIENTED_EDGE('',*,*,#22513,.F.);
#31918=ORIENTED_EDGE('',*,*,#22514,.F.);
#31919=ORIENTED_EDGE('',*,*,#22515,.T.);
#31920=ORIENTED_EDGE('',*,*,#22516,.F.);
#31921=ORIENTED_EDGE('',*,*,#22517,.F.);
#31922=ORIENTED_EDGE('',*,*,#22518,.F.);
#31923=ORIENTED_EDGE('',*,*,#22519,.F.);
#31924=ORIENTED_EDGE('',*,*,#22520,.F.);
#31925=ORIENTED_EDGE('',*,*,#22521,.T.);
#31926=ORIENTED_EDGE('',*,*,#22522,.F.);
#31927=ORIENTED_EDGE('',*,*,#22523,.F.);
#31928=ORIENTED_EDGE('',*,*,#22524,.F.);
#31929=ORIENTED_EDGE('',*,*,#22525,.F.);
#31930=ORIENTED_EDGE('',*,*,#22526,.F.);
#31931=ORIENTED_EDGE('',*,*,#22527,.T.);
#31932=ORIENTED_EDGE('',*,*,#22528,.F.);
#31933=ORIENTED_EDGE('',*,*,#22529,.F.);
#31934=ORIENTED_EDGE('',*,*,#22530,.F.);
#31935=ORIENTED_EDGE('',*,*,#22531,.F.);
#31936=ORIENTED_EDGE('',*,*,#22532,.F.);
#31937=ORIENTED_EDGE('',*,*,#22533,.T.);
#31938=ORIENTED_EDGE('',*,*,#22534,.F.);
#31939=ORIENTED_EDGE('',*,*,#22535,.F.);
#31940=ORIENTED_EDGE('',*,*,#22536,.F.);
#31941=ORIENTED_EDGE('',*,*,#22537,.F.);
#31942=ORIENTED_EDGE('',*,*,#22538,.F.);
#31943=ORIENTED_EDGE('',*,*,#22539,.T.);
#31944=ORIENTED_EDGE('',*,*,#22540,.F.);
#31945=ORIENTED_EDGE('',*,*,#22541,.F.);
#31946=ORIENTED_EDGE('',*,*,#22542,.F.);
#31947=ORIENTED_EDGE('',*,*,#22543,.F.);
#31948=ORIENTED_EDGE('',*,*,#22544,.F.);
#31949=ORIENTED_EDGE('',*,*,#22545,.T.);
#31950=ORIENTED_EDGE('',*,*,#22546,.F.);
#31951=ORIENTED_EDGE('',*,*,#22547,.F.);
#31952=ORIENTED_EDGE('',*,*,#22548,.F.);
#31953=ORIENTED_EDGE('',*,*,#22549,.F.);
#31954=ORIENTED_EDGE('',*,*,#22550,.F.);
#31955=ORIENTED_EDGE('',*,*,#22551,.T.);
#31956=ORIENTED_EDGE('',*,*,#22552,.F.);
#31957=ORIENTED_EDGE('',*,*,#22553,.F.);
#31958=ORIENTED_EDGE('',*,*,#22554,.F.);
#31959=ORIENTED_EDGE('',*,*,#22555,.F.);
#31960=ORIENTED_EDGE('',*,*,#22556,.F.);
#31961=ORIENTED_EDGE('',*,*,#22557,.T.);
#31962=ORIENTED_EDGE('',*,*,#22558,.F.);
#31963=ORIENTED_EDGE('',*,*,#22559,.F.);
#31964=ORIENTED_EDGE('',*,*,#22560,.F.);
#31965=ORIENTED_EDGE('',*,*,#22561,.F.);
#31966=ORIENTED_EDGE('',*,*,#22562,.F.);
#31967=ORIENTED_EDGE('',*,*,#22563,.T.);
#31968=ORIENTED_EDGE('',*,*,#22564,.F.);
#31969=ORIENTED_EDGE('',*,*,#22565,.F.);
#31970=ORIENTED_EDGE('',*,*,#22566,.F.);
#31971=ORIENTED_EDGE('',*,*,#22567,.F.);
#31972=ORIENTED_EDGE('',*,*,#22568,.F.);
#31973=ORIENTED_EDGE('',*,*,#22569,.T.);
#31974=ORIENTED_EDGE('',*,*,#22570,.F.);
#31975=ORIENTED_EDGE('',*,*,#22571,.F.);
#31976=ORIENTED_EDGE('',*,*,#22572,.F.);
#31977=ORIENTED_EDGE('',*,*,#22573,.F.);
#31978=ORIENTED_EDGE('',*,*,#22574,.F.);
#31979=ORIENTED_EDGE('',*,*,#22575,.T.);
#31980=ORIENTED_EDGE('',*,*,#22576,.F.);
#31981=ORIENTED_EDGE('',*,*,#22577,.F.);
#31982=ORIENTED_EDGE('',*,*,#22578,.F.);
#31983=ORIENTED_EDGE('',*,*,#22579,.F.);
#31984=ORIENTED_EDGE('',*,*,#22580,.F.);
#31985=ORIENTED_EDGE('',*,*,#22581,.T.);
#31986=ORIENTED_EDGE('',*,*,#22582,.F.);
#31987=ORIENTED_EDGE('',*,*,#22583,.F.);
#31988=ORIENTED_EDGE('',*,*,#22584,.F.);
#31989=ORIENTED_EDGE('',*,*,#22585,.F.);
#31990=ORIENTED_EDGE('',*,*,#22586,.F.);
#31991=ORIENTED_EDGE('',*,*,#22587,.T.);
#31992=ORIENTED_EDGE('',*,*,#22588,.F.);
#31993=ORIENTED_EDGE('',*,*,#22429,.F.);
#31994=ORIENTED_EDGE('',*,*,#22427,.F.);
#31995=ORIENTED_EDGE('',*,*,#22589,.T.);
#31996=ORIENTED_EDGE('',*,*,#22590,.T.);
#31997=ORIENTED_EDGE('',*,*,#22453,.T.);
#31998=ORIENTED_EDGE('',*,*,#22591,.T.);
#31999=ORIENTED_EDGE('',*,*,#22590,.F.);
#32000=ORIENTED_EDGE('',*,*,#22592,.F.);
#32001=ORIENTED_EDGE('',*,*,#22593,.F.);
#32002=ORIENTED_EDGE('',*,*,#22454,.T.);
#32003=ORIENTED_EDGE('',*,*,#22431,.F.);
#32004=ORIENTED_EDGE('',*,*,#22437,.T.);
#32005=ORIENTED_EDGE('',*,*,#22594,.F.);
#32006=ORIENTED_EDGE('',*,*,#22595,.F.);
#32007=ORIENTED_EDGE('',*,*,#22596,.F.);
#32008=ORIENTED_EDGE('',*,*,#22597,.F.);
#32009=ORIENTED_EDGE('',*,*,#22598,.F.);
#32010=ORIENTED_EDGE('',*,*,#22599,.T.);
#32011=ORIENTED_EDGE('',*,*,#22600,.F.);
#32012=ORIENTED_EDGE('',*,*,#22601,.T.);
#32013=ORIENTED_EDGE('',*,*,#22602,.F.);
#32014=ORIENTED_EDGE('',*,*,#22603,.T.);
#32015=ORIENTED_EDGE('',*,*,#22604,.F.);
#32016=ORIENTED_EDGE('',*,*,#22605,.T.);
#32017=ORIENTED_EDGE('',*,*,#22606,.F.);
#32018=ORIENTED_EDGE('',*,*,#22607,.T.);
#32019=ORIENTED_EDGE('',*,*,#22608,.F.);
#32020=ORIENTED_EDGE('',*,*,#22609,.T.);
#32021=ORIENTED_EDGE('',*,*,#22610,.F.);
#32022=ORIENTED_EDGE('',*,*,#22592,.T.);
#32023=ORIENTED_EDGE('',*,*,#22589,.F.);
#32024=ORIENTED_EDGE('',*,*,#22611,.T.);
#32025=ORIENTED_EDGE('',*,*,#22608,.T.);
#32026=ORIENTED_EDGE('',*,*,#22612,.T.);
#32027=ORIENTED_EDGE('',*,*,#22457,.T.);
#32028=ORIENTED_EDGE('',*,*,#22613,.T.);
#32029=ORIENTED_EDGE('',*,*,#22612,.F.);
#32030=ORIENTED_EDGE('',*,*,#22607,.F.);
#32031=ORIENTED_EDGE('',*,*,#22614,.F.);
#32032=ORIENTED_EDGE('',*,*,#22458,.T.);
#32033=ORIENTED_EDGE('',*,*,#22606,.T.);
#32034=ORIENTED_EDGE('',*,*,#22615,.T.);
#32035=ORIENTED_EDGE('',*,*,#22459,.T.);
#32036=ORIENTED_EDGE('',*,*,#22614,.T.);
#32037=ORIENTED_EDGE('',*,*,#22600,.T.);
#32038=ORIENTED_EDGE('',*,*,#22616,.T.);
#32039=ORIENTED_EDGE('',*,*,#22465,.T.);
#32040=ORIENTED_EDGE('',*,*,#22617,.T.);
#32041=ORIENTED_EDGE('',*,*,#22617,.F.);
#32042=ORIENTED_EDGE('',*,*,#22464,.T.);
#32043=ORIENTED_EDGE('',*,*,#22618,.F.);
#32044=ORIENTED_EDGE('',*,*,#22601,.F.);
#32045=ORIENTED_EDGE('',*,*,#22602,.T.);
#32046=ORIENTED_EDGE('',*,*,#22618,.T.);
#32047=ORIENTED_EDGE('',*,*,#22463,.T.);
#32048=ORIENTED_EDGE('',*,*,#22619,.T.);
#32049=ORIENTED_EDGE('',*,*,#22620,.T.);
#32050=ORIENTED_EDGE('',*,*,#22621,.T.);
#32051=ORIENTED_EDGE('',*,*,#22471,.T.);
#32052=ORIENTED_EDGE('',*,*,#22622,.T.);
#32053=ORIENTED_EDGE('',*,*,#22620,.F.);
#32054=ORIENTED_EDGE('',*,*,#22623,.T.);
#32055=ORIENTED_EDGE('',*,*,#22624,.F.);
#32056=ORIENTED_EDGE('',*,*,#22625,.T.);
#32057=ORIENTED_EDGE('',*,*,#22626,.T.);
#32058=ORIENTED_EDGE('',*,*,#22627,.F.);
#32059=ORIENTED_EDGE('',*,*,#22622,.F.);
#32060=ORIENTED_EDGE('',*,*,#22470,.T.);
#32061=ORIENTED_EDGE('',*,*,#22628,.F.);
#32062=ORIENTED_EDGE('',*,*,#22623,.F.);
#32063=ORIENTED_EDGE('',*,*,#22624,.T.);
#32064=ORIENTED_EDGE('',*,*,#22628,.T.);
#32065=ORIENTED_EDGE('',*,*,#22469,.T.);
#32066=ORIENTED_EDGE('',*,*,#22629,.T.);
#32067=ORIENTED_EDGE('',*,*,#22630,.T.);
#32068=ORIENTED_EDGE('',*,*,#22631,.T.);
#32069=ORIENTED_EDGE('',*,*,#22477,.T.);
#32070=ORIENTED_EDGE('',*,*,#22632,.T.);
#32071=ORIENTED_EDGE('',*,*,#22630,.F.);
#32072=ORIENTED_EDGE('',*,*,#22633,.T.);
#32073=ORIENTED_EDGE('',*,*,#22634,.F.);
#32074=ORIENTED_EDGE('',*,*,#22635,.T.);
#32075=ORIENTED_EDGE('',*,*,#22636,.F.);
#32076=ORIENTED_EDGE('',*,*,#22637,.F.);
#32077=ORIENTED_EDGE('',*,*,#22638,.F.);
#32078=ORIENTED_EDGE('',*,*,#22639,.F.);
#32079=ORIENTED_EDGE('',*,*,#22640,.F.);
#32080=ORIENTED_EDGE('',*,*,#22641,.T.);
#32081=ORIENTED_EDGE('',*,*,#22642,.F.);
#32082=ORIENTED_EDGE('',*,*,#22643,.T.);
#32083=ORIENTED_EDGE('',*,*,#22644,.F.);
#32084=ORIENTED_EDGE('',*,*,#22645,.T.);
#32085=ORIENTED_EDGE('',*,*,#22646,.F.);
#32086=ORIENTED_EDGE('',*,*,#22647,.T.);
#32087=ORIENTED_EDGE('',*,*,#22648,.F.);
#32088=ORIENTED_EDGE('',*,*,#22649,.T.);
#32089=ORIENTED_EDGE('',*,*,#22650,.F.);
#32090=ORIENTED_EDGE('',*,*,#22651,.T.);
#32091=ORIENTED_EDGE('',*,*,#22652,.F.);
#32092=ORIENTED_EDGE('',*,*,#22653,.T.);
#32093=ORIENTED_EDGE('',*,*,#22632,.F.);
#32094=ORIENTED_EDGE('',*,*,#22476,.T.);
#32095=ORIENTED_EDGE('',*,*,#22654,.F.);
#32096=ORIENTED_EDGE('',*,*,#22633,.F.);
#32097=ORIENTED_EDGE('',*,*,#22634,.T.);
#32098=ORIENTED_EDGE('',*,*,#22654,.T.);
#32099=ORIENTED_EDGE('',*,*,#22475,.T.);
#32100=ORIENTED_EDGE('',*,*,#22655,.T.);
#32101=ORIENTED_EDGE('',*,*,#22650,.T.);
#32102=ORIENTED_EDGE('',*,*,#22656,.T.);
#32103=ORIENTED_EDGE('',*,*,#22481,.T.);
#32104=ORIENTED_EDGE('',*,*,#22657,.T.);
#32105=ORIENTED_EDGE('',*,*,#22657,.F.);
#32106=ORIENTED_EDGE('',*,*,#22480,.T.);
#32107=ORIENTED_EDGE('',*,*,#22658,.F.);
#32108=ORIENTED_EDGE('',*,*,#22651,.F.);
#32109=ORIENTED_EDGE('',*,*,#22648,.T.);
#32110=ORIENTED_EDGE('',*,*,#22659,.T.);
#32111=ORIENTED_EDGE('',*,*,#22483,.T.);
#32112=ORIENTED_EDGE('',*,*,#22660,.T.);
#32113=ORIENTED_EDGE('',*,*,#22659,.F.);
#32114=ORIENTED_EDGE('',*,*,#22647,.F.);
#32115=ORIENTED_EDGE('',*,*,#22661,.F.);
#32116=ORIENTED_EDGE('',*,*,#22484,.T.);
#32117=ORIENTED_EDGE('',*,*,#22644,.T.);
#32118=ORIENTED_EDGE('',*,*,#22662,.T.);
#32119=ORIENTED_EDGE('',*,*,#22487,.T.);
#32120=ORIENTED_EDGE('',*,*,#22663,.T.);
#32121=ORIENTED_EDGE('',*,*,#22663,.F.);
#32122=ORIENTED_EDGE('',*,*,#22486,.T.);
#32123=ORIENTED_EDGE('',*,*,#22664,.F.);
#32124=ORIENTED_EDGE('',*,*,#22645,.F.);
#32125=ORIENTED_EDGE('',*,*,#22642,.T.);
#32126=ORIENTED_EDGE('',*,*,#22665,.T.);
#32127=ORIENTED_EDGE('',*,*,#22489,.T.);
#32128=ORIENTED_EDGE('',*,*,#22666,.T.);
#32129=ORIENTED_EDGE('',*,*,#22665,.F.);
#32130=ORIENTED_EDGE('',*,*,#22641,.F.);
#32131=ORIENTED_EDGE('',*,*,#22667,.F.);
#32132=ORIENTED_EDGE('',*,*,#22490,.T.);
#32133=ORIENTED_EDGE('',*,*,#22668,.T.);
#32134=ORIENTED_EDGE('',*,*,#22669,.T.);
#32135=ORIENTED_EDGE('',*,*,#22493,.T.);
#32136=ORIENTED_EDGE('',*,*,#22670,.T.);
#32137=ORIENTED_EDGE('',*,*,#22670,.F.);
#32138=ORIENTED_EDGE('',*,*,#22492,.T.);
#32139=ORIENTED_EDGE('',*,*,#22671,.F.);
#32140=ORIENTED_EDGE('',*,*,#22672,.F.);
#32141=ORIENTED_EDGE('',*,*,#22673,.F.);
#32142=ORIENTED_EDGE('',*,*,#22674,.T.);
#32143=ORIENTED_EDGE('',*,*,#22675,.F.);
#32144=ORIENTED_EDGE('',*,*,#22676,.T.);
#32145=ORIENTED_EDGE('',*,*,#22677,.T.);
#32146=ORIENTED_EDGE('',*,*,#22495,.T.);
#32147=ORIENTED_EDGE('',*,*,#22678,.T.);
#32148=ORIENTED_EDGE('',*,*,#22677,.F.);
#32149=ORIENTED_EDGE('',*,*,#22679,.T.);
#32150=ORIENTED_EDGE('',*,*,#22680,.F.);
#32151=ORIENTED_EDGE('',*,*,#22681,.F.);
#32152=ORIENTED_EDGE('',*,*,#22682,.T.);
#32153=ORIENTED_EDGE('',*,*,#22683,.F.);
#32154=ORIENTED_EDGE('',*,*,#22496,.T.);
#32155=ORIENTED_EDGE('',*,*,#22668,.F.);
#32156=ORIENTED_EDGE('',*,*,#22675,.T.);
#32157=ORIENTED_EDGE('',*,*,#22684,.T.);
#32158=ORIENTED_EDGE('',*,*,#22679,.F.);
#32159=ORIENTED_EDGE('',*,*,#22676,.F.);
#32160=ORIENTED_EDGE('',*,*,#22685,.T.);
#32161=ORIENTED_EDGE('',*,*,#22686,.T.);
#32162=ORIENTED_EDGE('',*,*,#22687,.T.);
#32163=ORIENTED_EDGE('',*,*,#22501,.T.);
#32164=ORIENTED_EDGE('',*,*,#22688,.T.);
#32165=ORIENTED_EDGE('',*,*,#22686,.F.);
#32166=ORIENTED_EDGE('',*,*,#22689,.T.);
#32167=ORIENTED_EDGE('',*,*,#22690,.F.);
#32168=ORIENTED_EDGE('',*,*,#22691,.T.);
#32169=ORIENTED_EDGE('',*,*,#22692,.F.);
#32170=ORIENTED_EDGE('',*,*,#22693,.F.);
#32171=ORIENTED_EDGE('',*,*,#22694,.F.);
#32172=ORIENTED_EDGE('',*,*,#22695,.F.);
#32173=ORIENTED_EDGE('',*,*,#22696,.F.);
#32174=ORIENTED_EDGE('',*,*,#22697,.T.);
#32175=ORIENTED_EDGE('',*,*,#22698,.F.);
#32176=ORIENTED_EDGE('',*,*,#22699,.T.);
#32177=ORIENTED_EDGE('',*,*,#22700,.F.);
#32178=ORIENTED_EDGE('',*,*,#22701,.T.);
#32179=ORIENTED_EDGE('',*,*,#22702,.F.);
#32180=ORIENTED_EDGE('',*,*,#22703,.T.);
#32181=ORIENTED_EDGE('',*,*,#22704,.F.);
#32182=ORIENTED_EDGE('',*,*,#22705,.T.);
#32183=ORIENTED_EDGE('',*,*,#22706,.F.);
#32184=ORIENTED_EDGE('',*,*,#22707,.T.);
#32185=ORIENTED_EDGE('',*,*,#22708,.F.);
#32186=ORIENTED_EDGE('',*,*,#22709,.T.);
#32187=ORIENTED_EDGE('',*,*,#22688,.F.);
#32188=ORIENTED_EDGE('',*,*,#22500,.T.);
#32189=ORIENTED_EDGE('',*,*,#22710,.F.);
#32190=ORIENTED_EDGE('',*,*,#22689,.F.);
#32191=ORIENTED_EDGE('',*,*,#22690,.T.);
#32192=ORIENTED_EDGE('',*,*,#22710,.T.);
#32193=ORIENTED_EDGE('',*,*,#22499,.T.);
#32194=ORIENTED_EDGE('',*,*,#22711,.T.);
#32195=ORIENTED_EDGE('',*,*,#22706,.T.);
#32196=ORIENTED_EDGE('',*,*,#22712,.T.);
#32197=ORIENTED_EDGE('',*,*,#22505,.T.);
#32198=ORIENTED_EDGE('',*,*,#22713,.T.);
#32199=ORIENTED_EDGE('',*,*,#22713,.F.);
#32200=ORIENTED_EDGE('',*,*,#22504,.T.);
#32201=ORIENTED_EDGE('',*,*,#22714,.F.);
#32202=ORIENTED_EDGE('',*,*,#22707,.F.);
#32203=ORIENTED_EDGE('',*,*,#22704,.T.);
#32204=ORIENTED_EDGE('',*,*,#22715,.T.);
#32205=ORIENTED_EDGE('',*,*,#22507,.T.);
#32206=ORIENTED_EDGE('',*,*,#22716,.T.);
#32207=ORIENTED_EDGE('',*,*,#22715,.F.);
#32208=ORIENTED_EDGE('',*,*,#22703,.F.);
#32209=ORIENTED_EDGE('',*,*,#22717,.F.);
#32210=ORIENTED_EDGE('',*,*,#22508,.T.);
#32211=ORIENTED_EDGE('',*,*,#22700,.T.);
#32212=ORIENTED_EDGE('',*,*,#22718,.T.);
#32213=ORIENTED_EDGE('',*,*,#22511,.T.);
#32214=ORIENTED_EDGE('',*,*,#22719,.T.);
#32215=ORIENTED_EDGE('',*,*,#22719,.F.);
#32216=ORIENTED_EDGE('',*,*,#22510,.T.);
#32217=ORIENTED_EDGE('',*,*,#22720,.F.);
#32218=ORIENTED_EDGE('',*,*,#22701,.F.);
#32219=ORIENTED_EDGE('',*,*,#22698,.T.);
#32220=ORIENTED_EDGE('',*,*,#22721,.T.);
#32221=ORIENTED_EDGE('',*,*,#22513,.T.);
#32222=ORIENTED_EDGE('',*,*,#22722,.T.);
#32223=ORIENTED_EDGE('',*,*,#22721,.F.);
#32224=ORIENTED_EDGE('',*,*,#22697,.F.);
#32225=ORIENTED_EDGE('',*,*,#22723,.F.);
#32226=ORIENTED_EDGE('',*,*,#22514,.T.);
#32227=ORIENTED_EDGE('',*,*,#22724,.T.);
#32228=ORIENTED_EDGE('',*,*,#22725,.T.);
#32229=ORIENTED_EDGE('',*,*,#22517,.T.);
#32230=ORIENTED_EDGE('',*,*,#22726,.T.);
#32231=ORIENTED_EDGE('',*,*,#22726,.F.);
#32232=ORIENTED_EDGE('',*,*,#22516,.T.);
#32233=ORIENTED_EDGE('',*,*,#22727,.F.);
#32234=ORIENTED_EDGE('',*,*,#22728,.F.);
#32235=ORIENTED_EDGE('',*,*,#22729,.F.);
#32236=ORIENTED_EDGE('',*,*,#22730,.T.);
#32237=ORIENTED_EDGE('',*,*,#22731,.F.);
#32238=ORIENTED_EDGE('',*,*,#22732,.T.);
#32239=ORIENTED_EDGE('',*,*,#22733,.T.);
#32240=ORIENTED_EDGE('',*,*,#22519,.T.);
#32241=ORIENTED_EDGE('',*,*,#22734,.T.);
#32242=ORIENTED_EDGE('',*,*,#22733,.F.);
#32243=ORIENTED_EDGE('',*,*,#22735,.T.);
#32244=ORIENTED_EDGE('',*,*,#22736,.F.);
#32245=ORIENTED_EDGE('',*,*,#22737,.F.);
#32246=ORIENTED_EDGE('',*,*,#22738,.T.);
#32247=ORIENTED_EDGE('',*,*,#22739,.F.);
#32248=ORIENTED_EDGE('',*,*,#22520,.T.);
#32249=ORIENTED_EDGE('',*,*,#22724,.F.);
#32250=ORIENTED_EDGE('',*,*,#22731,.T.);
#32251=ORIENTED_EDGE('',*,*,#22740,.T.);
#32252=ORIENTED_EDGE('',*,*,#22735,.F.);
#32253=ORIENTED_EDGE('',*,*,#22732,.F.);
#32254=ORIENTED_EDGE('',*,*,#22741,.T.);
#32255=ORIENTED_EDGE('',*,*,#22742,.T.);
#32256=ORIENTED_EDGE('',*,*,#22743,.T.);
#32257=ORIENTED_EDGE('',*,*,#22525,.T.);
#32258=ORIENTED_EDGE('',*,*,#22744,.T.);
#32259=ORIENTED_EDGE('',*,*,#22742,.F.);
#32260=ORIENTED_EDGE('',*,*,#22745,.T.);
#32261=ORIENTED_EDGE('',*,*,#22746,.F.);
#32262=ORIENTED_EDGE('',*,*,#22747,.T.);
#32263=ORIENTED_EDGE('',*,*,#22748,.F.);
#32264=ORIENTED_EDGE('',*,*,#22749,.F.);
#32265=ORIENTED_EDGE('',*,*,#22750,.F.);
#32266=ORIENTED_EDGE('',*,*,#22751,.F.);
#32267=ORIENTED_EDGE('',*,*,#22752,.F.);
#32268=ORIENTED_EDGE('',*,*,#22753,.T.);
#32269=ORIENTED_EDGE('',*,*,#22754,.F.);
#32270=ORIENTED_EDGE('',*,*,#22755,.T.);
#32271=ORIENTED_EDGE('',*,*,#22756,.F.);
#32272=ORIENTED_EDGE('',*,*,#22757,.T.);
#32273=ORIENTED_EDGE('',*,*,#22758,.F.);
#32274=ORIENTED_EDGE('',*,*,#22759,.T.);
#32275=ORIENTED_EDGE('',*,*,#22760,.F.);
#32276=ORIENTED_EDGE('',*,*,#22761,.T.);
#32277=ORIENTED_EDGE('',*,*,#22762,.F.);
#32278=ORIENTED_EDGE('',*,*,#22763,.T.);
#32279=ORIENTED_EDGE('',*,*,#22764,.F.);
#32280=ORIENTED_EDGE('',*,*,#22765,.T.);
#32281=ORIENTED_EDGE('',*,*,#22744,.F.);
#32282=ORIENTED_EDGE('',*,*,#22524,.T.);
#32283=ORIENTED_EDGE('',*,*,#22766,.F.);
#32284=ORIENTED_EDGE('',*,*,#22745,.F.);
#32285=ORIENTED_EDGE('',*,*,#22746,.T.);
#32286=ORIENTED_EDGE('',*,*,#22766,.T.);
#32287=ORIENTED_EDGE('',*,*,#22523,.T.);
#32288=ORIENTED_EDGE('',*,*,#22767,.T.);
#32289=ORIENTED_EDGE('',*,*,#22762,.T.);
#32290=ORIENTED_EDGE('',*,*,#22768,.T.);
#32291=ORIENTED_EDGE('',*,*,#22529,.T.);
#32292=ORIENTED_EDGE('',*,*,#22769,.T.);
#32293=ORIENTED_EDGE('',*,*,#22769,.F.);
#32294=ORIENTED_EDGE('',*,*,#22528,.T.);
#32295=ORIENTED_EDGE('',*,*,#22770,.F.);
#32296=ORIENTED_EDGE('',*,*,#22763,.F.);
#32297=ORIENTED_EDGE('',*,*,#22760,.T.);
#32298=ORIENTED_EDGE('',*,*,#22771,.T.);
#32299=ORIENTED_EDGE('',*,*,#22531,.T.);
#32300=ORIENTED_EDGE('',*,*,#22772,.T.);
#32301=ORIENTED_EDGE('',*,*,#22771,.F.);
#32302=ORIENTED_EDGE('',*,*,#22759,.F.);
#32303=ORIENTED_EDGE('',*,*,#22773,.F.);
#32304=ORIENTED_EDGE('',*,*,#22532,.T.);
#32305=ORIENTED_EDGE('',*,*,#22756,.T.);
#32306=ORIENTED_EDGE('',*,*,#22774,.T.);
#32307=ORIENTED_EDGE('',*,*,#22535,.T.);
#32308=ORIENTED_EDGE('',*,*,#22775,.T.);
#32309=ORIENTED_EDGE('',*,*,#22775,.F.);
#32310=ORIENTED_EDGE('',*,*,#22534,.T.);
#32311=ORIENTED_EDGE('',*,*,#22776,.F.);
#32312=ORIENTED_EDGE('',*,*,#22757,.F.);
#32313=ORIENTED_EDGE('',*,*,#22754,.T.);
#32314=ORIENTED_EDGE('',*,*,#22777,.T.);
#32315=ORIENTED_EDGE('',*,*,#22537,.T.);
#32316=ORIENTED_EDGE('',*,*,#22778,.T.);
#32317=ORIENTED_EDGE('',*,*,#22777,.F.);
#32318=ORIENTED_EDGE('',*,*,#22753,.F.);
#32319=ORIENTED_EDGE('',*,*,#22779,.F.);
#32320=ORIENTED_EDGE('',*,*,#22538,.T.);
#32321=ORIENTED_EDGE('',*,*,#22780,.T.);
#32322=ORIENTED_EDGE('',*,*,#22781,.T.);
#32323=ORIENTED_EDGE('',*,*,#22541,.T.);
#32324=ORIENTED_EDGE('',*,*,#22782,.T.);
#32325=ORIENTED_EDGE('',*,*,#22782,.F.);
#32326=ORIENTED_EDGE('',*,*,#22540,.T.);
#32327=ORIENTED_EDGE('',*,*,#22783,.F.);
#32328=ORIENTED_EDGE('',*,*,#22784,.F.);
#32329=ORIENTED_EDGE('',*,*,#22785,.F.);
#32330=ORIENTED_EDGE('',*,*,#22786,.T.);
#32331=ORIENTED_EDGE('',*,*,#22787,.F.);
#32332=ORIENTED_EDGE('',*,*,#22788,.T.);
#32333=ORIENTED_EDGE('',*,*,#22789,.T.);
#32334=ORIENTED_EDGE('',*,*,#22543,.T.);
#32335=ORIENTED_EDGE('',*,*,#22790,.T.);
#32336=ORIENTED_EDGE('',*,*,#22789,.F.);
#32337=ORIENTED_EDGE('',*,*,#22791,.T.);
#32338=ORIENTED_EDGE('',*,*,#22792,.F.);
#32339=ORIENTED_EDGE('',*,*,#22793,.F.);
#32340=ORIENTED_EDGE('',*,*,#22794,.T.);
#32341=ORIENTED_EDGE('',*,*,#22795,.F.);
#32342=ORIENTED_EDGE('',*,*,#22544,.T.);
#32343=ORIENTED_EDGE('',*,*,#22780,.F.);
#32344=ORIENTED_EDGE('',*,*,#22787,.T.);
#32345=ORIENTED_EDGE('',*,*,#22796,.T.);
#32346=ORIENTED_EDGE('',*,*,#22791,.F.);
#32347=ORIENTED_EDGE('',*,*,#22788,.F.);
#32348=ORIENTED_EDGE('',*,*,#22797,.T.);
#32349=ORIENTED_EDGE('',*,*,#22798,.T.);
#32350=ORIENTED_EDGE('',*,*,#22799,.T.);
#32351=ORIENTED_EDGE('',*,*,#22549,.T.);
#32352=ORIENTED_EDGE('',*,*,#22800,.T.);
#32353=ORIENTED_EDGE('',*,*,#22798,.F.);
#32354=ORIENTED_EDGE('',*,*,#22801,.T.);
#32355=ORIENTED_EDGE('',*,*,#22802,.F.);
#32356=ORIENTED_EDGE('',*,*,#22803,.T.);
#32357=ORIENTED_EDGE('',*,*,#22804,.F.);
#32358=ORIENTED_EDGE('',*,*,#22805,.F.);
#32359=ORIENTED_EDGE('',*,*,#22806,.F.);
#32360=ORIENTED_EDGE('',*,*,#22807,.F.);
#32361=ORIENTED_EDGE('',*,*,#22808,.F.);
#32362=ORIENTED_EDGE('',*,*,#22809,.T.);
#32363=ORIENTED_EDGE('',*,*,#22810,.F.);
#32364=ORIENTED_EDGE('',*,*,#22811,.T.);
#32365=ORIENTED_EDGE('',*,*,#22812,.F.);
#32366=ORIENTED_EDGE('',*,*,#22813,.T.);
#32367=ORIENTED_EDGE('',*,*,#22814,.F.);
#32368=ORIENTED_EDGE('',*,*,#22815,.T.);
#32369=ORIENTED_EDGE('',*,*,#22816,.F.);
#32370=ORIENTED_EDGE('',*,*,#22817,.T.);
#32371=ORIENTED_EDGE('',*,*,#22818,.F.);
#32372=ORIENTED_EDGE('',*,*,#22819,.T.);
#32373=ORIENTED_EDGE('',*,*,#22820,.F.);
#32374=ORIENTED_EDGE('',*,*,#22821,.T.);
#32375=ORIENTED_EDGE('',*,*,#22800,.F.);
#32376=ORIENTED_EDGE('',*,*,#22548,.T.);
#32377=ORIENTED_EDGE('',*,*,#22822,.F.);
#32378=ORIENTED_EDGE('',*,*,#22801,.F.);
#32379=ORIENTED_EDGE('',*,*,#22802,.T.);
#32380=ORIENTED_EDGE('',*,*,#22822,.T.);
#32381=ORIENTED_EDGE('',*,*,#22547,.T.);
#32382=ORIENTED_EDGE('',*,*,#22823,.T.);
#32383=ORIENTED_EDGE('',*,*,#22818,.T.);
#32384=ORIENTED_EDGE('',*,*,#22824,.T.);
#32385=ORIENTED_EDGE('',*,*,#22553,.T.);
#32386=ORIENTED_EDGE('',*,*,#22825,.T.);
#32387=ORIENTED_EDGE('',*,*,#22825,.F.);
#32388=ORIENTED_EDGE('',*,*,#22552,.T.);
#32389=ORIENTED_EDGE('',*,*,#22826,.F.);
#32390=ORIENTED_EDGE('',*,*,#22819,.F.);
#32391=ORIENTED_EDGE('',*,*,#22816,.T.);
#32392=ORIENTED_EDGE('',*,*,#22827,.T.);
#32393=ORIENTED_EDGE('',*,*,#22555,.T.);
#32394=ORIENTED_EDGE('',*,*,#22828,.T.);
#32395=ORIENTED_EDGE('',*,*,#22827,.F.);
#32396=ORIENTED_EDGE('',*,*,#22815,.F.);
#32397=ORIENTED_EDGE('',*,*,#22829,.F.);
#32398=ORIENTED_EDGE('',*,*,#22556,.T.);
#32399=ORIENTED_EDGE('',*,*,#22812,.T.);
#32400=ORIENTED_EDGE('',*,*,#22830,.T.);
#32401=ORIENTED_EDGE('',*,*,#22559,.T.);
#32402=ORIENTED_EDGE('',*,*,#22831,.T.);
#32403=ORIENTED_EDGE('',*,*,#22831,.F.);
#32404=ORIENTED_EDGE('',*,*,#22558,.T.);
#32405=ORIENTED_EDGE('',*,*,#22832,.F.);
#32406=ORIENTED_EDGE('',*,*,#22813,.F.);
#32407=ORIENTED_EDGE('',*,*,#22810,.T.);
#32408=ORIENTED_EDGE('',*,*,#22833,.T.);
#32409=ORIENTED_EDGE('',*,*,#22561,.T.);
#32410=ORIENTED_EDGE('',*,*,#22834,.T.);
#32411=ORIENTED_EDGE('',*,*,#22833,.F.);
#32412=ORIENTED_EDGE('',*,*,#22809,.F.);
#32413=ORIENTED_EDGE('',*,*,#22835,.F.);
#32414=ORIENTED_EDGE('',*,*,#22562,.T.);
#32415=ORIENTED_EDGE('',*,*,#22836,.T.);
#32416=ORIENTED_EDGE('',*,*,#22837,.T.);
#32417=ORIENTED_EDGE('',*,*,#22565,.T.);
#32418=ORIENTED_EDGE('',*,*,#22838,.T.);
#32419=ORIENTED_EDGE('',*,*,#22838,.F.);
#32420=ORIENTED_EDGE('',*,*,#22564,.T.);
#32421=ORIENTED_EDGE('',*,*,#22839,.F.);
#32422=ORIENTED_EDGE('',*,*,#22840,.F.);
#32423=ORIENTED_EDGE('',*,*,#22841,.F.);
#32424=ORIENTED_EDGE('',*,*,#22842,.T.);
#32425=ORIENTED_EDGE('',*,*,#22843,.F.);
#32426=ORIENTED_EDGE('',*,*,#22844,.T.);
#32427=ORIENTED_EDGE('',*,*,#22845,.T.);
#32428=ORIENTED_EDGE('',*,*,#22567,.T.);
#32429=ORIENTED_EDGE('',*,*,#22846,.T.);
#32430=ORIENTED_EDGE('',*,*,#22845,.F.);
#32431=ORIENTED_EDGE('',*,*,#22847,.T.);
#32432=ORIENTED_EDGE('',*,*,#22848,.F.);
#32433=ORIENTED_EDGE('',*,*,#22849,.F.);
#32434=ORIENTED_EDGE('',*,*,#22850,.T.);
#32435=ORIENTED_EDGE('',*,*,#22851,.F.);
#32436=ORIENTED_EDGE('',*,*,#22568,.T.);
#32437=ORIENTED_EDGE('',*,*,#22836,.F.);
#32438=ORIENTED_EDGE('',*,*,#22843,.T.);
#32439=ORIENTED_EDGE('',*,*,#22852,.T.);
#32440=ORIENTED_EDGE('',*,*,#22847,.F.);
#32441=ORIENTED_EDGE('',*,*,#22844,.F.);
#32442=ORIENTED_EDGE('',*,*,#22853,.T.);
#32443=ORIENTED_EDGE('',*,*,#22854,.T.);
#32444=ORIENTED_EDGE('',*,*,#22855,.T.);
#32445=ORIENTED_EDGE('',*,*,#22573,.T.);
#32446=ORIENTED_EDGE('',*,*,#22856,.T.);
#32447=ORIENTED_EDGE('',*,*,#22854,.F.);
#32448=ORIENTED_EDGE('',*,*,#22857,.T.);
#32449=ORIENTED_EDGE('',*,*,#22858,.F.);
#32450=ORIENTED_EDGE('',*,*,#22859,.T.);
#32451=ORIENTED_EDGE('',*,*,#22860,.F.);
#32452=ORIENTED_EDGE('',*,*,#22861,.F.);
#32453=ORIENTED_EDGE('',*,*,#22862,.F.);
#32454=ORIENTED_EDGE('',*,*,#22863,.F.);
#32455=ORIENTED_EDGE('',*,*,#22864,.F.);
#32456=ORIENTED_EDGE('',*,*,#22865,.T.);
#32457=ORIENTED_EDGE('',*,*,#22866,.F.);
#32458=ORIENTED_EDGE('',*,*,#22867,.T.);
#32459=ORIENTED_EDGE('',*,*,#22868,.F.);
#32460=ORIENTED_EDGE('',*,*,#22869,.T.);
#32461=ORIENTED_EDGE('',*,*,#22870,.F.);
#32462=ORIENTED_EDGE('',*,*,#22871,.T.);
#32463=ORIENTED_EDGE('',*,*,#22872,.F.);
#32464=ORIENTED_EDGE('',*,*,#22873,.T.);
#32465=ORIENTED_EDGE('',*,*,#22874,.F.);
#32466=ORIENTED_EDGE('',*,*,#22875,.T.);
#32467=ORIENTED_EDGE('',*,*,#22876,.F.);
#32468=ORIENTED_EDGE('',*,*,#22877,.T.);
#32469=ORIENTED_EDGE('',*,*,#22856,.F.);
#32470=ORIENTED_EDGE('',*,*,#22572,.T.);
#32471=ORIENTED_EDGE('',*,*,#22878,.F.);
#32472=ORIENTED_EDGE('',*,*,#22857,.F.);
#32473=ORIENTED_EDGE('',*,*,#22858,.T.);
#32474=ORIENTED_EDGE('',*,*,#22878,.T.);
#32475=ORIENTED_EDGE('',*,*,#22571,.T.);
#32476=ORIENTED_EDGE('',*,*,#22879,.T.);
#32477=ORIENTED_EDGE('',*,*,#22874,.T.);
#32478=ORIENTED_EDGE('',*,*,#22880,.T.);
#32479=ORIENTED_EDGE('',*,*,#22577,.T.);
#32480=ORIENTED_EDGE('',*,*,#22881,.T.);
#32481=ORIENTED_EDGE('',*,*,#22881,.F.);
#32482=ORIENTED_EDGE('',*,*,#22576,.T.);
#32483=ORIENTED_EDGE('',*,*,#22882,.F.);
#32484=ORIENTED_EDGE('',*,*,#22875,.F.);
#32485=ORIENTED_EDGE('',*,*,#22872,.T.);
#32486=ORIENTED_EDGE('',*,*,#22883,.T.);
#32487=ORIENTED_EDGE('',*,*,#22579,.T.);
#32488=ORIENTED_EDGE('',*,*,#22884,.T.);
#32489=ORIENTED_EDGE('',*,*,#22883,.F.);
#32490=ORIENTED_EDGE('',*,*,#22871,.F.);
#32491=ORIENTED_EDGE('',*,*,#22885,.F.);
#32492=ORIENTED_EDGE('',*,*,#22580,.T.);
#32493=ORIENTED_EDGE('',*,*,#22886,.T.);
#32494=ORIENTED_EDGE('',*,*,#22887,.T.);
#32495=ORIENTED_EDGE('',*,*,#22888,.T.);
#32496=ORIENTED_EDGE('',*,*,#22889,.T.);
#32497=ORIENTED_EDGE('',*,*,#22888,.F.);
#32498=ORIENTED_EDGE('',*,*,#22890,.T.);
#32499=ORIENTED_EDGE('',*,*,#22891,.T.);
#32500=ORIENTED_EDGE('',*,*,#22886,.F.);
#32501=ORIENTED_EDGE('',*,*,#22892,.T.);
#32502=ORIENTED_EDGE('',*,*,#22893,.T.);
#32503=ORIENTED_EDGE('',*,*,#22893,.F.);
#32504=ORIENTED_EDGE('',*,*,#22438,.T.);
#32505=ORIENTED_EDGE('',*,*,#22894,.T.);
#32506=ORIENTED_EDGE('',*,*,#22895,.T.);
#32507=ORIENTED_EDGE('',*,*,#22892,.F.);
#32508=ORIENTED_EDGE('',*,*,#22896,.T.);
#32509=ORIENTED_EDGE('',*,*,#22897,.T.);
#32510=ORIENTED_EDGE('',*,*,#22898,.T.);
#32511=ORIENTED_EDGE('',*,*,#22439,.T.);
#32512=ORIENTED_EDGE('',*,*,#22889,.F.);
#32513=ORIENTED_EDGE('',*,*,#22899,.F.);
#32514=ORIENTED_EDGE('',*,*,#22900,.T.);
#32515=ORIENTED_EDGE('',*,*,#22901,.T.);
#32516=ORIENTED_EDGE('',*,*,#22902,.T.);
#32517=ORIENTED_EDGE('',*,*,#22903,.F.);
#32518=ORIENTED_EDGE('',*,*,#22904,.F.);
#32519=ORIENTED_EDGE('',*,*,#22896,.F.);
#32520=ORIENTED_EDGE('',*,*,#22905,.T.);
#32521=ORIENTED_EDGE('',*,*,#22906,.T.);
#32522=ORIENTED_EDGE('',*,*,#22907,.T.);
#32523=ORIENTED_EDGE('',*,*,#22908,.T.);
#32524=ORIENTED_EDGE('',*,*,#22907,.F.);
#32525=ORIENTED_EDGE('',*,*,#22909,.T.);
#32526=ORIENTED_EDGE('',*,*,#22910,.T.);
#32527=ORIENTED_EDGE('',*,*,#22905,.F.);
#32528=ORIENTED_EDGE('',*,*,#22911,.T.);
#32529=ORIENTED_EDGE('',*,*,#22912,.T.);
#32530=ORIENTED_EDGE('',*,*,#22910,.F.);
#32531=ORIENTED_EDGE('',*,*,#22749,.T.);
#32532=ORIENTED_EDGE('',*,*,#22913,.T.);
#32533=ORIENTED_EDGE('',*,*,#22738,.F.);
#32534=ORIENTED_EDGE('',*,*,#22914,.T.);
#32535=ORIENTED_EDGE('',*,*,#22909,.F.);
#32536=ORIENTED_EDGE('',*,*,#22915,.T.);
#32537=ORIENTED_EDGE('',*,*,#22916,.F.);
#32538=ORIENTED_EDGE('',*,*,#22750,.T.);
#32539=ORIENTED_EDGE('',*,*,#22906,.F.);
#32540=ORIENTED_EDGE('',*,*,#22917,.F.);
#32541=ORIENTED_EDGE('',*,*,#22918,.F.);
#32542=ORIENTED_EDGE('',*,*,#22915,.F.);
#32543=ORIENTED_EDGE('',*,*,#22894,.F.);
#32544=ORIENTED_EDGE('',*,*,#22919,.T.);
#32545=ORIENTED_EDGE('',*,*,#22920,.T.);
#32546=ORIENTED_EDGE('',*,*,#22440,.T.);
#32547=ORIENTED_EDGE('',*,*,#22898,.F.);
#32548=ORIENTED_EDGE('',*,*,#22921,.T.);
#32549=ORIENTED_EDGE('',*,*,#22922,.T.);
#32550=ORIENTED_EDGE('',*,*,#22923,.T.);
#32551=ORIENTED_EDGE('',*,*,#22924,.T.);
#32552=ORIENTED_EDGE('',*,*,#22441,.T.);
#32553=ORIENTED_EDGE('',*,*,#22922,.F.);
#32554=ORIENTED_EDGE('',*,*,#22925,.T.);
#32555=ORIENTED_EDGE('',*,*,#22924,.F.);
#32556=ORIENTED_EDGE('',*,*,#22926,.T.);
#32557=ORIENTED_EDGE('',*,*,#22927,.T.);
#32558=ORIENTED_EDGE('',*,*,#22919,.F.);
#32559=ORIENTED_EDGE('',*,*,#22449,.T.);
#32560=ORIENTED_EDGE('',*,*,#22928,.F.);
#32561=ORIENTED_EDGE('',*,*,#22929,.T.);
#32562=ORIENTED_EDGE('',*,*,#22927,.F.);
#32563=ORIENTED_EDGE('',*,*,#22930,.T.);
#32564=ORIENTED_EDGE('',*,*,#22931,.T.);
#32565=ORIENTED_EDGE('',*,*,#22932,.F.);
#32566=ORIENTED_EDGE('',*,*,#22442,.T.);
#32567=ORIENTED_EDGE('',*,*,#22926,.F.);
#32568=ORIENTED_EDGE('',*,*,#22933,.T.);
#32569=ORIENTED_EDGE('',*,*,#22934,.T.);
#32570=ORIENTED_EDGE('',*,*,#22935,.T.);
#32571=ORIENTED_EDGE('',*,*,#22923,.F.);
#32572=ORIENTED_EDGE('',*,*,#22936,.F.);
#32573=ORIENTED_EDGE('',*,*,#22937,.F.);
#32574=ORIENTED_EDGE('',*,*,#22849,.T.);
#32575=ORIENTED_EDGE('',*,*,#22938,.T.);
#32576=ORIENTED_EDGE('',*,*,#22841,.T.);
#32577=ORIENTED_EDGE('',*,*,#22939,.F.);
#32578=ORIENTED_EDGE('',*,*,#22933,.F.);
#32579=ORIENTED_EDGE('',*,*,#22940,.T.);
#32580=ORIENTED_EDGE('',*,*,#22941,.T.);
#32581=ORIENTED_EDGE('',*,*,#22942,.T.);
#32582=ORIENTED_EDGE('',*,*,#22943,.T.);
#32583=ORIENTED_EDGE('',*,*,#22940,.F.);
#32584=ORIENTED_EDGE('',*,*,#22944,.T.);
#32585=ORIENTED_EDGE('',*,*,#22945,.T.);
#32586=ORIENTED_EDGE('',*,*,#22946,.T.);
#32587=ORIENTED_EDGE('',*,*,#22947,.T.);
#32588=ORIENTED_EDGE('',*,*,#22948,.T.);
#32589=ORIENTED_EDGE('',*,*,#22949,.T.);
#32590=ORIENTED_EDGE('',*,*,#22448,.T.);
#32591=ORIENTED_EDGE('',*,*,#22949,.F.);
#32592=ORIENTED_EDGE('',*,*,#22950,.T.);
#32593=ORIENTED_EDGE('',*,*,#22928,.T.);
#32594=ORIENTED_EDGE('',*,*,#22946,.F.);
#32595=ORIENTED_EDGE('',*,*,#22951,.T.);
#32596=ORIENTED_EDGE('',*,*,#22942,.F.);
#32597=ORIENTED_EDGE('',*,*,#22945,.F.);
#32598=ORIENTED_EDGE('',*,*,#22638,.T.);
#32599=ORIENTED_EDGE('',*,*,#22952,.F.);
#32600=ORIENTED_EDGE('',*,*,#22953,.T.);
#32601=ORIENTED_EDGE('',*,*,#22944,.F.);
#32602=ORIENTED_EDGE('',*,*,#22954,.T.);
#32603=ORIENTED_EDGE('',*,*,#22672,.T.);
#32604=ORIENTED_EDGE('',*,*,#22955,.T.);
#32605=ORIENTED_EDGE('',*,*,#22639,.T.);
#32606=ORIENTED_EDGE('',*,*,#22943,.F.);
#32607=ORIENTED_EDGE('',*,*,#22956,.F.);
#32608=ORIENTED_EDGE('',*,*,#22957,.F.);
#32609=ORIENTED_EDGE('',*,*,#22958,.F.);
#32610=ORIENTED_EDGE('',*,*,#22681,.T.);
#32611=ORIENTED_EDGE('',*,*,#22959,.T.);
#32612=ORIENTED_EDGE('',*,*,#22673,.T.);
#32613=ORIENTED_EDGE('',*,*,#22954,.F.);
#32614=ORIENTED_EDGE('',*,*,#22951,.F.);
#32615=ORIENTED_EDGE('',*,*,#22447,.T.);
#32616=ORIENTED_EDGE('',*,*,#22960,.F.);
#32617=ORIENTED_EDGE('',*,*,#22956,.T.);
#32618=ORIENTED_EDGE('',*,*,#22961,.T.);
#32619=ORIENTED_EDGE('',*,*,#22962,.T.);
#32620=ORIENTED_EDGE('',*,*,#22963,.T.);
#32621=ORIENTED_EDGE('',*,*,#22957,.T.);
#32622=ORIENTED_EDGE('',*,*,#22963,.F.);
#32623=ORIENTED_EDGE('',*,*,#22964,.T.);
#32624=ORIENTED_EDGE('',*,*,#22965,.T.);
#32625=ORIENTED_EDGE('',*,*,#22961,.F.);
#32626=ORIENTED_EDGE('',*,*,#22960,.T.);
#32627=ORIENTED_EDGE('',*,*,#22966,.T.);
#32628=ORIENTED_EDGE('',*,*,#22965,.F.);
#32629=ORIENTED_EDGE('',*,*,#22693,.T.);
#32630=ORIENTED_EDGE('',*,*,#22967,.T.);
#32631=ORIENTED_EDGE('',*,*,#22682,.F.);
#32632=ORIENTED_EDGE('',*,*,#22958,.T.);
#32633=ORIENTED_EDGE('',*,*,#22964,.F.);
#32634=ORIENTED_EDGE('',*,*,#22968,.T.);
#32635=ORIENTED_EDGE('',*,*,#22969,.F.);
#32636=ORIENTED_EDGE('',*,*,#22694,.T.);
#32637=ORIENTED_EDGE('',*,*,#22962,.F.);
#32638=ORIENTED_EDGE('',*,*,#22970,.F.);
#32639=ORIENTED_EDGE('',*,*,#22971,.F.);
#32640=ORIENTED_EDGE('',*,*,#22972,.T.);
#32641=ORIENTED_EDGE('',*,*,#22973,.F.);
#32642=ORIENTED_EDGE('',*,*,#22968,.F.);
#32643=ORIENTED_EDGE('',*,*,#22966,.F.);
#32644=ORIENTED_EDGE('',*,*,#22446,.T.);
#32645=ORIENTED_EDGE('',*,*,#22974,.T.);
#32646=ORIENTED_EDGE('',*,*,#22970,.T.);
#32647=ORIENTED_EDGE('',*,*,#22912,.F.);
#32648=ORIENTED_EDGE('',*,*,#22444,.T.);
#32649=ORIENTED_EDGE('',*,*,#22975,.T.);
#32650=ORIENTED_EDGE('',*,*,#22917,.T.);
#32651=ORIENTED_EDGE('',*,*,#22976,.T.);
#32652=ORIENTED_EDGE('',*,*,#22977,.T.);
#32653=ORIENTED_EDGE('',*,*,#22975,.F.);
#32654=ORIENTED_EDGE('',*,*,#22911,.F.);
#32655=ORIENTED_EDGE('',*,*,#22978,.T.);
#32656=ORIENTED_EDGE('',*,*,#22971,.T.);
#32657=ORIENTED_EDGE('',*,*,#22974,.F.);
#32658=ORIENTED_EDGE('',*,*,#22445,.T.);
#32659=ORIENTED_EDGE('',*,*,#22908,.F.);
#32660=ORIENTED_EDGE('',*,*,#22914,.F.);
#32661=ORIENTED_EDGE('',*,*,#22737,.T.);
#32662=ORIENTED_EDGE('',*,*,#22979,.T.);
#32663=ORIENTED_EDGE('',*,*,#22729,.T.);
#32664=ORIENTED_EDGE('',*,*,#22980,.F.);
#32665=ORIENTED_EDGE('',*,*,#22972,.F.);
#32666=ORIENTED_EDGE('',*,*,#22978,.F.);
#32667=ORIENTED_EDGE('',*,*,#22934,.F.);
#32668=ORIENTED_EDGE('',*,*,#22981,.F.);
#32669=ORIENTED_EDGE('',*,*,#22982,.F.);
#32670=ORIENTED_EDGE('',*,*,#22983,.T.);
#32671=ORIENTED_EDGE('',*,*,#22807,.T.);
#32672=ORIENTED_EDGE('',*,*,#22981,.T.);
#32673=ORIENTED_EDGE('',*,*,#22939,.T.);
#32674=ORIENTED_EDGE('',*,*,#22840,.T.);
#32675=ORIENTED_EDGE('',*,*,#22984,.T.);
#32676=ORIENTED_EDGE('',*,*,#22985,.T.);
#32677=ORIENTED_EDGE('',*,*,#22986,.T.);
#32678=ORIENTED_EDGE('',*,*,#22984,.F.);
#32679=ORIENTED_EDGE('',*,*,#22987,.T.);
#32680=ORIENTED_EDGE('',*,*,#22982,.T.);
#32681=ORIENTED_EDGE('',*,*,#22806,.T.);
#32682=ORIENTED_EDGE('',*,*,#22932,.T.);
#32683=ORIENTED_EDGE('',*,*,#22988,.T.);
#32684=ORIENTED_EDGE('',*,*,#22989,.T.);
#32685=ORIENTED_EDGE('',*,*,#22976,.F.);
#32686=ORIENTED_EDGE('',*,*,#22443,.T.);
#32687=ORIENTED_EDGE('',*,*,#22989,.F.);
#32688=ORIENTED_EDGE('',*,*,#22990,.T.);
#32689=ORIENTED_EDGE('',*,*,#22985,.F.);
#32690=ORIENTED_EDGE('',*,*,#22805,.T.);
#32691=ORIENTED_EDGE('',*,*,#22991,.T.);
#32692=ORIENTED_EDGE('',*,*,#22794,.F.);
#32693=ORIENTED_EDGE('',*,*,#22992,.T.);
#32694=ORIENTED_EDGE('',*,*,#22986,.F.);
#32695=ORIENTED_EDGE('',*,*,#22993,.T.);
#32696=ORIENTED_EDGE('',*,*,#22988,.F.);
#32697=ORIENTED_EDGE('',*,*,#22994,.T.);
#32698=ORIENTED_EDGE('',*,*,#22977,.F.);
#32699=ORIENTED_EDGE('',*,*,#22995,.T.);
#32700=ORIENTED_EDGE('',*,*,#22996,.T.);
#32701=ORIENTED_EDGE('',*,*,#22918,.T.);
#32702=ORIENTED_EDGE('',*,*,#22996,.F.);
#32703=ORIENTED_EDGE('',*,*,#22997,.T.);
#32704=ORIENTED_EDGE('',*,*,#22916,.T.);
#32705=ORIENTED_EDGE('',*,*,#22991,.F.);
#32706=ORIENTED_EDGE('',*,*,#22804,.T.);
#32707=ORIENTED_EDGE('',*,*,#22998,.T.);
#32708=ORIENTED_EDGE('',*,*,#22545,.F.);
#32709=ORIENTED_EDGE('',*,*,#22795,.T.);
#32710=ORIENTED_EDGE('',*,*,#22987,.F.);
#32711=ORIENTED_EDGE('',*,*,#22994,.F.);
#32712=ORIENTED_EDGE('',*,*,#22931,.F.);
#32713=ORIENTED_EDGE('',*,*,#22999,.T.);
#32714=ORIENTED_EDGE('',*,*,#22999,.F.);
#32715=ORIENTED_EDGE('',*,*,#22930,.F.);
#32716=ORIENTED_EDGE('',*,*,#22935,.F.);
#32717=ORIENTED_EDGE('',*,*,#22997,.F.);
#32718=ORIENTED_EDGE('',*,*,#23000,.T.);
#32719=ORIENTED_EDGE('',*,*,#22784,.T.);
#32720=ORIENTED_EDGE('',*,*,#23001,.T.);
#32721=ORIENTED_EDGE('',*,*,#22751,.T.);
#32722=ORIENTED_EDGE('',*,*,#22992,.F.);
#32723=ORIENTED_EDGE('',*,*,#22793,.T.);
#32724=ORIENTED_EDGE('',*,*,#23002,.T.);
#32725=ORIENTED_EDGE('',*,*,#22785,.T.);
#32726=ORIENTED_EDGE('',*,*,#23000,.F.);
#32727=ORIENTED_EDGE('',*,*,#22995,.F.);
#32728=ORIENTED_EDGE('',*,*,#22990,.F.);
#32729=ORIENTED_EDGE('',*,*,#22993,.F.);
#32730=ORIENTED_EDGE('',*,*,#22980,.T.);
#32731=ORIENTED_EDGE('',*,*,#22728,.T.);
#32732=ORIENTED_EDGE('',*,*,#23003,.T.);
#32733=ORIENTED_EDGE('',*,*,#22695,.T.);
#32734=ORIENTED_EDGE('',*,*,#22969,.T.);
#32735=ORIENTED_EDGE('',*,*,#22973,.T.);
#32736=ORIENTED_EDGE('',*,*,#22952,.T.);
#32737=ORIENTED_EDGE('',*,*,#23004,.T.);
#32738=ORIENTED_EDGE('',*,*,#23005,.T.);
#32739=ORIENTED_EDGE('',*,*,#22941,.F.);
#32740=ORIENTED_EDGE('',*,*,#22953,.F.);
#32741=ORIENTED_EDGE('',*,*,#23006,.F.);
#32742=ORIENTED_EDGE('',*,*,#22948,.F.);
#32743=ORIENTED_EDGE('',*,*,#23007,.F.);
#32744=ORIENTED_EDGE('',*,*,#23007,.T.);
#32745=ORIENTED_EDGE('',*,*,#22947,.F.);
#32746=ORIENTED_EDGE('',*,*,#22950,.F.);
#32747=ORIENTED_EDGE('',*,*,#23006,.T.);
#32748=ORIENTED_EDGE('',*,*,#23005,.F.);
#32749=ORIENTED_EDGE('',*,*,#23008,.T.);
#32750=ORIENTED_EDGE('',*,*,#23004,.F.);
#32751=ORIENTED_EDGE('',*,*,#22637,.T.);
#32752=ORIENTED_EDGE('',*,*,#23009,.T.);
#32753=ORIENTED_EDGE('',*,*,#23010,.F.);
#32754=ORIENTED_EDGE('',*,*,#23011,.T.);
#32755=ORIENTED_EDGE('',*,*,#22920,.F.);
#32756=ORIENTED_EDGE('',*,*,#23012,.T.);
#32757=ORIENTED_EDGE('',*,*,#23013,.T.);
#32758=ORIENTED_EDGE('',*,*,#23014,.T.);
#32759=ORIENTED_EDGE('',*,*,#23013,.F.);
#32760=ORIENTED_EDGE('',*,*,#23015,.T.);
#32761=ORIENTED_EDGE('',*,*,#23016,.T.);
#32762=ORIENTED_EDGE('',*,*,#23009,.F.);
#32763=ORIENTED_EDGE('',*,*,#22636,.T.);
#32764=ORIENTED_EDGE('',*,*,#23017,.T.);
#32765=ORIENTED_EDGE('',*,*,#22473,.F.);
#32766=ORIENTED_EDGE('',*,*,#23018,.T.);
#32767=ORIENTED_EDGE('',*,*,#23015,.F.);
#32768=ORIENTED_EDGE('',*,*,#23019,.T.);
#32769=ORIENTED_EDGE('',*,*,#23020,.T.);
#32770=ORIENTED_EDGE('',*,*,#23021,.T.);
#32771=ORIENTED_EDGE('',*,*,#22597,.T.);
#32772=ORIENTED_EDGE('',*,*,#22890,.F.);
#32773=ORIENTED_EDGE('',*,*,#23022,.T.);
#32774=ORIENTED_EDGE('',*,*,#23016,.F.);
#32775=ORIENTED_EDGE('',*,*,#22596,.T.);
#32776=ORIENTED_EDGE('',*,*,#22891,.F.);
#32777=ORIENTED_EDGE('',*,*,#22595,.T.);
#32778=ORIENTED_EDGE('',*,*,#23023,.T.);
#32779=ORIENTED_EDGE('',*,*,#23024,.F.);
#32780=ORIENTED_EDGE('',*,*,#22899,.T.);
#32781=ORIENTED_EDGE('',*,*,#23011,.F.);
#32782=ORIENTED_EDGE('',*,*,#23025,.T.);
#32783=ORIENTED_EDGE('',*,*,#23026,.T.);
#32784=ORIENTED_EDGE('',*,*,#23027,.T.);
#32785=ORIENTED_EDGE('',*,*,#23019,.F.);
#32786=ORIENTED_EDGE('',*,*,#23012,.F.);
#32787=ORIENTED_EDGE('',*,*,#22929,.F.);
#32788=ORIENTED_EDGE('',*,*,#23008,.F.);
#32789=ORIENTED_EDGE('',*,*,#22887,.F.);
#32790=ORIENTED_EDGE('',*,*,#22895,.F.);
#32791=ORIENTED_EDGE('',*,*,#23014,.F.);
#32792=ORIENTED_EDGE('',*,*,#23022,.F.);
#32793=ORIENTED_EDGE('',*,*,#22903,.T.);
#32794=ORIENTED_EDGE('',*,*,#23028,.T.);
#32795=ORIENTED_EDGE('',*,*,#23029,.T.);
#32796=ORIENTED_EDGE('',*,*,#22863,.T.);
#32797=ORIENTED_EDGE('',*,*,#23030,.T.);
#32798=ORIENTED_EDGE('',*,*,#23031,.T.);
#32799=ORIENTED_EDGE('',*,*,#22862,.T.);
#32800=ORIENTED_EDGE('',*,*,#23032,.T.);
#32801=ORIENTED_EDGE('',*,*,#23033,.T.);
#32802=ORIENTED_EDGE('',*,*,#23030,.F.);
#32803=ORIENTED_EDGE('',*,*,#22861,.T.);
#32804=ORIENTED_EDGE('',*,*,#23034,.T.);
#32805=ORIENTED_EDGE('',*,*,#22850,.F.);
#32806=ORIENTED_EDGE('',*,*,#22937,.T.);
#32807=ORIENTED_EDGE('',*,*,#23035,.T.);
#32808=ORIENTED_EDGE('',*,*,#23032,.F.);
#32809=ORIENTED_EDGE('',*,*,#22897,.F.);
#32810=ORIENTED_EDGE('',*,*,#22904,.T.);
#32811=ORIENTED_EDGE('',*,*,#23031,.F.);
#32812=ORIENTED_EDGE('',*,*,#23033,.F.);
#32813=ORIENTED_EDGE('',*,*,#23035,.F.);
#32814=ORIENTED_EDGE('',*,*,#22936,.T.);
#32815=ORIENTED_EDGE('',*,*,#22925,.F.);
#32816=ORIENTED_EDGE('',*,*,#22921,.F.);
#32817=ORIENTED_EDGE('',*,*,#22868,.T.);
#32818=ORIENTED_EDGE('',*,*,#23036,.T.);
#32819=ORIENTED_EDGE('',*,*,#22583,.T.);
#32820=ORIENTED_EDGE('',*,*,#23037,.T.);
#32821=ORIENTED_EDGE('',*,*,#23036,.F.);
#32822=ORIENTED_EDGE('',*,*,#22867,.F.);
#32823=ORIENTED_EDGE('',*,*,#23038,.F.);
#32824=ORIENTED_EDGE('',*,*,#22584,.T.);
#32825=ORIENTED_EDGE('',*,*,#22866,.T.);
#32826=ORIENTED_EDGE('',*,*,#23039,.T.);
#32827=ORIENTED_EDGE('',*,*,#22585,.T.);
#32828=ORIENTED_EDGE('',*,*,#23038,.T.);
#32829=ORIENTED_EDGE('',*,*,#23039,.F.);
#32830=ORIENTED_EDGE('',*,*,#22865,.F.);
#32831=ORIENTED_EDGE('',*,*,#23040,.F.);
#32832=ORIENTED_EDGE('',*,*,#22586,.T.);
#32833=ORIENTED_EDGE('',*,*,#23037,.F.);
#32834=ORIENTED_EDGE('',*,*,#22582,.T.);
#32835=ORIENTED_EDGE('',*,*,#23041,.F.);
#32836=ORIENTED_EDGE('',*,*,#22869,.F.);
#32837=ORIENTED_EDGE('',*,*,#23041,.T.);
#32838=ORIENTED_EDGE('',*,*,#22581,.F.);
#32839=ORIENTED_EDGE('',*,*,#22885,.T.);
#32840=ORIENTED_EDGE('',*,*,#22870,.T.);
#32841=ORIENTED_EDGE('',*,*,#22880,.F.);
#32842=ORIENTED_EDGE('',*,*,#22873,.F.);
#32843=ORIENTED_EDGE('',*,*,#22884,.F.);
#32844=ORIENTED_EDGE('',*,*,#22578,.T.);
#32845=ORIENTED_EDGE('',*,*,#23029,.F.);
#32846=ORIENTED_EDGE('',*,*,#23042,.T.);
#32847=ORIENTED_EDGE('',*,*,#22587,.F.);
#32848=ORIENTED_EDGE('',*,*,#23040,.T.);
#32849=ORIENTED_EDGE('',*,*,#22864,.T.);
#32850=ORIENTED_EDGE('',*,*,#22882,.T.);
#32851=ORIENTED_EDGE('',*,*,#22575,.F.);
#32852=ORIENTED_EDGE('',*,*,#23043,.T.);
#32853=ORIENTED_EDGE('',*,*,#22876,.T.);
#32854=ORIENTED_EDGE('',*,*,#22879,.F.);
#32855=ORIENTED_EDGE('',*,*,#22570,.T.);
#32856=ORIENTED_EDGE('',*,*,#23044,.F.);
#32857=ORIENTED_EDGE('',*,*,#22859,.F.);
#32858=ORIENTED_EDGE('',*,*,#22855,.F.);
#32859=ORIENTED_EDGE('',*,*,#22877,.F.);
#32860=ORIENTED_EDGE('',*,*,#23043,.F.);
#32861=ORIENTED_EDGE('',*,*,#22574,.T.);
#32862=ORIENTED_EDGE('',*,*,#22938,.F.);
#32863=ORIENTED_EDGE('',*,*,#22848,.T.);
#32864=ORIENTED_EDGE('',*,*,#22852,.F.);
#32865=ORIENTED_EDGE('',*,*,#22842,.F.);
#32866=ORIENTED_EDGE('',*,*,#22837,.F.);
#32867=ORIENTED_EDGE('',*,*,#22853,.F.);
#32868=ORIENTED_EDGE('',*,*,#22846,.F.);
#32869=ORIENTED_EDGE('',*,*,#22566,.T.);
#32870=ORIENTED_EDGE('',*,*,#22983,.F.);
#32871=ORIENTED_EDGE('',*,*,#22839,.T.);
#32872=ORIENTED_EDGE('',*,*,#22563,.F.);
#32873=ORIENTED_EDGE('',*,*,#22835,.T.);
#32874=ORIENTED_EDGE('',*,*,#22808,.T.);
#32875=ORIENTED_EDGE('',*,*,#22830,.F.);
#32876=ORIENTED_EDGE('',*,*,#22811,.F.);
#32877=ORIENTED_EDGE('',*,*,#22834,.F.);
#32878=ORIENTED_EDGE('',*,*,#22560,.T.);
#32879=ORIENTED_EDGE('',*,*,#22832,.T.);
#32880=ORIENTED_EDGE('',*,*,#22557,.F.);
#32881=ORIENTED_EDGE('',*,*,#22829,.T.);
#32882=ORIENTED_EDGE('',*,*,#22814,.T.);
#32883=ORIENTED_EDGE('',*,*,#22824,.F.);
#32884=ORIENTED_EDGE('',*,*,#22817,.F.);
#32885=ORIENTED_EDGE('',*,*,#22828,.F.);
#32886=ORIENTED_EDGE('',*,*,#22554,.T.);
#32887=ORIENTED_EDGE('',*,*,#23034,.F.);
#32888=ORIENTED_EDGE('',*,*,#22860,.T.);
#32889=ORIENTED_EDGE('',*,*,#23044,.T.);
#32890=ORIENTED_EDGE('',*,*,#22569,.F.);
#32891=ORIENTED_EDGE('',*,*,#22851,.T.);
#32892=ORIENTED_EDGE('',*,*,#22826,.T.);
#32893=ORIENTED_EDGE('',*,*,#22551,.F.);
#32894=ORIENTED_EDGE('',*,*,#23045,.T.);
#32895=ORIENTED_EDGE('',*,*,#22820,.T.);
#32896=ORIENTED_EDGE('',*,*,#22823,.F.);
#32897=ORIENTED_EDGE('',*,*,#22546,.T.);
#32898=ORIENTED_EDGE('',*,*,#22998,.F.);
#32899=ORIENTED_EDGE('',*,*,#22803,.F.);
#32900=ORIENTED_EDGE('',*,*,#22799,.F.);
#32901=ORIENTED_EDGE('',*,*,#22821,.F.);
#32902=ORIENTED_EDGE('',*,*,#23045,.F.);
#32903=ORIENTED_EDGE('',*,*,#22550,.T.);
#32904=ORIENTED_EDGE('',*,*,#23002,.F.);
#32905=ORIENTED_EDGE('',*,*,#22792,.T.);
#32906=ORIENTED_EDGE('',*,*,#22796,.F.);
#32907=ORIENTED_EDGE('',*,*,#22786,.F.);
#32908=ORIENTED_EDGE('',*,*,#22781,.F.);
#32909=ORIENTED_EDGE('',*,*,#22797,.F.);
#32910=ORIENTED_EDGE('',*,*,#22790,.F.);
#32911=ORIENTED_EDGE('',*,*,#22542,.T.);
#32912=ORIENTED_EDGE('',*,*,#23001,.F.);
#32913=ORIENTED_EDGE('',*,*,#22783,.T.);
#32914=ORIENTED_EDGE('',*,*,#22539,.F.);
#32915=ORIENTED_EDGE('',*,*,#22779,.T.);
#32916=ORIENTED_EDGE('',*,*,#22752,.T.);
#32917=ORIENTED_EDGE('',*,*,#22774,.F.);
#32918=ORIENTED_EDGE('',*,*,#22755,.F.);
#32919=ORIENTED_EDGE('',*,*,#22778,.F.);
#32920=ORIENTED_EDGE('',*,*,#22536,.T.);
#32921=ORIENTED_EDGE('',*,*,#22776,.T.);
#32922=ORIENTED_EDGE('',*,*,#22533,.F.);
#32923=ORIENTED_EDGE('',*,*,#22773,.T.);
#32924=ORIENTED_EDGE('',*,*,#22758,.T.);
#32925=ORIENTED_EDGE('',*,*,#22768,.F.);
#32926=ORIENTED_EDGE('',*,*,#22761,.F.);
#32927=ORIENTED_EDGE('',*,*,#22772,.F.);
#32928=ORIENTED_EDGE('',*,*,#22530,.T.);
#32929=ORIENTED_EDGE('',*,*,#22770,.T.);
#32930=ORIENTED_EDGE('',*,*,#22527,.F.);
#32931=ORIENTED_EDGE('',*,*,#23046,.T.);
#32932=ORIENTED_EDGE('',*,*,#22764,.T.);
#32933=ORIENTED_EDGE('',*,*,#22767,.F.);
#32934=ORIENTED_EDGE('',*,*,#22522,.T.);
#32935=ORIENTED_EDGE('',*,*,#23047,.F.);
#32936=ORIENTED_EDGE('',*,*,#22747,.F.);
#32937=ORIENTED_EDGE('',*,*,#22743,.F.);
#32938=ORIENTED_EDGE('',*,*,#22765,.F.);
#32939=ORIENTED_EDGE('',*,*,#23046,.F.);
#32940=ORIENTED_EDGE('',*,*,#22526,.T.);
#32941=ORIENTED_EDGE('',*,*,#22979,.F.);
#32942=ORIENTED_EDGE('',*,*,#22736,.T.);
#32943=ORIENTED_EDGE('',*,*,#22740,.F.);
#32944=ORIENTED_EDGE('',*,*,#22730,.F.);
#32945=ORIENTED_EDGE('',*,*,#22725,.F.);
#32946=ORIENTED_EDGE('',*,*,#22741,.F.);
#32947=ORIENTED_EDGE('',*,*,#22734,.F.);
#32948=ORIENTED_EDGE('',*,*,#22518,.T.);
#32949=ORIENTED_EDGE('',*,*,#23003,.F.);
#32950=ORIENTED_EDGE('',*,*,#22727,.T.);
#32951=ORIENTED_EDGE('',*,*,#22515,.F.);
#32952=ORIENTED_EDGE('',*,*,#22723,.T.);
#32953=ORIENTED_EDGE('',*,*,#22696,.T.);
#32954=ORIENTED_EDGE('',*,*,#22718,.F.);
#32955=ORIENTED_EDGE('',*,*,#22699,.F.);
#32956=ORIENTED_EDGE('',*,*,#22722,.F.);
#32957=ORIENTED_EDGE('',*,*,#22512,.T.);
#32958=ORIENTED_EDGE('',*,*,#22720,.T.);
#32959=ORIENTED_EDGE('',*,*,#22509,.F.);
#32960=ORIENTED_EDGE('',*,*,#22717,.T.);
#32961=ORIENTED_EDGE('',*,*,#22702,.T.);
#32962=ORIENTED_EDGE('',*,*,#22712,.F.);
#32963=ORIENTED_EDGE('',*,*,#22705,.F.);
#32964=ORIENTED_EDGE('',*,*,#22716,.F.);
#32965=ORIENTED_EDGE('',*,*,#22506,.T.);
#32966=ORIENTED_EDGE('',*,*,#22913,.F.);
#32967=ORIENTED_EDGE('',*,*,#22748,.T.);
#32968=ORIENTED_EDGE('',*,*,#23047,.T.);
#32969=ORIENTED_EDGE('',*,*,#22521,.F.);
#32970=ORIENTED_EDGE('',*,*,#22739,.T.);
#32971=ORIENTED_EDGE('',*,*,#22714,.T.);
#32972=ORIENTED_EDGE('',*,*,#22503,.F.);
#32973=ORIENTED_EDGE('',*,*,#23048,.T.);
#32974=ORIENTED_EDGE('',*,*,#22708,.T.);
#32975=ORIENTED_EDGE('',*,*,#22711,.F.);
#32976=ORIENTED_EDGE('',*,*,#22498,.T.);
#32977=ORIENTED_EDGE('',*,*,#23049,.F.);
#32978=ORIENTED_EDGE('',*,*,#22691,.F.);
#32979=ORIENTED_EDGE('',*,*,#22687,.F.);
#32980=ORIENTED_EDGE('',*,*,#22709,.F.);
#32981=ORIENTED_EDGE('',*,*,#23048,.F.);
#32982=ORIENTED_EDGE('',*,*,#22502,.T.);
#32983=ORIENTED_EDGE('',*,*,#22959,.F.);
#32984=ORIENTED_EDGE('',*,*,#22680,.T.);
#32985=ORIENTED_EDGE('',*,*,#22684,.F.);
#32986=ORIENTED_EDGE('',*,*,#22674,.F.);
#32987=ORIENTED_EDGE('',*,*,#22669,.F.);
#32988=ORIENTED_EDGE('',*,*,#22685,.F.);
#32989=ORIENTED_EDGE('',*,*,#22678,.F.);
#32990=ORIENTED_EDGE('',*,*,#22494,.T.);
#32991=ORIENTED_EDGE('',*,*,#22955,.F.);
#32992=ORIENTED_EDGE('',*,*,#22671,.T.);
#32993=ORIENTED_EDGE('',*,*,#22491,.F.);
#32994=ORIENTED_EDGE('',*,*,#22667,.T.);
#32995=ORIENTED_EDGE('',*,*,#22640,.T.);
#32996=ORIENTED_EDGE('',*,*,#22662,.F.);
#32997=ORIENTED_EDGE('',*,*,#22643,.F.);
#32998=ORIENTED_EDGE('',*,*,#22666,.F.);
#32999=ORIENTED_EDGE('',*,*,#22488,.T.);
#33000=ORIENTED_EDGE('',*,*,#22664,.T.);
#33001=ORIENTED_EDGE('',*,*,#22485,.F.);
#33002=ORIENTED_EDGE('',*,*,#22661,.T.);
#33003=ORIENTED_EDGE('',*,*,#22646,.T.);
#33004=ORIENTED_EDGE('',*,*,#22656,.F.);
#33005=ORIENTED_EDGE('',*,*,#22649,.F.);
#33006=ORIENTED_EDGE('',*,*,#22660,.F.);
#33007=ORIENTED_EDGE('',*,*,#22482,.T.);
#33008=ORIENTED_EDGE('',*,*,#22967,.F.);
#33009=ORIENTED_EDGE('',*,*,#22692,.T.);
#33010=ORIENTED_EDGE('',*,*,#23049,.T.);
#33011=ORIENTED_EDGE('',*,*,#22497,.F.);
#33012=ORIENTED_EDGE('',*,*,#22683,.T.);
#33013=ORIENTED_EDGE('',*,*,#22658,.T.);
#33014=ORIENTED_EDGE('',*,*,#22479,.F.);
#33015=ORIENTED_EDGE('',*,*,#23050,.T.);
#33016=ORIENTED_EDGE('',*,*,#22652,.T.);
#33017=ORIENTED_EDGE('',*,*,#22655,.F.);
#33018=ORIENTED_EDGE('',*,*,#22474,.T.);
#33019=ORIENTED_EDGE('',*,*,#23017,.F.);
#33020=ORIENTED_EDGE('',*,*,#22635,.F.);
#33021=ORIENTED_EDGE('',*,*,#22631,.F.);
#33022=ORIENTED_EDGE('',*,*,#22653,.F.);
#33023=ORIENTED_EDGE('',*,*,#23050,.F.);
#33024=ORIENTED_EDGE('',*,*,#22478,.T.);
#33025=ORIENTED_EDGE('',*,*,#23026,.F.);
#33026=ORIENTED_EDGE('',*,*,#23051,.T.);
#33027=ORIENTED_EDGE('',*,*,#22626,.F.);
#33028=ORIENTED_EDGE('',*,*,#23052,.F.);
#33029=ORIENTED_EDGE('',*,*,#22629,.F.);
#33030=ORIENTED_EDGE('',*,*,#22468,.T.);
#33031=ORIENTED_EDGE('',*,*,#23053,.F.);
#33032=ORIENTED_EDGE('',*,*,#23020,.F.);
#33033=ORIENTED_EDGE('',*,*,#23027,.F.);
#33034=ORIENTED_EDGE('',*,*,#23052,.T.);
#33035=ORIENTED_EDGE('',*,*,#22625,.F.);
#33036=ORIENTED_EDGE('',*,*,#22621,.F.);
#33037=ORIENTED_EDGE('',*,*,#22627,.T.);
#33038=ORIENTED_EDGE('',*,*,#23051,.F.);
#33039=ORIENTED_EDGE('',*,*,#23025,.F.);
#33040=ORIENTED_EDGE('',*,*,#23010,.T.);
#33041=ORIENTED_EDGE('',*,*,#23018,.F.);
#33042=ORIENTED_EDGE('',*,*,#22472,.T.);
#33043=ORIENTED_EDGE('',*,*,#23021,.F.);
#33044=ORIENTED_EDGE('',*,*,#23053,.T.);
#33045=ORIENTED_EDGE('',*,*,#22467,.F.);
#33046=ORIENTED_EDGE('',*,*,#23054,.T.);
#33047=ORIENTED_EDGE('',*,*,#22598,.T.);
#33048=ORIENTED_EDGE('',*,*,#22619,.F.);
#33049=ORIENTED_EDGE('',*,*,#22462,.T.);
#33050=ORIENTED_EDGE('',*,*,#23055,.F.);
#33051=ORIENTED_EDGE('',*,*,#22603,.F.);
#33052=ORIENTED_EDGE('',*,*,#22616,.F.);
#33053=ORIENTED_EDGE('',*,*,#22599,.F.);
#33054=ORIENTED_EDGE('',*,*,#23054,.F.);
#33055=ORIENTED_EDGE('',*,*,#22466,.T.);
#33056=ORIENTED_EDGE('',*,*,#22615,.F.);
#33057=ORIENTED_EDGE('',*,*,#22605,.F.);
#33058=ORIENTED_EDGE('',*,*,#23056,.F.);
#33059=ORIENTED_EDGE('',*,*,#22460,.T.);
#33060=ORIENTED_EDGE('',*,*,#22613,.F.);
#33061=ORIENTED_EDGE('',*,*,#22456,.T.);
#33062=ORIENTED_EDGE('',*,*,#23057,.F.);
#33063=ORIENTED_EDGE('',*,*,#22609,.F.);
#33064=ORIENTED_EDGE('',*,*,#23057,.T.);
#33065=ORIENTED_EDGE('',*,*,#22455,.F.);
#33066=ORIENTED_EDGE('',*,*,#22593,.T.);
#33067=ORIENTED_EDGE('',*,*,#22610,.T.);
#33068=ORIENTED_EDGE('',*,*,#22432,.F.);
#33069=ORIENTED_EDGE('',*,*,#22611,.F.);
#33070=ORIENTED_EDGE('',*,*,#22591,.F.);
#33071=ORIENTED_EDGE('',*,*,#22452,.T.);
#33072=ORIENTED_EDGE('',*,*,#23055,.T.);
#33073=ORIENTED_EDGE('',*,*,#22461,.F.);
#33074=ORIENTED_EDGE('',*,*,#23056,.T.);
#33075=ORIENTED_EDGE('',*,*,#22604,.T.);
#33076=ORIENTED_EDGE('',*,*,#23023,.F.);
#33077=ORIENTED_EDGE('',*,*,#22594,.T.);
#33078=ORIENTED_EDGE('',*,*,#22436,.T.);
#33079=ORIENTED_EDGE('',*,*,#22451,.F.);
#33080=ORIENTED_EDGE('',*,*,#23058,.T.);
#33081=ORIENTED_EDGE('',*,*,#22430,.F.);
#33082=ORIENTED_EDGE('',*,*,#22588,.T.);
#33083=ORIENTED_EDGE('',*,*,#23042,.F.);
#33084=ORIENTED_EDGE('',*,*,#23028,.F.);
#33085=ORIENTED_EDGE('',*,*,#22902,.F.);
#33086=ORIENTED_EDGE('',*,*,#23059,.T.);
#33087=ORIENTED_EDGE('',*,*,#22424,.F.);
#33088=ORIENTED_EDGE('',*,*,#22901,.F.);
#33089=ORIENTED_EDGE('',*,*,#23060,.T.);
#33090=ORIENTED_EDGE('',*,*,#22425,.F.);
#33091=ORIENTED_EDGE('',*,*,#23059,.F.);
#33092=ORIENTED_EDGE('',*,*,#22419,.F.);
#33093=ORIENTED_EDGE('',*,*,#22426,.T.);
#33094=ORIENTED_EDGE('',*,*,#23060,.F.);
#33095=ORIENTED_EDGE('',*,*,#22900,.F.);
#33096=ORIENTED_EDGE('',*,*,#23024,.T.);
#33097=ORIENTED_EDGE('',*,*,#23058,.F.);
#33098=ORIENTED_EDGE('',*,*,#22450,.T.);
#37698=CYLINDRICAL_SURFACE('',#43276,0.4);
#37699=CYLINDRICAL_SURFACE('',#43282,0.4);
#37700=CYLINDRICAL_SURFACE('',#43284,0.4);
#37701=CYLINDRICAL_SURFACE('',#43364,0.4);
#37702=CYLINDRICAL_SURFACE('',#43377,0.4);
#37703=CYLINDRICAL_SURFACE('',#43379,0.4);
#37704=CYLINDRICAL_SURFACE('',#43380,0.4);
#37705=CYLINDRICAL_SURFACE('',#43382,0.4);
#37706=CYLINDRICAL_SURFACE('',#43383,0.4);
#37707=CYLINDRICAL_SURFACE('',#43388,0.4);
#37708=CYLINDRICAL_SURFACE('',#43389,0.4);
#37709=CYLINDRICAL_SURFACE('',#43403,0.4);
#37710=CYLINDRICAL_SURFACE('',#43404,0.4);
#37711=CYLINDRICAL_SURFACE('',#43406,0.4);
#37712=CYLINDRICAL_SURFACE('',#43408,0.4);
#37713=CYLINDRICAL_SURFACE('',#43410,0.4);
#37714=CYLINDRICAL_SURFACE('',#43412,0.4);
#37715=CYLINDRICAL_SURFACE('',#43416,0.4);
#37716=CYLINDRICAL_SURFACE('',#43421,0.4);
#37717=CYLINDRICAL_SURFACE('',#43435,0.4);
#37718=CYLINDRICAL_SURFACE('',#43436,0.4);
#37719=CYLINDRICAL_SURFACE('',#43438,0.4);
#37720=CYLINDRICAL_SURFACE('',#43440,0.4);
#37721=CYLINDRICAL_SURFACE('',#43442,0.4);
#37722=CYLINDRICAL_SURFACE('',#43444,0.4);
#37723=CYLINDRICAL_SURFACE('',#43448,0.4);
#37724=CYLINDRICAL_SURFACE('',#43453,0.4);
#37725=CYLINDRICAL_SURFACE('',#43467,0.4);
#37726=CYLINDRICAL_SURFACE('',#43468,0.4);
#37727=CYLINDRICAL_SURFACE('',#43470,0.4);
#37728=CYLINDRICAL_SURFACE('',#43472,0.4);
#37729=CYLINDRICAL_SURFACE('',#43474,0.4);
#37730=CYLINDRICAL_SURFACE('',#43476,0.4);
#37731=CYLINDRICAL_SURFACE('',#43480,0.4);
#37732=CYLINDRICAL_SURFACE('',#43485,0.4);
#37733=CYLINDRICAL_SURFACE('',#43499,0.4);
#37734=CYLINDRICAL_SURFACE('',#43500,0.4);
#37735=CYLINDRICAL_SURFACE('',#43502,0.4);
#37736=CYLINDRICAL_SURFACE('',#43504,0.4);
#37737=CYLINDRICAL_SURFACE('',#43506,0.4);
#37738=CYLINDRICAL_SURFACE('',#43508,0.4);
#37739=CYLINDRICAL_SURFACE('',#43512,0.4);
#37740=CYLINDRICAL_SURFACE('',#43517,0.4);
#37741=CYLINDRICAL_SURFACE('',#43531,0.4);
#37742=CYLINDRICAL_SURFACE('',#43532,0.4);
#37743=CYLINDRICAL_SURFACE('',#43534,0.4);
#37744=CYLINDRICAL_SURFACE('',#43631,12.);
#37745=CYLINDRICAL_SURFACE('',#43644,12.);
#37746=CYLINDRICAL_SURFACE('',#43654,0.4);
#37747=CYLINDRICAL_SURFACE('',#43656,0.4);
#37748=CYLINDRICAL_SURFACE('',#43659,12.);
#37749=CYLINDRICAL_SURFACE('',#43661,12.);
#37750=CYLINDRICAL_SURFACE('',#43662,12.);
#37751=CYLINDRICAL_SURFACE('',#43667,12.);
#37752=CYLINDRICAL_SURFACE('',#43669,12.);
#37753=CYLINDRICAL_SURFACE('',#43671,12.);
#37754=CYLINDRICAL_SURFACE('',#43672,12.);
#37755=CYLINDRICAL_SURFACE('',#43677,12.);
#37756=CYLINDRICAL_SURFACE('',#43679,12.);
#37757=CYLINDRICAL_SURFACE('',#43681,12.);
#37758=CYLINDRICAL_SURFACE('',#43686,12.);
#37759=CYLINDRICAL_SURFACE('',#43688,12.);
#37760=CYLINDRICAL_SURFACE('',#43690,12.);
#37761=CYLINDRICAL_SURFACE('',#43691,12.);
#37762=CYLINDRICAL_SURFACE('',#43696,12.);
#37763=CYLINDRICAL_SURFACE('',#43698,12.);
#37764=CYLINDRICAL_SURFACE('',#43700,12.);
#37765=CYLINDRICAL_SURFACE('',#43701,12.);
#37766=CYLINDRICAL_SURFACE('',#43707,12.);
#37767=CYLINDRICAL_SURFACE('',#43712,12.);
#37768=CYLINDRICAL_SURFACE('',#43714,12.);
#37769=CYLINDRICAL_SURFACE('',#43715,12.);
#39351=ADVANCED_FACE('',(#3548),#37698,.T.);
#39352=ADVANCED_FACE('',(#3549),#1329,.T.);
#39353=ADVANCED_FACE('',(#3550),#1330,.T.);
#39354=ADVANCED_FACE('',(#3551),#37699,.T.);
#39355=ADVANCED_FACE('',(#3552),#37700,.T.);
#39356=ADVANCED_FACE('',(#3553),#1331,.T.);
#39357=ADVANCED_FACE('',(#3554,#1052),#1332,.T.);
#39358=ADVANCED_FACE('',(#3555),#37701,.T.);
#39359=ADVANCED_FACE('',(#3556),#1333,.T.);
#39360=ADVANCED_FACE('',(#3557),#1334,.T.);
#39361=ADVANCED_FACE('',(#3558),#37702,.T.);
#39362=ADVANCED_FACE('',(#3559),#1335,.T.);
#39363=ADVANCED_FACE('',(#3560),#37703,.T.);
#39364=ADVANCED_FACE('',(#3561),#37704,.T.);
#39365=ADVANCED_FACE('',(#3562),#1336,.T.);
#39366=ADVANCED_FACE('',(#3563),#37705,.T.);
#39367=ADVANCED_FACE('',(#3564),#37706,.T.);
#39368=ADVANCED_FACE('',(#3565),#1337,.T.);
#39369=ADVANCED_FACE('',(#3566),#1338,.T.);
#39370=ADVANCED_FACE('',(#3567),#37707,.T.);
#39371=ADVANCED_FACE('',(#3568),#37708,.T.);
#39372=ADVANCED_FACE('',(#3569),#1339,.T.);
#39373=ADVANCED_FACE('',(#3570),#1340,.T.);
#39374=ADVANCED_FACE('',(#3571),#37709,.T.);
#39375=ADVANCED_FACE('',(#3572),#37710,.T.);
#39376=ADVANCED_FACE('',(#3573),#1341,.T.);
#39377=ADVANCED_FACE('',(#3574),#37711,.T.);
#39378=ADVANCED_FACE('',(#3575),#1342,.T.);
#39379=ADVANCED_FACE('',(#3576),#37712,.T.);
#39380=ADVANCED_FACE('',(#3577),#1343,.T.);
#39381=ADVANCED_FACE('',(#3578),#37713,.T.);
#39382=ADVANCED_FACE('',(#3579),#1344,.T.);
#39383=ADVANCED_FACE('',(#3580),#37714,.T.);
#39384=ADVANCED_FACE('',(#3581),#1345,.T.);
#39385=ADVANCED_FACE('',(#3582),#37715,.T.);
#39386=ADVANCED_FACE('',(#3583),#1346,.T.);
#39387=ADVANCED_FACE('',(#3584),#1347,.T.);
#39388=ADVANCED_FACE('',(#3585),#37716,.T.);
#39389=ADVANCED_FACE('',(#3586),#1348,.T.);
#39390=ADVANCED_FACE('',(#3587),#1349,.T.);
#39391=ADVANCED_FACE('',(#3588),#37717,.T.);
#39392=ADVANCED_FACE('',(#3589),#37718,.T.);
#39393=ADVANCED_FACE('',(#3590),#1350,.T.);
#39394=ADVANCED_FACE('',(#3591),#37719,.T.);
#39395=ADVANCED_FACE('',(#3592),#1351,.T.);
#39396=ADVANCED_FACE('',(#3593),#37720,.T.);
#39397=ADVANCED_FACE('',(#3594),#1352,.T.);
#39398=ADVANCED_FACE('',(#3595),#37721,.T.);
#39399=ADVANCED_FACE('',(#3596),#1353,.T.);
#39400=ADVANCED_FACE('',(#3597),#37722,.T.);
#39401=ADVANCED_FACE('',(#3598),#1354,.T.);
#39402=ADVANCED_FACE('',(#3599),#37723,.T.);
#39403=ADVANCED_FACE('',(#3600),#1355,.T.);
#39404=ADVANCED_FACE('',(#3601),#1356,.T.);
#39405=ADVANCED_FACE('',(#3602),#37724,.T.);
#39406=ADVANCED_FACE('',(#3603),#1357,.T.);
#39407=ADVANCED_FACE('',(#3604),#1358,.T.);
#39408=ADVANCED_FACE('',(#3605),#37725,.T.);
#39409=ADVANCED_FACE('',(#3606),#37726,.T.);
#39410=ADVANCED_FACE('',(#3607),#1359,.T.);
#39411=ADVANCED_FACE('',(#3608),#37727,.T.);
#39412=ADVANCED_FACE('',(#3609),#1360,.T.);
#39413=ADVANCED_FACE('',(#3610),#37728,.T.);
#39414=ADVANCED_FACE('',(#3611),#1361,.T.);
#39415=ADVANCED_FACE('',(#3612),#37729,.T.);
#39416=ADVANCED_FACE('',(#3613),#1362,.T.);
#39417=ADVANCED_FACE('',(#3614),#37730,.T.);
#39418=ADVANCED_FACE('',(#3615),#1363,.T.);
#39419=ADVANCED_FACE('',(#3616),#37731,.T.);
#39420=ADVANCED_FACE('',(#3617),#1364,.T.);
#39421=ADVANCED_FACE('',(#3618),#1365,.T.);
#39422=ADVANCED_FACE('',(#3619),#37732,.T.);
#39423=ADVANCED_FACE('',(#3620),#1366,.T.);
#39424=ADVANCED_FACE('',(#3621),#1367,.T.);
#39425=ADVANCED_FACE('',(#3622),#37733,.T.);
#39426=ADVANCED_FACE('',(#3623),#37734,.T.);
#39427=ADVANCED_FACE('',(#3624),#1368,.T.);
#39428=ADVANCED_FACE('',(#3625),#37735,.T.);
#39429=ADVANCED_FACE('',(#3626),#1369,.T.);
#39430=ADVANCED_FACE('',(#3627),#37736,.T.);
#39431=ADVANCED_FACE('',(#3628),#1370,.T.);
#39432=ADVANCED_FACE('',(#3629),#37737,.T.);
#39433=ADVANCED_FACE('',(#3630),#1371,.T.);
#39434=ADVANCED_FACE('',(#3631),#37738,.T.);
#39435=ADVANCED_FACE('',(#3632),#1372,.T.);
#39436=ADVANCED_FACE('',(#3633),#37739,.T.);
#39437=ADVANCED_FACE('',(#3634),#1373,.T.);
#39438=ADVANCED_FACE('',(#3635),#1374,.T.);
#39439=ADVANCED_FACE('',(#3636),#37740,.T.);
#39440=ADVANCED_FACE('',(#3637),#1375,.T.);
#39441=ADVANCED_FACE('',(#3638),#1376,.T.);
#39442=ADVANCED_FACE('',(#3639),#37741,.T.);
#39443=ADVANCED_FACE('',(#3640),#37742,.T.);
#39444=ADVANCED_FACE('',(#3641),#1377,.T.);
#39445=ADVANCED_FACE('',(#3642),#37743,.T.);
#39446=ADVANCED_FACE('',(#3643),#1378,.T.);
#39447=ADVANCED_FACE('',(#3644),#2106,.F.);
#39448=ADVANCED_FACE('',(#3645),#533,.T.);
#39449=ADVANCED_FACE('',(#3646),#534,.T.);
#39450=ADVANCED_FACE('',(#3647),#973,.T.);
#39451=ADVANCED_FACE('',(#3648),#2107,.F.);
#39452=ADVANCED_FACE('',(#3649),#974,.F.);
#39453=ADVANCED_FACE('',(#3650),#2108,.F.);
#39454=ADVANCED_FACE('',(#3651),#535,.T.);
#39455=ADVANCED_FACE('',(#3652),#536,.T.);
#39456=ADVANCED_FACE('',(#3653),#2109,.F.);
#39457=ADVANCED_FACE('',(#3654),#975,.T.);
#39458=ADVANCED_FACE('',(#3655),#537,.T.);
#39459=ADVANCED_FACE('',(#3656),#538,.T.);
#39460=ADVANCED_FACE('',(#3657),#976,.T.);
#39461=ADVANCED_FACE('',(#3658),#2110,.F.);
#39462=ADVANCED_FACE('',(#3659),#539,.T.);
#39463=ADVANCED_FACE('',(#3660),#2111,.F.);
#39464=ADVANCED_FACE('',(#3661),#977,.T.);
#39465=ADVANCED_FACE('',(#3662),#2112,.F.);
#39466=ADVANCED_FACE('',(#3663),#978,.F.);
#39467=ADVANCED_FACE('',(#3664),#2113,.F.);
#39468=ADVANCED_FACE('',(#3665),#540,.T.);
#39469=ADVANCED_FACE('',(#3666),#979,.T.);
#39470=ADVANCED_FACE('',(#3667),#541,.T.);
#39471=ADVANCED_FACE('',(#3668),#542,.T.);
#39472=ADVANCED_FACE('',(#3669),#980,.T.);
#39473=ADVANCED_FACE('',(#3670),#2114,.F.);
#39474=ADVANCED_FACE('',(#3671),#981,.F.);
#39475=ADVANCED_FACE('',(#3672),#2115,.F.);
#39476=ADVANCED_FACE('',(#3673),#2116,.F.);
#39477=ADVANCED_FACE('',(#3674),#543,.T.);
#39478=ADVANCED_FACE('',(#3675),#544,.T.);
#39479=ADVANCED_FACE('',(#3676),#2117,.F.);
#39480=ADVANCED_FACE('',(#3677),#982,.T.);
#39481=ADVANCED_FACE('',(#3678),#545,.T.);
#39482=ADVANCED_FACE('',(#3679),#983,.T.);
#39483=ADVANCED_FACE('',(#3680),#984,.T.);
#39484=ADVANCED_FACE('',(#3681),#546,.T.);
#39485=ADVANCED_FACE('',(#3682),#2118,.F.);
#39486=ADVANCED_FACE('',(#3683),#985,.F.);
#39487=ADVANCED_FACE('',(#3684),#547,.T.);
#39488=ADVANCED_FACE('',(#3685),#2119,.F.);
#39489=ADVANCED_FACE('',(#3686),#548,.T.);
#39490=ADVANCED_FACE('',(#3687),#986,.T.);
#39491=ADVANCED_FACE('',(#3688),#549,.T.);
#39492=ADVANCED_FACE('',(#3689),#2120,.F.);
#39493=ADVANCED_FACE('',(#3690),#2121,.F.);
#39494=ADVANCED_FACE('',(#3691),#2122,.F.);
#39495=ADVANCED_FACE('',(#3692),#2123,.F.);
#39496=ADVANCED_FACE('',(#3693),#550,.T.);
#39497=ADVANCED_FACE('',(#3694),#37744,.F.);
#39498=ADVANCED_FACE('',(#3695),#551,.T.);
#39499=ADVANCED_FACE('',(#3696),#2124,.F.);
#39500=ADVANCED_FACE('',(#3697),#987,.F.);
#39501=ADVANCED_FACE('',(#3698),#2125,.F.);
#39502=ADVANCED_FACE('',(#3699),#552,.T.);
#39503=ADVANCED_FACE('',(#3700),#553,.T.);
#39504=ADVANCED_FACE('',(#3701),#2126,.F.);
#39505=ADVANCED_FACE('',(#3702),#2127,.F.);
#39506=ADVANCED_FACE('',(#3703),#2128,.F.);
#39507=ADVANCED_FACE('',(#3704),#554,.T.);
#39508=ADVANCED_FACE('',(#3705),#37745,.F.);
#39509=ADVANCED_FACE('',(#3706),#2129,.F.);
#39510=ADVANCED_FACE('',(#3707),#988,.T.);
#39511=ADVANCED_FACE('',(#3708),#2130,.F.);
#39512=ADVANCED_FACE('',(#3709),#989,.F.);
#39513=ADVANCED_FACE('',(#3710),#555,.T.);
#39514=ADVANCED_FACE('',(#3711),#2131,.F.);
#39515=ADVANCED_FACE('',(#3712),#990,.T.);
#39516=ADVANCED_FACE('',(#3713),#2132,.F.);
#39517=ADVANCED_FACE('',(#3714),#556,.T.);
#39518=ADVANCED_FACE('',(#3715),#37746,.T.);
#39519=ADVANCED_FACE('',(#3716),#1379,.T.);
#39520=ADVANCED_FACE('',(#3717),#37747,.T.);
#39521=ADVANCED_FACE('',(#3718),#1380,.T.);
#39522=ADVANCED_FACE('',(#3719),#1381,.T.);
#39523=ADVANCED_FACE('',(#3720),#37748,.F.);
#39524=ADVANCED_FACE('',(#3721),#1382,.T.);
#39525=ADVANCED_FACE('',(#3722),#37749,.F.);
#39526=ADVANCED_FACE('',(#3723),#37750,.F.);
#39527=ADVANCED_FACE('',(#3724),#1383,.T.);
#39528=ADVANCED_FACE('',(#3725),#1384,.T.);
#39529=ADVANCED_FACE('',(#3726),#1385,.T.);
#39530=ADVANCED_FACE('',(#3727),#1386,.T.);
#39531=ADVANCED_FACE('',(#3728),#37751,.F.);
#39532=ADVANCED_FACE('',(#3729),#1387,.T.);
#39533=ADVANCED_FACE('',(#3730),#37752,.F.);
#39534=ADVANCED_FACE('',(#3731),#1388,.T.);
#39535=ADVANCED_FACE('',(#3732),#37753,.F.);
#39536=ADVANCED_FACE('',(#3733),#37754,.F.);
#39537=ADVANCED_FACE('',(#3734),#1389,.T.);
#39538=ADVANCED_FACE('',(#3735),#1390,.T.);
#39539=ADVANCED_FACE('',(#3736),#1391,.T.);
#39540=ADVANCED_FACE('',(#3737),#1392,.T.);
#39541=ADVANCED_FACE('',(#3738),#37755,.F.);
#39542=ADVANCED_FACE('',(#3739),#1393,.T.);
#39543=ADVANCED_FACE('',(#3740),#37756,.F.);
#39544=ADVANCED_FACE('',(#3741),#1394,.T.);
#39545=ADVANCED_FACE('',(#3742),#37757,.F.);
#39546=ADVANCED_FACE('',(#3743),#1395,.T.);
#39547=ADVANCED_FACE('',(#3744),#1396,.T.);
#39548=ADVANCED_FACE('',(#3745),#1397,.T.);
#39549=ADVANCED_FACE('',(#3746),#1398,.T.);
#39550=ADVANCED_FACE('',(#3747),#37758,.F.);
#39551=ADVANCED_FACE('',(#3748),#1399,.T.);
#39552=ADVANCED_FACE('',(#3749),#37759,.F.);
#39553=ADVANCED_FACE('',(#3750),#1400,.T.);
#39554=ADVANCED_FACE('',(#3751),#37760,.F.);
#39555=ADVANCED_FACE('',(#3752),#37761,.F.);
#39556=ADVANCED_FACE('',(#3753),#1401,.T.);
#39557=ADVANCED_FACE('',(#3754),#1402,.T.);
#39558=ADVANCED_FACE('',(#3755),#1403,.T.);
#39559=ADVANCED_FACE('',(#3756),#1404,.T.);
#39560=ADVANCED_FACE('',(#3757),#37762,.F.);
#39561=ADVANCED_FACE('',(#3758),#1405,.T.);
#39562=ADVANCED_FACE('',(#3759),#37763,.F.);
#39563=ADVANCED_FACE('',(#3760),#1406,.T.);
#39564=ADVANCED_FACE('',(#3761),#37764,.F.);
#39565=ADVANCED_FACE('',(#3762),#37765,.F.);
#39566=ADVANCED_FACE('',(#3763),#1407,.T.);
#39567=ADVANCED_FACE('',(#3764),#1408,.T.);
#39568=ADVANCED_FACE('',(#3765),#1409,.T.);
#39569=ADVANCED_FACE('',(#3766),#1410,.T.);
#39570=ADVANCED_FACE('',(#3767),#1411,.T.);
#39571=ADVANCED_FACE('',(#3768),#37766,.F.);
#39572=ADVANCED_FACE('',(#3769),#1412,.T.);
#39573=ADVANCED_FACE('',(#3770),#1413,.T.);
#39574=ADVANCED_FACE('',(#3771),#1414,.T.);
#39575=ADVANCED_FACE('',(#3772),#1415,.T.);
#39576=ADVANCED_FACE('',(#3773),#37767,.F.);
#39577=ADVANCED_FACE('',(#3774),#1416,.T.);
#39578=ADVANCED_FACE('',(#3775),#37768,.F.);
#39579=ADVANCED_FACE('',(#3776),#37769,.F.);
#39580=ADVANCED_FACE('',(#3777),#1417,.T.);
#39581=ADVANCED_FACE('',(#3778),#1418,.T.);
#39582=ADVANCED_FACE('',(#3779),#1419,.T.);
#40348=CLOSED_SHELL('',(#39351,#39352,#39353,#39354,#39355,#39356,#39357,
#39358,#39359,#39360,#39361,#39362,#39363,#39364,#39365,#39366,#39367,#39368,
#39369,#39370,#39371,#39372,#39373,#39374,#39375,#39376,#39377,#39378,#39379,
#39380,#39381,#39382,#39383,#39384,#39385,#39386,#39387,#39388,#39389,#39390,
#39391,#39392,#39393,#39394,#39395,#39396,#39397,#39398,#39399,#39400,#39401,
#39402,#39403,#39404,#39405,#39406,#39407,#39408,#39409,#39410,#39411,#39412,
#39413,#39414,#39415,#39416,#39417,#39418,#39419,#39420,#39421,#39422,#39423,
#39424,#39425,#39426,#39427,#39428,#39429,#39430,#39431,#39432,#39433,#39434,
#39435,#39436,#39437,#39438,#39439,#39440,#39441,#39442,#39443,#39444,#39445,
#39446,#39447,#39448,#39449,#39450,#39451,#39452,#39453,#39454,#39455,#39456,
#39457,#39458,#39459,#39460,#39461,#39462,#39463,#39464,#39465,#39466,#39467,
#39468,#39469,#39470,#39471,#39472,#39473,#39474,#39475,#39476,#39477,#39478,
#39479,#39480,#39481,#39482,#39483,#39484,#39485,#39486,#39487,#39488,#39489,
#39490,#39491,#39492,#39493,#39494,#39495,#39496,#39497,#39498,#39499,#39500,
#39501,#39502,#39503,#39504,#39505,#39506,#39507,#39508,#39509,#39510,#39511,
#39512,#39513,#39514,#39515,#39516,#39517,#39518,#39519,#39520,#39521,#39522,
#39523,#39524,#39525,#39526,#39527,#39528,#39529,#39530,#39531,#39532,#39533,
#39534,#39535,#39536,#39537,#39538,#39539,#39540,#39541,#39542,#39543,#39544,
#39545,#39546,#39547,#39548,#39549,#39550,#39551,#39552,#39553,#39554,#39555,
#39556,#39557,#39558,#39559,#39560,#39561,#39562,#39563,#39564,#39565,#39566,
#39567,#39568,#39569,#39570,#39571,#39572,#39573,#39574,#39575,#39576,#39577,
#39578,#39579,#39580,#39581,#39582));
#43275=AXIS2_PLACEMENT_3D('',#78381,#51887,#51888);
#43276=AXIS2_PLACEMENT_3D('',#78382,#51889,#51890);
#43277=AXIS2_PLACEMENT_3D('',#78385,#51891,#51892);
#43278=AXIS2_PLACEMENT_3D('',#78389,#51894,#51895);
#43279=AXIS2_PLACEMENT_3D('',#78391,#51897,#51898);
#43280=AXIS2_PLACEMENT_3D('',#78395,#51900,#51901);
#43281=AXIS2_PLACEMENT_3D('',#78401,#51905,#51906);
#43282=AXIS2_PLACEMENT_3D('',#78405,#51909,#51910);
#43283=AXIS2_PLACEMENT_3D('',#78407,#51911,#51912);
#43284=AXIS2_PLACEMENT_3D('',#78409,#51914,#51915);
#43285=AXIS2_PLACEMENT_3D('',#78412,#51916,#51917);
#43286=AXIS2_PLACEMENT_3D('',#78416,#51919,#51920);
#43287=AXIS2_PLACEMENT_3D('',#78418,#51922,#51923);
#43288=AXIS2_PLACEMENT_3D('',#78424,#51927,#51928);
#43289=AXIS2_PLACEMENT_3D('',#78427,#51929,#51930);
#43290=AXIS2_PLACEMENT_3D('',#78436,#51931,#51932);
#43291=AXIS2_PLACEMENT_3D('',#78445,#51933,#51934);
#43292=AXIS2_PLACEMENT_3D('',#78454,#51935,#51936);
#43293=AXIS2_PLACEMENT_3D('',#78463,#51937,#51938);
#43294=AXIS2_PLACEMENT_3D('',#78472,#51939,#51940);
#43295=AXIS2_PLACEMENT_3D('',#78481,#51942,#51943);
#43296=AXIS2_PLACEMENT_3D('',#78485,#51945,#51946);
#43297=AXIS2_PLACEMENT_3D('',#78489,#51948,#51949);
#43298=AXIS2_PLACEMENT_3D('',#78493,#51951,#51952);
#43299=AXIS2_PLACEMENT_3D('',#78497,#51954,#51955);
#43300=AXIS2_PLACEMENT_3D('',#78501,#51957,#51958);
#43301=AXIS2_PLACEMENT_3D('',#78505,#51960,#51961);
#43302=AXIS2_PLACEMENT_3D('',#78509,#51963,#51964);
#43303=AXIS2_PLACEMENT_3D('',#78513,#51966,#51967);
#43304=AXIS2_PLACEMENT_3D('',#78517,#51969,#51970);
#43305=AXIS2_PLACEMENT_3D('',#78521,#51972,#51973);
#43306=AXIS2_PLACEMENT_3D('',#78525,#51975,#51976);
#43307=AXIS2_PLACEMENT_3D('',#78529,#51978,#51979);
#43308=AXIS2_PLACEMENT_3D('',#78533,#51981,#51982);
#43309=AXIS2_PLACEMENT_3D('',#78537,#51984,#51985);
#43310=AXIS2_PLACEMENT_3D('',#78541,#51987,#51988);
#43311=AXIS2_PLACEMENT_3D('',#78545,#51990,#51991);
#43312=AXIS2_PLACEMENT_3D('',#78549,#51993,#51994);
#43313=AXIS2_PLACEMENT_3D('',#78553,#51996,#51997);
#43314=AXIS2_PLACEMENT_3D('',#78557,#51999,#52000);
#43315=AXIS2_PLACEMENT_3D('',#78561,#52002,#52003);
#43316=AXIS2_PLACEMENT_3D('',#78565,#52005,#52006);
#43317=AXIS2_PLACEMENT_3D('',#78569,#52008,#52009);
#43318=AXIS2_PLACEMENT_3D('',#78573,#52011,#52012);
#43319=AXIS2_PLACEMENT_3D('',#78577,#52014,#52015);
#43320=AXIS2_PLACEMENT_3D('',#78581,#52017,#52018);
#43321=AXIS2_PLACEMENT_3D('',#78585,#52020,#52021);
#43322=AXIS2_PLACEMENT_3D('',#78589,#52023,#52024);
#43323=AXIS2_PLACEMENT_3D('',#78593,#52026,#52027);
#43324=AXIS2_PLACEMENT_3D('',#78597,#52029,#52030);
#43325=AXIS2_PLACEMENT_3D('',#78601,#52032,#52033);
#43326=AXIS2_PLACEMENT_3D('',#78605,#52035,#52036);
#43327=AXIS2_PLACEMENT_3D('',#78609,#52038,#52039);
#43328=AXIS2_PLACEMENT_3D('',#78613,#52041,#52042);
#43329=AXIS2_PLACEMENT_3D('',#78617,#52044,#52045);
#43330=AXIS2_PLACEMENT_3D('',#78621,#52047,#52048);
#43331=AXIS2_PLACEMENT_3D('',#78625,#52050,#52051);
#43332=AXIS2_PLACEMENT_3D('',#78629,#52053,#52054);
#43333=AXIS2_PLACEMENT_3D('',#78633,#52056,#52057);
#43334=AXIS2_PLACEMENT_3D('',#78637,#52059,#52060);
#43335=AXIS2_PLACEMENT_3D('',#78641,#52062,#52063);
#43336=AXIS2_PLACEMENT_3D('',#78645,#52065,#52066);
#43337=AXIS2_PLACEMENT_3D('',#78649,#52068,#52069);
#43338=AXIS2_PLACEMENT_3D('',#78653,#52071,#52072);
#43339=AXIS2_PLACEMENT_3D('',#78657,#52074,#52075);
#43340=AXIS2_PLACEMENT_3D('',#78661,#52077,#52078);
#43341=AXIS2_PLACEMENT_3D('',#78665,#52080,#52081);
#43342=AXIS2_PLACEMENT_3D('',#78669,#52083,#52084);
#43343=AXIS2_PLACEMENT_3D('',#78673,#52086,#52087);
#43344=AXIS2_PLACEMENT_3D('',#78677,#52089,#52090);
#43345=AXIS2_PLACEMENT_3D('',#78681,#52092,#52093);
#43346=AXIS2_PLACEMENT_3D('',#78685,#52095,#52096);
#43347=AXIS2_PLACEMENT_3D('',#78689,#52098,#52099);
#43348=AXIS2_PLACEMENT_3D('',#78693,#52101,#52102);
#43349=AXIS2_PLACEMENT_3D('',#78697,#52104,#52105);
#43350=AXIS2_PLACEMENT_3D('',#78701,#52107,#52108);
#43351=AXIS2_PLACEMENT_3D('',#78705,#52110,#52111);
#43352=AXIS2_PLACEMENT_3D('',#78709,#52113,#52114);
#43353=AXIS2_PLACEMENT_3D('',#78713,#52116,#52117);
#43354=AXIS2_PLACEMENT_3D('',#78717,#52119,#52120);
#43355=AXIS2_PLACEMENT_3D('',#78721,#52122,#52123);
#43356=AXIS2_PLACEMENT_3D('',#78725,#52125,#52126);
#43357=AXIS2_PLACEMENT_3D('',#78729,#52128,#52129);
#43358=AXIS2_PLACEMENT_3D('',#78733,#52131,#52132);
#43359=AXIS2_PLACEMENT_3D('',#78737,#52134,#52135);
#43360=AXIS2_PLACEMENT_3D('',#78741,#52137,#52138);
#43361=AXIS2_PLACEMENT_3D('',#78745,#52140,#52141);
#43362=AXIS2_PLACEMENT_3D('',#78749,#52143,#52144);
#43363=AXIS2_PLACEMENT_3D('',#78753,#52146,#52147);
#43364=AXIS2_PLACEMENT_3D('',#78755,#52149,#52150);
#43365=AXIS2_PLACEMENT_3D('',#78758,#52151,#52152);
#43366=AXIS2_PLACEMENT_3D('',#78761,#52155,#52156);
#43367=AXIS2_PLACEMENT_3D('',#78765,#52159,#52160);
#43368=AXIS2_PLACEMENT_3D('',#78767,#52161,#52162);
#43369=AXIS2_PLACEMENT_3D('',#78776,#52163,#52164);
#43370=AXIS2_PLACEMENT_3D('',#78785,#52165,#52166);
#43371=AXIS2_PLACEMENT_3D('',#78789,#52168,#52169);
#43372=AXIS2_PLACEMENT_3D('',#78793,#52171,#52172);
#43373=AXIS2_PLACEMENT_3D('',#78797,#52174,#52175);
#43374=AXIS2_PLACEMENT_3D('',#78801,#52177,#52178);
#43375=AXIS2_PLACEMENT_3D('',#78805,#52180,#52181);
#43376=AXIS2_PLACEMENT_3D('',#78808,#52183,#52184);
#43377=AXIS2_PLACEMENT_3D('',#78810,#52186,#52187);
#43378=AXIS2_PLACEMENT_3D('',#78813,#52190,#52191);
#43379=AXIS2_PLACEMENT_3D('',#78815,#52193,#52194);
#43380=AXIS2_PLACEMENT_3D('',#78817,#52196,#52197);
#43381=AXIS2_PLACEMENT_3D('',#78820,#52200,#52201);
#43382=AXIS2_PLACEMENT_3D('',#78822,#52203,#52204);
#43383=AXIS2_PLACEMENT_3D('',#78824,#52206,#52207);
#43384=AXIS2_PLACEMENT_3D('',#78827,#52208,#52209);
#43385=AXIS2_PLACEMENT_3D('',#78830,#52212,#52213);
#43386=AXIS2_PLACEMENT_3D('',#78834,#52215,#52216);
#43387=AXIS2_PLACEMENT_3D('',#78840,#52220,#52221);
#43388=AXIS2_PLACEMENT_3D('',#78842,#52223,#52224);
#43389=AXIS2_PLACEMENT_3D('',#78844,#52226,#52227);
#43390=AXIS2_PLACEMENT_3D('',#78847,#52228,#52229);
#43391=AXIS2_PLACEMENT_3D('',#78850,#52232,#52233);
#43392=AXIS2_PLACEMENT_3D('',#78854,#52235,#52236);
#43393=AXIS2_PLACEMENT_3D('',#78858,#52238,#52239);
#43394=AXIS2_PLACEMENT_3D('',#78867,#52240,#52241);
#43395=AXIS2_PLACEMENT_3D('',#78876,#52242,#52243);
#43396=AXIS2_PLACEMENT_3D('',#78880,#52245,#52246);
#43397=AXIS2_PLACEMENT_3D('',#78884,#52248,#52249);
#43398=AXIS2_PLACEMENT_3D('',#78888,#52251,#52252);
#43399=AXIS2_PLACEMENT_3D('',#78892,#52254,#52255);
#43400=AXIS2_PLACEMENT_3D('',#78896,#52257,#52258);
#43401=AXIS2_PLACEMENT_3D('',#78900,#52260,#52261);
#43402=AXIS2_PLACEMENT_3D('',#78902,#52263,#52264);
#43403=AXIS2_PLACEMENT_3D('',#78904,#52266,#52267);
#43404=AXIS2_PLACEMENT_3D('',#78906,#52269,#52270);
#43405=AXIS2_PLACEMENT_3D('',#78909,#52273,#52274);
#43406=AXIS2_PLACEMENT_3D('',#78911,#52276,#52277);
#43407=AXIS2_PLACEMENT_3D('',#78914,#52280,#52281);
#43408=AXIS2_PLACEMENT_3D('',#78916,#52283,#52284);
#43409=AXIS2_PLACEMENT_3D('',#78919,#52287,#52288);
#43410=AXIS2_PLACEMENT_3D('',#78921,#52290,#52291);
#43411=AXIS2_PLACEMENT_3D('',#78924,#52294,#52295);
#43412=AXIS2_PLACEMENT_3D('',#78926,#52297,#52298);
#43413=AXIS2_PLACEMENT_3D('',#78929,#52299,#52300);
#43414=AXIS2_PLACEMENT_3D('',#78932,#52303,#52304);
#43415=AXIS2_PLACEMENT_3D('',#78950,#52306,#52307);
#43416=AXIS2_PLACEMENT_3D('',#78954,#52310,#52311);
#43417=AXIS2_PLACEMENT_3D('',#78957,#52312,#52313);
#43418=AXIS2_PLACEMENT_3D('',#78960,#52316,#52317);
#43419=AXIS2_PLACEMENT_3D('',#78966,#52320,#52321);
#43420=AXIS2_PLACEMENT_3D('',#78982,#52323,#52324);
#43421=AXIS2_PLACEMENT_3D('',#78985,#52327,#52328);
#43422=AXIS2_PLACEMENT_3D('',#78988,#52329,#52330);
#43423=AXIS2_PLACEMENT_3D('',#78991,#52333,#52334);
#43424=AXIS2_PLACEMENT_3D('',#78995,#52336,#52337);
#43425=AXIS2_PLACEMENT_3D('',#78999,#52339,#52340);
#43426=AXIS2_PLACEMENT_3D('',#79008,#52341,#52342);
#43427=AXIS2_PLACEMENT_3D('',#79017,#52343,#52344);
#43428=AXIS2_PLACEMENT_3D('',#79021,#52346,#52347);
#43429=AXIS2_PLACEMENT_3D('',#79025,#52349,#52350);
#43430=AXIS2_PLACEMENT_3D('',#79029,#52352,#52353);
#43431=AXIS2_PLACEMENT_3D('',#79033,#52355,#52356);
#43432=AXIS2_PLACEMENT_3D('',#79037,#52358,#52359);
#43433=AXIS2_PLACEMENT_3D('',#79041,#52361,#52362);
#43434=AXIS2_PLACEMENT_3D('',#79043,#52364,#52365);
#43435=AXIS2_PLACEMENT_3D('',#79045,#52367,#52368);
#43436=AXIS2_PLACEMENT_3D('',#79047,#52370,#52371);
#43437=AXIS2_PLACEMENT_3D('',#79050,#52374,#52375);
#43438=AXIS2_PLACEMENT_3D('',#79052,#52377,#52378);
#43439=AXIS2_PLACEMENT_3D('',#79055,#52381,#52382);
#43440=AXIS2_PLACEMENT_3D('',#79057,#52384,#52385);
#43441=AXIS2_PLACEMENT_3D('',#79060,#52388,#52389);
#43442=AXIS2_PLACEMENT_3D('',#79062,#52391,#52392);
#43443=AXIS2_PLACEMENT_3D('',#79065,#52395,#52396);
#43444=AXIS2_PLACEMENT_3D('',#79067,#52398,#52399);
#43445=AXIS2_PLACEMENT_3D('',#79070,#52400,#52401);
#43446=AXIS2_PLACEMENT_3D('',#79073,#52404,#52405);
#43447=AXIS2_PLACEMENT_3D('',#79091,#52407,#52408);
#43448=AXIS2_PLACEMENT_3D('',#79095,#52411,#52412);
#43449=AXIS2_PLACEMENT_3D('',#79098,#52413,#52414);
#43450=AXIS2_PLACEMENT_3D('',#79101,#52417,#52418);
#43451=AXIS2_PLACEMENT_3D('',#79107,#52421,#52422);
#43452=AXIS2_PLACEMENT_3D('',#79123,#52424,#52425);
#43453=AXIS2_PLACEMENT_3D('',#79126,#52428,#52429);
#43454=AXIS2_PLACEMENT_3D('',#79129,#52430,#52431);
#43455=AXIS2_PLACEMENT_3D('',#79132,#52434,#52435);
#43456=AXIS2_PLACEMENT_3D('',#79136,#52437,#52438);
#43457=AXIS2_PLACEMENT_3D('',#79140,#52440,#52441);
#43458=AXIS2_PLACEMENT_3D('',#79149,#52442,#52443);
#43459=AXIS2_PLACEMENT_3D('',#79158,#52444,#52445);
#43460=AXIS2_PLACEMENT_3D('',#79162,#52447,#52448);
#43461=AXIS2_PLACEMENT_3D('',#79166,#52450,#52451);
#43462=AXIS2_PLACEMENT_3D('',#79170,#52453,#52454);
#43463=AXIS2_PLACEMENT_3D('',#79174,#52456,#52457);
#43464=AXIS2_PLACEMENT_3D('',#79178,#52459,#52460);
#43465=AXIS2_PLACEMENT_3D('',#79182,#52462,#52463);
#43466=AXIS2_PLACEMENT_3D('',#79184,#52465,#52466);
#43467=AXIS2_PLACEMENT_3D('',#79186,#52468,#52469);
#43468=AXIS2_PLACEMENT_3D('',#79188,#52471,#52472);
#43469=AXIS2_PLACEMENT_3D('',#79191,#52475,#52476);
#43470=AXIS2_PLACEMENT_3D('',#79193,#52478,#52479);
#43471=AXIS2_PLACEMENT_3D('',#79196,#52482,#52483);
#43472=AXIS2_PLACEMENT_3D('',#79198,#52485,#52486);
#43473=AXIS2_PLACEMENT_3D('',#79201,#52489,#52490);
#43474=AXIS2_PLACEMENT_3D('',#79203,#52492,#52493);
#43475=AXIS2_PLACEMENT_3D('',#79206,#52496,#52497);
#43476=AXIS2_PLACEMENT_3D('',#79208,#52499,#52500);
#43477=AXIS2_PLACEMENT_3D('',#79211,#52501,#52502);
#43478=AXIS2_PLACEMENT_3D('',#79214,#52505,#52506);
#43479=AXIS2_PLACEMENT_3D('',#79232,#52508,#52509);
#43480=AXIS2_PLACEMENT_3D('',#79236,#52512,#52513);
#43481=AXIS2_PLACEMENT_3D('',#79239,#52514,#52515);
#43482=AXIS2_PLACEMENT_3D('',#79242,#52518,#52519);
#43483=AXIS2_PLACEMENT_3D('',#79248,#52522,#52523);
#43484=AXIS2_PLACEMENT_3D('',#79264,#52525,#52526);
#43485=AXIS2_PLACEMENT_3D('',#79267,#52529,#52530);
#43486=AXIS2_PLACEMENT_3D('',#79270,#52531,#52532);
#43487=AXIS2_PLACEMENT_3D('',#79273,#52535,#52536);
#43488=AXIS2_PLACEMENT_3D('',#79277,#52538,#52539);
#43489=AXIS2_PLACEMENT_3D('',#79281,#52541,#52542);
#43490=AXIS2_PLACEMENT_3D('',#79290,#52543,#52544);
#43491=AXIS2_PLACEMENT_3D('',#79299,#52545,#52546);
#43492=AXIS2_PLACEMENT_3D('',#79303,#52548,#52549);
#43493=AXIS2_PLACEMENT_3D('',#79307,#52551,#52552);
#43494=AXIS2_PLACEMENT_3D('',#79311,#52554,#52555);
#43495=AXIS2_PLACEMENT_3D('',#79315,#52557,#52558);
#43496=AXIS2_PLACEMENT_3D('',#79319,#52560,#52561);
#43497=AXIS2_PLACEMENT_3D('',#79323,#52563,#52564);
#43498=AXIS2_PLACEMENT_3D('',#79325,#52566,#52567);
#43499=AXIS2_PLACEMENT_3D('',#79327,#52569,#52570);
#43500=AXIS2_PLACEMENT_3D('',#79329,#52572,#52573);
#43501=AXIS2_PLACEMENT_3D('',#79332,#52576,#52577);
#43502=AXIS2_PLACEMENT_3D('',#79334,#52579,#52580);
#43503=AXIS2_PLACEMENT_3D('',#79337,#52583,#52584);
#43504=AXIS2_PLACEMENT_3D('',#79339,#52586,#52587);
#43505=AXIS2_PLACEMENT_3D('',#79342,#52590,#52591);
#43506=AXIS2_PLACEMENT_3D('',#79344,#52593,#52594);
#43507=AXIS2_PLACEMENT_3D('',#79347,#52597,#52598);
#43508=AXIS2_PLACEMENT_3D('',#79349,#52600,#52601);
#43509=AXIS2_PLACEMENT_3D('',#79352,#52602,#52603);
#43510=AXIS2_PLACEMENT_3D('',#79355,#52606,#52607);
#43511=AXIS2_PLACEMENT_3D('',#79373,#52609,#52610);
#43512=AXIS2_PLACEMENT_3D('',#79377,#52613,#52614);
#43513=AXIS2_PLACEMENT_3D('',#79380,#52615,#52616);
#43514=AXIS2_PLACEMENT_3D('',#79383,#52619,#52620);
#43515=AXIS2_PLACEMENT_3D('',#79389,#52623,#52624);
#43516=AXIS2_PLACEMENT_3D('',#79405,#52626,#52627);
#43517=AXIS2_PLACEMENT_3D('',#79408,#52630,#52631);
#43518=AXIS2_PLACEMENT_3D('',#79411,#52632,#52633);
#43519=AXIS2_PLACEMENT_3D('',#79414,#52636,#52637);
#43520=AXIS2_PLACEMENT_3D('',#79418,#52639,#52640);
#43521=AXIS2_PLACEMENT_3D('',#79422,#52642,#52643);
#43522=AXIS2_PLACEMENT_3D('',#79431,#52644,#52645);
#43523=AXIS2_PLACEMENT_3D('',#79440,#52646,#52647);
#43524=AXIS2_PLACEMENT_3D('',#79444,#52649,#52650);
#43525=AXIS2_PLACEMENT_3D('',#79448,#52652,#52653);
#43526=AXIS2_PLACEMENT_3D('',#79452,#52655,#52656);
#43527=AXIS2_PLACEMENT_3D('',#79456,#52658,#52659);
#43528=AXIS2_PLACEMENT_3D('',#79460,#52661,#52662);
#43529=AXIS2_PLACEMENT_3D('',#79464,#52664,#52665);
#43530=AXIS2_PLACEMENT_3D('',#79466,#52667,#52668);
#43531=AXIS2_PLACEMENT_3D('',#79468,#52670,#52671);
#43532=AXIS2_PLACEMENT_3D('',#79470,#52673,#52674);
#43533=AXIS2_PLACEMENT_3D('',#79473,#52677,#52678);
#43534=AXIS2_PLACEMENT_3D('',#79475,#52680,#52681);
#43535=AXIS2_PLACEMENT_3D('',#79478,#52684,#52685);
#43536=AXIS2_PLACEMENT_3D('',#79507,#52687,#52688);
#43537=AXIS2_PLACEMENT_3D('',#79515,#52689,#52690);
#43538=AXIS2_PLACEMENT_3D('',#79521,#52691,#52692);
#43539=AXIS2_PLACEMENT_3D('',#79522,#52693,#52694);
#43540=AXIS2_PLACEMENT_3D('',#79523,#52695,#52696);
#43541=AXIS2_PLACEMENT_3D('',#79524,#52697,#52698);
#43542=AXIS2_PLACEMENT_3D('',#79525,#52699,#52700);
#43543=AXIS2_PLACEMENT_3D('',#79526,#52701,#52702);
#43544=AXIS2_PLACEMENT_3D('',#79527,#52703,#52704);
#43545=AXIS2_PLACEMENT_3D('',#79529,#52705,#52706);
#43546=AXIS2_PLACEMENT_3D('',#79530,#52707,#52708);
#43547=AXIS2_PLACEMENT_3D('',#79607,#52709,#52710);
#43548=AXIS2_PLACEMENT_3D('',#79616,#52711,#52712);
#43549=AXIS2_PLACEMENT_3D('',#79625,#52713,#52714);
#43550=AXIS2_PLACEMENT_3D('',#79672,#52715,#52716);
#43551=AXIS2_PLACEMENT_3D('',#79680,#52717,#52718);
#43552=AXIS2_PLACEMENT_3D('',#79686,#52719,#52720);
#43553=AXIS2_PLACEMENT_3D('',#79687,#52721,#52722);
#43554=AXIS2_PLACEMENT_3D('',#79688,#52723,#52724);
#43555=AXIS2_PLACEMENT_3D('',#79689,#52725,#52726);
#43556=AXIS2_PLACEMENT_3D('',#79690,#52727,#52728);
#43557=AXIS2_PLACEMENT_3D('',#79691,#52729,#52730);
#43558=AXIS2_PLACEMENT_3D('',#79732,#52731,#52732);
#43559=AXIS2_PLACEMENT_3D('',#79734,#52733,#52734);
#43560=AXIS2_PLACEMENT_3D('',#79735,#52735,#52736);
#43561=AXIS2_PLACEMENT_3D('',#79736,#52737,#52738);
#43562=AXIS2_PLACEMENT_3D('',#79738,#52739,#52740);
#43563=AXIS2_PLACEMENT_3D('',#79744,#52741,#52742);
#43564=AXIS2_PLACEMENT_3D('',#79746,#52743,#52744);
#43565=AXIS2_PLACEMENT_3D('',#79747,#52745,#52746);
#43566=AXIS2_PLACEMENT_3D('',#79748,#52747,#52748);
#43567=AXIS2_PLACEMENT_3D('',#79750,#52749,#52750);
#43568=AXIS2_PLACEMENT_3D('',#79820,#52751,#52752);
#43569=AXIS2_PLACEMENT_3D('',#79831,#52753,#52754);
#43570=AXIS2_PLACEMENT_3D('',#79833,#52755,#52756);
#43571=AXIS2_PLACEMENT_3D('',#79834,#52757,#52758);
#43572=AXIS2_PLACEMENT_3D('',#79866,#52759,#52760);
#43573=AXIS2_PLACEMENT_3D('',#79873,#52761,#52762);
#43574=AXIS2_PLACEMENT_3D('',#79875,#52763,#52764);
#43575=AXIS2_PLACEMENT_3D('',#79877,#52765,#52766);
#43576=AXIS2_PLACEMENT_3D('',#79878,#52767,#52768);
#43577=AXIS2_PLACEMENT_3D('',#79911,#52769,#52770);
#43578=AXIS2_PLACEMENT_3D('',#79917,#52771,#52772);
#43579=AXIS2_PLACEMENT_3D('',#79976,#52773,#52774);
#43580=AXIS2_PLACEMENT_3D('',#79984,#52775,#52776);
#43581=AXIS2_PLACEMENT_3D('',#79990,#52777,#52778);
#43582=AXIS2_PLACEMENT_3D('',#79991,#52779,#52780);
#43583=AXIS2_PLACEMENT_3D('',#79992,#52781,#52782);
#43584=AXIS2_PLACEMENT_3D('',#79993,#52783,#52784);
#43585=AXIS2_PLACEMENT_3D('',#79994,#52785,#52786);
#43586=AXIS2_PLACEMENT_3D('',#79996,#52787,#52788);
#43587=AXIS2_PLACEMENT_3D('',#79998,#52789,#52790);
#43588=AXIS2_PLACEMENT_3D('',#79999,#52791,#52792);
#43589=AXIS2_PLACEMENT_3D('',#80000,#52793,#52794);
#43590=AXIS2_PLACEMENT_3D('',#80001,#52795,#52796);
#43591=AXIS2_PLACEMENT_3D('',#80002,#52797,#52798);
#43592=AXIS2_PLACEMENT_3D('',#80003,#52799,#52800);
#43593=AXIS2_PLACEMENT_3D('',#80004,#52801,#52802);
#43594=AXIS2_PLACEMENT_3D('',#80006,#52803,#52804);
#43595=AXIS2_PLACEMENT_3D('',#80007,#52805,#52806);
#43596=AXIS2_PLACEMENT_3D('',#80048,#52807,#52808);
#43597=AXIS2_PLACEMENT_3D('',#80104,#52809,#52810);
#43598=AXIS2_PLACEMENT_3D('',#80131,#52811,#52812);
#43599=AXIS2_PLACEMENT_3D('',#80138,#52813,#52814);
#43600=AXIS2_PLACEMENT_3D('',#80139,#52815,#52816);
#43601=AXIS2_PLACEMENT_3D('',#80140,#52817,#52818);
#43602=AXIS2_PLACEMENT_3D('',#80141,#52819,#52820);
#43603=AXIS2_PLACEMENT_3D('',#80142,#52821,#52822);
#43604=AXIS2_PLACEMENT_3D('',#80143,#52823,#52824);
#43605=AXIS2_PLACEMENT_3D('',#80178,#52825,#52826);
#43606=AXIS2_PLACEMENT_3D('',#80180,#52827,#52828);
#43607=AXIS2_PLACEMENT_3D('',#80191,#52829,#52830);
#43608=AXIS2_PLACEMENT_3D('',#80193,#52831,#52832);
#43609=AXIS2_PLACEMENT_3D('',#80222,#52833,#52834);
#43610=AXIS2_PLACEMENT_3D('',#80254,#52835,#52836);
#43611=AXIS2_PLACEMENT_3D('',#80255,#52837,#52838);
#43612=AXIS2_PLACEMENT_3D('',#80256,#52839,#52840);
#43613=AXIS2_PLACEMENT_3D('',#80258,#52841,#52842);
#43614=AXIS2_PLACEMENT_3D('',#80259,#52843,#52844);
#43615=AXIS2_PLACEMENT_3D('',#80296,#52845,#52846);
#43616=AXIS2_PLACEMENT_3D('',#80309,#52847,#52848);
#43617=AXIS2_PLACEMENT_3D('',#80310,#52849,#52850);
#43618=AXIS2_PLACEMENT_3D('',#80311,#52851,#52852);
#43619=AXIS2_PLACEMENT_3D('',#80346,#52853,#52854);
#43620=AXIS2_PLACEMENT_3D('',#80348,#52855,#52856);
#43621=AXIS2_PLACEMENT_3D('',#80350,#52857,#52858);
#43622=AXIS2_PLACEMENT_3D('',#80351,#52859,#52860);
#43623=AXIS2_PLACEMENT_3D('',#80352,#52861,#52862);
#43624=AXIS2_PLACEMENT_3D('',#80353,#52863,#52864);
#43625=AXIS2_PLACEMENT_3D('',#80354,#52865,#52866);
#43626=AXIS2_PLACEMENT_3D('',#80356,#52867,#52868);
#43627=AXIS2_PLACEMENT_3D('',#80357,#52869,#52870);
#43628=AXIS2_PLACEMENT_3D('',#80500,#52871,#52872);
#43629=AXIS2_PLACEMENT_3D('',#80501,#52873,#52874);
#43630=AXIS2_PLACEMENT_3D('',#80502,#52875,#52876);
#43631=AXIS2_PLACEMENT_3D('',#80503,#52877,#52878);
#43632=AXIS2_PLACEMENT_3D('',#80505,#52880,#52881);
#43633=AXIS2_PLACEMENT_3D('',#80507,#52882,#52883);
#43634=AXIS2_PLACEMENT_3D('',#80548,#52884,#52885);
#43635=AXIS2_PLACEMENT_3D('',#80589,#52886,#52887);
#43636=AXIS2_PLACEMENT_3D('',#80591,#52888,#52889);
#43637=AXIS2_PLACEMENT_3D('',#80592,#52890,#52891);
#43638=AXIS2_PLACEMENT_3D('',#80593,#52892,#52893);
#43639=AXIS2_PLACEMENT_3D('',#80600,#52894,#52895);
#43640=AXIS2_PLACEMENT_3D('',#80718,#52896,#52897);
#43641=AXIS2_PLACEMENT_3D('',#80724,#52898,#52899);
#43642=AXIS2_PLACEMENT_3D('',#80725,#52900,#52901);
#43643=AXIS2_PLACEMENT_3D('',#80726,#52902,#52903);
#43644=AXIS2_PLACEMENT_3D('',#80727,#52904,#52905);
#43645=AXIS2_PLACEMENT_3D('',#80785,#52908,#52909);
#43646=AXIS2_PLACEMENT_3D('',#80786,#52910,#52911);
#43647=AXIS2_PLACEMENT_3D('',#80835,#52912,#52913);
#43648=AXIS2_PLACEMENT_3D('',#80837,#52914,#52915);
#43649=AXIS2_PLACEMENT_3D('',#80845,#52916,#52917);
#43650=AXIS2_PLACEMENT_3D('',#80846,#52918,#52919);
#43651=AXIS2_PLACEMENT_3D('',#80913,#52920,#52921);
#43652=AXIS2_PLACEMENT_3D('',#80925,#52922,#52923);
#43653=AXIS2_PLACEMENT_3D('',#80967,#52924,#52925);
#43654=AXIS2_PLACEMENT_3D('',#80968,#52926,#52927);
#43655=AXIS2_PLACEMENT_3D('',#80971,#52930,#52931);
#43656=AXIS2_PLACEMENT_3D('',#80973,#52933,#52934);
#43657=AXIS2_PLACEMENT_3D('',#80975,#52936,#52937);
#43658=AXIS2_PLACEMENT_3D('',#80977,#52939,#52940);
#43659=AXIS2_PLACEMENT_3D('',#80979,#52942,#52943);
#43660=AXIS2_PLACEMENT_3D('',#80980,#52944,#52945);
#43661=AXIS2_PLACEMENT_3D('',#80981,#52946,#52947);
#43662=AXIS2_PLACEMENT_3D('',#80983,#52949,#52950);
#43663=AXIS2_PLACEMENT_3D('',#80985,#52952,#52953);
#43664=AXIS2_PLACEMENT_3D('',#80987,#52955,#52956);
#43665=AXIS2_PLACEMENT_3D('',#80988,#52957,#52958);
#43666=AXIS2_PLACEMENT_3D('',#80989,#52959,#52960);
#43667=AXIS2_PLACEMENT_3D('',#80990,#52961,#52962);
#43668=AXIS2_PLACEMENT_3D('',#80991,#52963,#52964);
#43669=AXIS2_PLACEMENT_3D('',#80992,#52965,#52966);
#43670=AXIS2_PLACEMENT_3D('',#80993,#52967,#52968);
#43671=AXIS2_PLACEMENT_3D('',#80994,#52969,#52970);
#43672=AXIS2_PLACEMENT_3D('',#80995,#52971,#52972);
#43673=AXIS2_PLACEMENT_3D('',#80997,#52974,#52975);
#43674=AXIS2_PLACEMENT_3D('',#80998,#52976,#52977);
#43675=AXIS2_PLACEMENT_3D('',#80999,#52978,#52979);
#43676=AXIS2_PLACEMENT_3D('',#81000,#52980,#52981);
#43677=AXIS2_PLACEMENT_3D('',#81001,#52982,#52983);
#43678=AXIS2_PLACEMENT_3D('',#81002,#52984,#52985);
#43679=AXIS2_PLACEMENT_3D('',#81003,#52986,#52987);
#43680=AXIS2_PLACEMENT_3D('',#81004,#52988,#52989);
#43681=AXIS2_PLACEMENT_3D('',#81005,#52990,#52991);
#43682=AXIS2_PLACEMENT_3D('',#81007,#52993,#52994);
#43683=AXIS2_PLACEMENT_3D('',#81009,#52996,#52997);
#43684=AXIS2_PLACEMENT_3D('',#81010,#52998,#52999);
#43685=AXIS2_PLACEMENT_3D('',#81011,#53000,#53001);
#43686=AXIS2_PLACEMENT_3D('',#81012,#53002,#53003);
#43687=AXIS2_PLACEMENT_3D('',#81013,#53004,#53005);
#43688=AXIS2_PLACEMENT_3D('',#81014,#53006,#53007);
#43689=AXIS2_PLACEMENT_3D('',#81015,#53008,#53009);
#43690=AXIS2_PLACEMENT_3D('',#81016,#53010,#53011);
#43691=AXIS2_PLACEMENT_3D('',#81017,#53012,#53013);
#43692=AXIS2_PLACEMENT_3D('',#81019,#53015,#53016);
#43693=AXIS2_PLACEMENT_3D('',#81021,#53018,#53019);
#43694=AXIS2_PLACEMENT_3D('',#81022,#53020,#53021);
#43695=AXIS2_PLACEMENT_3D('',#81023,#53022,#53023);
#43696=AXIS2_PLACEMENT_3D('',#81024,#53024,#53025);
#43697=AXIS2_PLACEMENT_3D('',#81025,#53026,#53027);
#43698=AXIS2_PLACEMENT_3D('',#81026,#53028,#53029);
#43699=AXIS2_PLACEMENT_3D('',#81027,#53030,#53031);
#43700=AXIS2_PLACEMENT_3D('',#81028,#53032,#53033);
#43701=AXIS2_PLACEMENT_3D('',#81029,#53034,#53035);
#43702=AXIS2_PLACEMENT_3D('',#81031,#53037,#53038);
#43703=AXIS2_PLACEMENT_3D('',#81032,#53039,#53040);
#43704=AXIS2_PLACEMENT_3D('',#81033,#53041,#53042);
#43705=AXIS2_PLACEMENT_3D('',#81036,#53045,#53046);
#43706=AXIS2_PLACEMENT_3D('',#81038,#53048,#53049);
#43707=AXIS2_PLACEMENT_3D('',#81039,#53050,#53051);
#43708=AXIS2_PLACEMENT_3D('',#81041,#53053,#53054);
#43709=AXIS2_PLACEMENT_3D('',#81043,#53056,#53057);
#43710=AXIS2_PLACEMENT_3D('',#81044,#53058,#53059);
#43711=AXIS2_PLACEMENT_3D('',#81046,#53061,#53062);
#43712=AXIS2_PLACEMENT_3D('',#81048,#53064,#53065);
#43713=AXIS2_PLACEMENT_3D('',#81049,#53066,#53067);
#43714=AXIS2_PLACEMENT_3D('',#81050,#53068,#53069);
#43715=AXIS2_PLACEMENT_3D('',#81051,#53070,#53071);
#43716=AXIS2_PLACEMENT_3D('',#81053,#53073,#53074);
#43717=AXIS2_PLACEMENT_3D('',#81055,#53076,#53077);
#43718=AXIS2_PLACEMENT_3D('',#81057,#53079,#53080);
#51887=DIRECTION('axis',(0.,0.,1.));
#51888=DIRECTION('refdir',(1.,0.,0.));
#51889=DIRECTION('center_axis',(1.,0.,0.));
#51890=DIRECTION('ref_axis',(0.,-0.707106781186548,0.707106781186547));
#51891=DIRECTION('center_axis',(-1.,0.,0.));
#51892=DIRECTION('ref_axis',(0.,-0.707106781186548,0.707106781186547));
#51893=DIRECTION('',(-1.,0.,0.));
#51894=DIRECTION('center_axis',(1.,0.,0.));
#51895=DIRECTION('ref_axis',(0.,-0.707106781186548,0.707106781186547));
#51896=DIRECTION('',(1.,0.,0.));
#51897=DIRECTION('center_axis',(1.,0.,0.));
#51898=DIRECTION('ref_axis',(0.,0.,-1.));
#51899=DIRECTION('',(0.,0.,-1.));
#51900=DIRECTION('center_axis',(-1.,0.,0.));
#51901=DIRECTION('ref_axis',(0.,-0.707106781186548,-0.707106781186547));
#51902=DIRECTION('',(0.,1.,0.));
#51903=DIRECTION('',(0.,0.,1.));
#51904=DIRECTION('',(0.,1.,0.));
#51905=DIRECTION('center_axis',(0.,-1.,0.));
#51906=DIRECTION('ref_axis',(0.,0.,-1.));
#51907=DIRECTION('',(0.,0.,-1.));
#51908=DIRECTION('',(-1.,0.,0.));
#51909=DIRECTION('center_axis',(1.,0.,0.));
#51910=DIRECTION('ref_axis',(0.,-0.707106781186548,-0.707106781186547));
#51911=DIRECTION('center_axis',(1.,0.,0.));
#51912=DIRECTION('ref_axis',(0.,-0.707106781186548,-0.707106781186547));
#51913=DIRECTION('',(1.,0.,0.));
#51914=DIRECTION('center_axis',(1.,0.,0.));
#51915=DIRECTION('ref_axis',(0.,-0.500000000000001,-0.866025403784438));
#51916=DIRECTION('center_axis',(-1.,0.,0.));
#51917=DIRECTION('ref_axis',(0.,-0.500000000000001,-0.866025403784438));
#51918=DIRECTION('',(-1.,0.,0.));
#51919=DIRECTION('center_axis',(1.,0.,0.));
#51920=DIRECTION('ref_axis',(0.,-0.500000000000001,-0.866025403784438));
#51921=DIRECTION('',(1.,0.,0.));
#51922=DIRECTION('center_axis',(0.,0.258819045102521,-0.965925826289068));
#51923=DIRECTION('ref_axis',(0.,0.965925826289068,0.258819045102521));
#51924=DIRECTION('',(0.,0.965925826289068,0.258819045102521));
#51925=DIRECTION('',(-1.,0.,0.));
#51926=DIRECTION('',(0.,0.965925826289068,0.258819045102521));
#51927=DIRECTION('center_axis',(-1.,0.,0.));
#51928=DIRECTION('ref_axis',(0.,0.,1.));
#51929=DIRECTION('center_axis',(1.,0.,0.));
#51930=DIRECTION('ref_axis',(0.,0.870686243840935,0.49183886058969));
#51931=DIRECTION('center_axis',(1.,0.,0.));
#51932=DIRECTION('ref_axis',(0.,0.866025403784439,-0.5));
#51933=DIRECTION('center_axis',(1.,0.,0.));
#51934=DIRECTION('ref_axis',(0.,0.00939817408142913,-0.999955836186746));
#51935=DIRECTION('center_axis',(1.,0.,0.));
#51936=DIRECTION('ref_axis',(0.,-0.870686243840935,-0.49183886058969));
#51937=DIRECTION('center_axis',(1.,0.,0.));
#51938=DIRECTION('ref_axis',(0.,-0.866025403784438,0.500000000000001));
#51939=DIRECTION('center_axis',(1.,0.,0.));
#51940=DIRECTION('ref_axis',(0.,-1.25707743249494E-14,1.));
#51941=DIRECTION('',(0.,-1.,0.));
#51942=DIRECTION('center_axis',(1.,0.,0.));
#51943=DIRECTION('ref_axis',(0.,0.,-1.));
#51944=DIRECTION('',(0.,0.258819045102521,-0.965925826289068));
#51945=DIRECTION('center_axis',(1.,0.,0.));
#51946=DIRECTION('ref_axis',(0.,-0.866025403784438,0.500000000000001));
#51947=DIRECTION('',(0.,-0.965925826289068,-0.258819045102521));
#51948=DIRECTION('center_axis',(1.,0.,0.));
#51949=DIRECTION('ref_axis',(0.,0.,-1.));
#51950=DIRECTION('',(0.,0.866025403784439,0.5));
#51951=DIRECTION('center_axis',(1.,0.,0.));
#51952=DIRECTION('ref_axis',(0.,-0.258819045102523,-0.965925826289068));
#51953=DIRECTION('',(0.,0.5,-0.866025403784439));
#51954=DIRECTION('center_axis',(1.,0.,0.));
#51955=DIRECTION('ref_axis',(0.,-0.965925826289069,0.258819045102519));
#51956=DIRECTION('',(0.,-0.866025403784439,-0.5));
#51957=DIRECTION('center_axis',(1.,0.,0.));
#51958=DIRECTION('ref_axis',(0.,0.,-1.));
#51959=DIRECTION('',(0.,0.707106781186548,0.707106781186548));
#51960=DIRECTION('center_axis',(1.,0.,0.));
#51961=DIRECTION('ref_axis',(0.,0.,-1.));
#51962=DIRECTION('',(0.,0.707106781186548,-0.707106781186548));
#51963=DIRECTION('center_axis',(1.,0.,0.));
#51964=DIRECTION('ref_axis',(0.,-1.,0.));
#51965=DIRECTION('',(0.,-0.707106781186548,-0.707106781186548));
#51966=DIRECTION('center_axis',(1.,0.,0.));
#51967=DIRECTION('ref_axis',(0.,0.,-1.));
#51968=DIRECTION('',(0.,0.5,0.866025403784439));
#51969=DIRECTION('center_axis',(1.,0.,0.));
#51970=DIRECTION('ref_axis',(0.,0.25881904510252,-0.965925826289069));
#51971=DIRECTION('',(0.,0.866025403784439,-0.5));
#51972=DIRECTION('center_axis',(1.,0.,0.));
#51973=DIRECTION('ref_axis',(0.,-0.965925826289068,-0.258819045102523));
#51974=DIRECTION('',(0.,-0.5,-0.866025403784439));
#51975=DIRECTION('center_axis',(1.,0.,0.));
#51976=DIRECTION('ref_axis',(0.,0.,-1.));
#51977=DIRECTION('',(0.,0.258819045102521,0.965925826289068));
#51978=DIRECTION('center_axis',(1.,0.,0.));
#51979=DIRECTION('ref_axis',(0.,0.499999999999999,-0.866025403784439));
#51980=DIRECTION('',(0.,0.965925826289068,-0.258819045102521));
#51981=DIRECTION('center_axis',(1.,0.,0.));
#51982=DIRECTION('ref_axis',(0.,-0.866025403784438,-0.500000000000002));
#51983=DIRECTION('',(0.,-0.258819045102521,-0.965925826289068));
#51984=DIRECTION('center_axis',(1.,0.,0.));
#51985=DIRECTION('ref_axis',(0.,0.,-1.));
#51986=DIRECTION('',(0.,6.12323399573677E-17,1.));
#51987=DIRECTION('center_axis',(1.,0.,0.));
#51988=DIRECTION('ref_axis',(0.,0.707106781186547,-0.707106781186548));
#51989=DIRECTION('',(0.,1.,-6.12323399573677E-17));
#51990=DIRECTION('center_axis',(1.,0.,0.));
#51991=DIRECTION('ref_axis',(0.,-0.707106781186547,-0.707106781186548));
#51992=DIRECTION('',(0.,-6.12323399573677E-17,-1.));
#51993=DIRECTION('center_axis',(1.,0.,0.));
#51994=DIRECTION('ref_axis',(0.,0.,-1.));
#51995=DIRECTION('',(0.,-0.258819045102521,0.965925826289068));
#51996=DIRECTION('center_axis',(1.,0.,0.));
#51997=DIRECTION('ref_axis',(0.,0.866025403784438,-0.500000000000002));
#51998=DIRECTION('',(0.,0.965925826289068,0.258819045102521));
#51999=DIRECTION('center_axis',(1.,0.,0.));
#52000=DIRECTION('ref_axis',(0.,-0.500000000000001,-0.866025403784438));
#52001=DIRECTION('',(0.,0.258819045102521,-0.965925826289068));
#52002=DIRECTION('center_axis',(1.,0.,0.));
#52003=DIRECTION('ref_axis',(0.,0.,-1.));
#52004=DIRECTION('',(0.,-0.5,0.866025403784439));
#52005=DIRECTION('center_axis',(1.,0.,0.));
#52006=DIRECTION('ref_axis',(0.,0.965925826289068,-0.258819045102523));
#52007=DIRECTION('',(0.,0.866025403784439,0.5));
#52008=DIRECTION('center_axis',(1.,0.,0.));
#52009=DIRECTION('ref_axis',(0.,-0.25881904510252,-0.965925826289069));
#52010=DIRECTION('',(0.,0.5,-0.866025403784439));
#52011=DIRECTION('center_axis',(1.,0.,0.));
#52012=DIRECTION('ref_axis',(0.,0.,-1.));
#52013=DIRECTION('',(0.,-0.707106781186547,0.707106781186548));
#52014=DIRECTION('center_axis',(1.,0.,0.));
#52015=DIRECTION('ref_axis',(0.,1.,0.));
#52016=DIRECTION('',(0.,0.707106781186548,0.707106781186547));
#52017=DIRECTION('center_axis',(1.,0.,0.));
#52018=DIRECTION('ref_axis',(0.,0.,-1.));
#52019=DIRECTION('',(0.,0.707106781186547,-0.707106781186548));
#52020=DIRECTION('center_axis',(1.,0.,0.));
#52021=DIRECTION('ref_axis',(0.,0.,-1.));
#52022=DIRECTION('',(0.,-0.866025403784438,0.5));
#52023=DIRECTION('center_axis',(1.,0.,0.));
#52024=DIRECTION('ref_axis',(0.,0.965925826289069,0.258819045102519));
#52025=DIRECTION('',(0.,0.5,0.866025403784438));
#52026=DIRECTION('center_axis',(1.,0.,0.));
#52027=DIRECTION('ref_axis',(0.,0.258819045102523,-0.965925826289068));
#52028=DIRECTION('',(0.,0.866025403784438,-0.5));
#52029=DIRECTION('center_axis',(1.,0.,0.));
#52030=DIRECTION('ref_axis',(0.,0.,-1.));
#52031=DIRECTION('',(0.,-0.965925826289068,0.258819045102521));
#52032=DIRECTION('center_axis',(1.,0.,0.));
#52033=DIRECTION('ref_axis',(0.,0.866025403784439,0.499999999999999));
#52034=DIRECTION('',(0.,0.258819045102521,0.965925826289068));
#52035=DIRECTION('center_axis',(1.,0.,0.));
#52036=DIRECTION('ref_axis',(0.,0.500000000000002,-0.866025403784438));
#52037=DIRECTION('',(0.,0.965925826289068,-0.258819045102521));
#52038=DIRECTION('center_axis',(1.,0.,0.));
#52039=DIRECTION('ref_axis',(0.,0.,-1.));
#52040=DIRECTION('',(0.,-1.,1.22464679914735E-16));
#52041=DIRECTION('center_axis',(1.,0.,0.));
#52042=DIRECTION('ref_axis',(0.,0.707106781186548,0.707106781186547));
#52043=DIRECTION('',(0.,1.22464679914735E-16,1.));
#52044=DIRECTION('center_axis',(1.,0.,0.));
#52045=DIRECTION('ref_axis',(0.,0.707106781186548,-0.707106781186547));
#52046=DIRECTION('',(0.,1.,-1.22464679914735E-16));
#52047=DIRECTION('center_axis',(1.,0.,0.));
#52048=DIRECTION('ref_axis',(0.,0.,-1.));
#52049=DIRECTION('',(0.,-0.965925826289068,-0.25881904510252));
#52050=DIRECTION('center_axis',(1.,0.,0.));
#52051=DIRECTION('ref_axis',(0.,0.500000000000002,0.866025403784438));
#52052=DIRECTION('',(0.,-0.25881904510252,0.965925826289068));
#52053=DIRECTION('center_axis',(1.,0.,0.));
#52054=DIRECTION('ref_axis',(0.,0.866025403784439,-0.499999999999999));
#52055=DIRECTION('',(0.,0.965925826289068,0.25881904510252));
#52056=DIRECTION('center_axis',(1.,0.,0.));
#52057=DIRECTION('ref_axis',(0.,0.,-1.));
#52058=DIRECTION('',(0.,-0.866025403784439,-0.5));
#52059=DIRECTION('center_axis',(1.,0.,0.));
#52060=DIRECTION('ref_axis',(0.,0.258819045102516,0.965925826289069));
#52061=DIRECTION('',(0.,-0.5,0.866025403784439));
#52062=DIRECTION('center_axis',(1.,0.,0.));
#52063=DIRECTION('ref_axis',(0.,0.965925826289069,-0.25881904510252));
#52064=DIRECTION('',(0.,0.866025403784439,0.5));
#52065=DIRECTION('center_axis',(1.,0.,0.));
#52066=DIRECTION('ref_axis',(0.,0.,-1.));
#52067=DIRECTION('',(0.,-0.707106781186548,-0.707106781186547));
#52068=DIRECTION('center_axis',(1.,0.,0.));
#52069=DIRECTION('ref_axis',(0.,0.,1.));
#52070=DIRECTION('',(0.,-0.707106781186547,0.707106781186548));
#52071=DIRECTION('center_axis',(1.,0.,0.));
#52072=DIRECTION('ref_axis',(0.,1.,0.));
#52073=DIRECTION('',(0.,0.707106781186548,0.707106781186547));
#52074=DIRECTION('center_axis',(1.,0.,0.));
#52075=DIRECTION('ref_axis',(0.,0.,-1.));
#52076=DIRECTION('',(0.,-0.5,-0.866025403784438));
#52077=DIRECTION('center_axis',(1.,0.,0.));
#52078=DIRECTION('ref_axis',(0.,-0.25881904510252,0.965925826289069));
#52079=DIRECTION('',(0.,-0.866025403784438,0.5));
#52080=DIRECTION('center_axis',(1.,0.,0.));
#52081=DIRECTION('ref_axis',(0.,0.965925826289069,0.258819045102516));
#52082=DIRECTION('',(0.,0.5,0.866025403784438));
#52083=DIRECTION('center_axis',(1.,0.,0.));
#52084=DIRECTION('ref_axis',(0.,0.,-1.));
#52085=DIRECTION('',(0.,-0.258819045102522,-0.965925826289068));
#52086=DIRECTION('center_axis',(1.,0.,0.));
#52087=DIRECTION('ref_axis',(0.,-0.500000000000004,0.866025403784436));
#52088=DIRECTION('',(0.,-0.965925826289068,0.258819045102522));
#52089=DIRECTION('center_axis',(1.,0.,0.));
#52090=DIRECTION('ref_axis',(0.,0.866025403784441,0.499999999999996));
#52091=DIRECTION('',(0.,0.258819045102522,0.965925826289068));
#52092=DIRECTION('center_axis',(1.,0.,0.));
#52093=DIRECTION('ref_axis',(0.,0.,-1.));
#52094=DIRECTION('',(0.,-1.83697019872103E-16,-1.));
#52095=DIRECTION('center_axis',(1.,0.,0.));
#52096=DIRECTION('ref_axis',(0.,-0.707106781186547,0.707106781186548));
#52097=DIRECTION('',(0.,-1.,1.83697019872103E-16));
#52098=DIRECTION('center_axis',(1.,0.,0.));
#52099=DIRECTION('ref_axis',(0.,0.707106781186547,0.707106781186548));
#52100=DIRECTION('',(0.,1.83697019872103E-16,1.));
#52101=DIRECTION('center_axis',(1.,0.,0.));
#52102=DIRECTION('ref_axis',(0.,0.,-1.));
#52103=DIRECTION('',(0.,0.25881904510252,-0.965925826289068));
#52104=DIRECTION('center_axis',(1.,0.,0.));
#52105=DIRECTION('ref_axis',(0.,-0.866025403784438,0.500000000000001));
#52106=DIRECTION('',(0.,-0.965925826289068,-0.25881904510252));
#52107=DIRECTION('center_axis',(1.,0.,0.));
#52108=DIRECTION('ref_axis',(0.,0.499999999999998,0.86602540378444));
#52109=DIRECTION('',(0.,-0.25881904510252,0.965925826289068));
#52110=DIRECTION('center_axis',(1.,0.,0.));
#52111=DIRECTION('ref_axis',(0.,0.,-1.));
#52112=DIRECTION('',(0.,0.499999999999999,-0.866025403784439));
#52113=DIRECTION('center_axis',(1.,0.,0.));
#52114=DIRECTION('ref_axis',(0.,-0.965925826289068,0.258819045102523));
#52115=DIRECTION('',(0.,-0.866025403784439,-0.499999999999999));
#52116=DIRECTION('center_axis',(1.,0.,0.));
#52117=DIRECTION('ref_axis',(0.,0.258819045102522,0.965925826289068));
#52118=DIRECTION('',(0.,-0.499999999999999,0.866025403784439));
#52119=DIRECTION('center_axis',(1.,0.,0.));
#52120=DIRECTION('ref_axis',(0.,0.,-1.));
#52121=DIRECTION('',(0.,0.707106781186547,-0.707106781186548));
#52122=DIRECTION('center_axis',(1.,0.,0.));
#52123=DIRECTION('ref_axis',(0.,-1.,0.));
#52124=DIRECTION('',(0.,-0.707106781186548,-0.707106781186547));
#52125=DIRECTION('center_axis',(1.,0.,0.));
#52126=DIRECTION('ref_axis',(0.,0.,1.));
#52127=DIRECTION('',(0.,-0.707106781186547,0.707106781186548));
#52128=DIRECTION('center_axis',(1.,0.,0.));
#52129=DIRECTION('ref_axis',(0.,0.,-1.));
#52130=DIRECTION('',(0.,0.866025403784438,-0.5));
#52131=DIRECTION('center_axis',(1.,0.,0.));
#52132=DIRECTION('ref_axis',(0.,-0.965925826289069,-0.25881904510252));
#52133=DIRECTION('',(0.,-0.5,-0.866025403784438));
#52134=DIRECTION('center_axis',(1.,0.,0.));
#52135=DIRECTION('ref_axis',(0.,-0.258819045102516,0.965925826289069));
#52136=DIRECTION('',(0.,-0.866025403784438,0.5));
#52137=DIRECTION('center_axis',(1.,0.,0.));
#52138=DIRECTION('ref_axis',(0.,0.,-1.));
#52139=DIRECTION('',(0.,0.965925826289068,-0.258819045102522));
#52140=DIRECTION('center_axis',(1.,0.,0.));
#52141=DIRECTION('ref_axis',(0.,-0.866025403784437,-0.500000000000003));
#52142=DIRECTION('',(0.,-0.258819045102522,-0.965925826289068));
#52143=DIRECTION('center_axis',(1.,0.,0.));
#52144=DIRECTION('ref_axis',(0.,-0.499999999999996,0.866025403784441));
#52145=DIRECTION('',(0.,-0.965925826289068,0.258819045102522));
#52146=DIRECTION('center_axis',(1.,0.,0.));
#52147=DIRECTION('ref_axis',(0.,0.,-1.));
#52148=DIRECTION('',(0.,1.,0.));
#52149=DIRECTION('center_axis',(1.,0.,0.));
#52150=DIRECTION('ref_axis',(0.,-0.866025403784438,0.500000000000001));
#52151=DIRECTION('center_axis',(-1.,0.,0.));
#52152=DIRECTION('ref_axis',(0.,-0.866025403784438,0.500000000000001));
#52153=DIRECTION('',(-1.,0.,0.));
#52154=DIRECTION('',(1.,0.,0.));
#52155=DIRECTION('center_axis',(0.,-0.258819045102521,0.965925826289068));
#52156=DIRECTION('ref_axis',(0.,-0.965925826289068,-0.258819045102521));
#52157=DIRECTION('',(0.,-0.965925826289068,-0.258819045102521));
#52158=DIRECTION('',(1.,0.,0.));
#52159=DIRECTION('center_axis',(1.,0.,0.));
#52160=DIRECTION('ref_axis',(0.,0.,-1.));
#52161=DIRECTION('center_axis',(1.,0.,0.));
#52162=DIRECTION('ref_axis',(0.,0.,-1.));
#52163=DIRECTION('center_axis',(-1.,0.,0.));
#52164=DIRECTION('ref_axis',(0.,0.866025403784439,0.5));
#52165=DIRECTION('center_axis',(1.,0.,0.));
#52166=DIRECTION('ref_axis',(0.,0.,-1.));
#52167=DIRECTION('',(0.,-0.707106781186548,-0.707106781186548));
#52168=DIRECTION('center_axis',(-1.,0.,0.));
#52169=DIRECTION('ref_axis',(0.,-1.,0.));
#52170=DIRECTION('',(0.,0.707106781186548,-0.707106781186548));
#52171=DIRECTION('center_axis',(-1.,0.,0.));
#52172=DIRECTION('ref_axis',(0.,0.,-1.));
#52173=DIRECTION('',(0.,0.707106781186548,0.707106781186548));
#52174=DIRECTION('center_axis',(1.,0.,0.));
#52175=DIRECTION('ref_axis',(0.,0.,-1.));
#52176=DIRECTION('',(0.,-0.866025403784439,-0.5));
#52177=DIRECTION('center_axis',(-1.,0.,0.));
#52178=DIRECTION('ref_axis',(0.,-0.965925826289069,0.258819045102519));
#52179=DIRECTION('',(0.,0.5,-0.866025403784439));
#52180=DIRECTION('center_axis',(-1.,0.,0.));
#52181=DIRECTION('ref_axis',(0.,-0.258819045102523,-0.965925826289068));
#52182=DIRECTION('',(0.,0.866025403784439,0.5));
#52183=DIRECTION('center_axis',(1.,0.,0.));
#52184=DIRECTION('ref_axis',(0.,0.,-1.));
#52185=DIRECTION('',(0.,0.258819045102521,-0.965925826289068));
#52186=DIRECTION('center_axis',(1.,0.,0.));
#52187=DIRECTION('ref_axis',(0.,-0.258819045102523,-0.965925826289068));
#52188=DIRECTION('',(-1.,0.,0.));
#52189=DIRECTION('',(1.,0.,0.));
#52190=DIRECTION('center_axis',(0.,-0.866025403784439,-0.5));
#52191=DIRECTION('ref_axis',(0.,0.5,-0.866025403784439));
#52192=DIRECTION('',(1.,0.,0.));
#52193=DIRECTION('center_axis',(1.,0.,0.));
#52194=DIRECTION('ref_axis',(0.,-0.965925826289069,0.258819045102519));
#52195=DIRECTION('',(-1.,0.,0.));
#52196=DIRECTION('center_axis',(1.,0.,0.));
#52197=DIRECTION('ref_axis',(0.,-1.,0.));
#52198=DIRECTION('',(-1.,0.,0.));
#52199=DIRECTION('',(1.,0.,0.));
#52200=DIRECTION('center_axis',(0.,-0.707106781186548,-0.707106781186548));
#52201=DIRECTION('ref_axis',(0.,0.707106781186548,-0.707106781186548));
#52202=DIRECTION('',(-1.,0.,0.));
#52203=DIRECTION('center_axis',(1.,0.,0.));
#52204=DIRECTION('ref_axis',(0.,0.,-1.));
#52205=DIRECTION('',(1.,0.,0.));
#52206=DIRECTION('center_axis',(1.,0.,0.));
#52207=DIRECTION('ref_axis',(0.,-0.965925826289068,-0.258819045102523));
#52208=DIRECTION('center_axis',(-1.,0.,0.));
#52209=DIRECTION('ref_axis',(0.,-0.965925826289068,-0.258819045102523));
#52210=DIRECTION('',(-1.,0.,0.));
#52211=DIRECTION('',(1.,0.,0.));
#52212=DIRECTION('center_axis',(1.,0.,0.));
#52213=DIRECTION('ref_axis',(0.,0.,-1.));
#52214=DIRECTION('',(0.,0.866025403784439,-0.5));
#52215=DIRECTION('center_axis',(-1.,0.,0.));
#52216=DIRECTION('ref_axis',(0.,0.25881904510252,-0.965925826289069));
#52217=DIRECTION('',(0.,0.5,0.866025403784439));
#52218=DIRECTION('',(0.,-0.866025403784439,0.5));
#52219=DIRECTION('',(0.,0.5,0.866025403784439));
#52220=DIRECTION('center_axis',(0.,-0.5,-0.866025403784439));
#52221=DIRECTION('ref_axis',(0.,0.866025403784439,-0.5));
#52222=DIRECTION('',(-1.,0.,0.));
#52223=DIRECTION('center_axis',(1.,0.,0.));
#52224=DIRECTION('ref_axis',(0.,0.25881904510252,-0.965925826289069));
#52225=DIRECTION('',(1.,0.,0.));
#52226=DIRECTION('center_axis',(1.,0.,0.));
#52227=DIRECTION('ref_axis',(0.,-0.866025403784438,-0.500000000000002));
#52228=DIRECTION('center_axis',(-1.,0.,0.));
#52229=DIRECTION('ref_axis',(0.,-0.866025403784438,-0.500000000000002));
#52230=DIRECTION('',(-1.,0.,0.));
#52231=DIRECTION('',(1.,0.,0.));
#52232=DIRECTION('center_axis',(1.,0.,0.));
#52233=DIRECTION('ref_axis',(0.,0.,-1.));
#52234=DIRECTION('',(0.,0.965925826289068,-0.258819045102521));
#52235=DIRECTION('center_axis',(-1.,0.,0.));
#52236=DIRECTION('ref_axis',(0.,0.499999999999999,-0.866025403784439));
#52237=DIRECTION('',(0.,0.258819045102521,0.965925826289068));
#52238=DIRECTION('center_axis',(1.,0.,0.));
#52239=DIRECTION('ref_axis',(0.,0.,-1.));
#52240=DIRECTION('center_axis',(-1.,0.,0.));
#52241=DIRECTION('ref_axis',(0.,-0.0101818638820796,0.999948163480431));
#52242=DIRECTION('center_axis',(1.,0.,0.));
#52243=DIRECTION('ref_axis',(0.,0.,-1.));
#52244=DIRECTION('',(0.,0.258819045102521,-0.965925826289068));
#52245=DIRECTION('center_axis',(-1.,0.,0.));
#52246=DIRECTION('ref_axis',(0.,-0.500000000000001,-0.866025403784438));
#52247=DIRECTION('',(0.,0.965925826289068,0.258819045102521));
#52248=DIRECTION('center_axis',(-1.,0.,0.));
#52249=DIRECTION('ref_axis',(0.,0.866025403784438,-0.500000000000002));
#52250=DIRECTION('',(0.,-0.258819045102521,0.965925826289068));
#52251=DIRECTION('center_axis',(1.,0.,0.));
#52252=DIRECTION('ref_axis',(0.,0.,-1.));
#52253=DIRECTION('',(0.,-6.12323399573677E-17,-1.));
#52254=DIRECTION('center_axis',(-1.,0.,0.));
#52255=DIRECTION('ref_axis',(0.,-0.707106781186547,-0.707106781186548));
#52256=DIRECTION('',(0.,1.,-6.12323399573677E-17));
#52257=DIRECTION('center_axis',(-1.,0.,0.));
#52258=DIRECTION('ref_axis',(0.,0.707106781186547,-0.707106781186548));
#52259=DIRECTION('',(0.,6.12323399573677E-17,1.));
#52260=DIRECTION('center_axis',(1.,0.,0.));
#52261=DIRECTION('ref_axis',(0.,0.,-1.));
#52262=DIRECTION('',(0.,-0.258819045102521,-0.965925826289068));
#52263=DIRECTION('center_axis',(0.,-0.258819045102521,-0.965925826289068));
#52264=DIRECTION('ref_axis',(0.,0.965925826289068,-0.258819045102521));
#52265=DIRECTION('',(-1.,0.,0.));
#52266=DIRECTION('center_axis',(1.,0.,0.));
#52267=DIRECTION('ref_axis',(0.,0.499999999999999,-0.866025403784439));
#52268=DIRECTION('',(1.,0.,0.));
#52269=DIRECTION('center_axis',(1.,0.,0.));
#52270=DIRECTION('ref_axis',(0.,0.707106781186547,-0.707106781186548));
#52271=DIRECTION('',(-1.,0.,0.));
#52272=DIRECTION('',(1.,0.,0.));
#52273=DIRECTION('center_axis',(0.,1.,-6.12323399573677E-17));
#52274=DIRECTION('ref_axis',(0.,6.12323399573677E-17,1.));
#52275=DIRECTION('',(-1.,0.,0.));
#52276=DIRECTION('center_axis',(1.,0.,0.));
#52277=DIRECTION('ref_axis',(0.,-0.707106781186547,-0.707106781186548));
#52278=DIRECTION('',(-1.,0.,0.));
#52279=DIRECTION('',(1.,0.,0.));
#52280=DIRECTION('center_axis',(0.,-1.,6.12323399573677E-17));
#52281=DIRECTION('ref_axis',(0.,-6.12323399573677E-17,-1.));
#52282=DIRECTION('',(1.,0.,0.));
#52283=DIRECTION('center_axis',(1.,0.,0.));
#52284=DIRECTION('ref_axis',(0.,0.866025403784438,-0.500000000000002));
#52285=DIRECTION('',(-1.,0.,0.));
#52286=DIRECTION('',(1.,0.,0.));
#52287=DIRECTION('center_axis',(0.,0.965925826289068,0.258819045102521));
#52288=DIRECTION('ref_axis',(0.,-0.258819045102521,0.965925826289068));
#52289=DIRECTION('',(-1.,0.,0.));
#52290=DIRECTION('center_axis',(1.,0.,0.));
#52291=DIRECTION('ref_axis',(0.,-0.500000000000001,-0.866025403784438));
#52292=DIRECTION('',(-1.,0.,0.));
#52293=DIRECTION('',(1.,0.,0.));
#52294=DIRECTION('center_axis',(0.,-0.965925826289068,-0.258819045102521));
#52295=DIRECTION('ref_axis',(0.,0.258819045102521,-0.965925826289068));
#52296=DIRECTION('',(1.,0.,0.));
#52297=DIRECTION('center_axis',(1.,0.,0.));
#52298=DIRECTION('ref_axis',(0.,0.965925826289068,-0.258819045102523));
#52299=DIRECTION('center_axis',(-1.,0.,0.));
#52300=DIRECTION('ref_axis',(0.,0.965925826289068,-0.258819045102523));
#52301=DIRECTION('',(-1.,0.,0.));
#52302=DIRECTION('',(1.,0.,0.));
#52303=DIRECTION('center_axis',(0.,0.866025403784439,0.5));
#52304=DIRECTION('ref_axis',(0.,-0.5,0.866025403784439));
#52305=DIRECTION('',(-1.,0.,0.));
#52306=DIRECTION('center_axis',(3.00652763009229E-17,0.866025403784439,
0.5));
#52307=DIRECTION('ref_axis',(0.,-0.5,0.866025403784439));
#52308=DIRECTION('',(1.,0.,0.));
#52309=DIRECTION('',(0.,-0.5,0.866025403784439));
#52310=DIRECTION('center_axis',(1.,0.,0.));
#52311=DIRECTION('ref_axis',(0.,-0.25881904510252,-0.965925826289069));
#52312=DIRECTION('center_axis',(-1.,0.,0.));
#52313=DIRECTION('ref_axis',(0.,-0.25881904510252,-0.965925826289069));
#52314=DIRECTION('',(-1.,0.,0.));
#52315=DIRECTION('',(1.,0.,0.));
#52316=DIRECTION('center_axis',(0.,-0.866025403784439,-0.5));
#52317=DIRECTION('ref_axis',(0.,0.5,-0.866025403784439));
#52318=DIRECTION('',(0.,-0.5,0.866025403784439));
#52319=DIRECTION('',(1.,0.,0.));
#52320=DIRECTION('center_axis',(-3.00652763009229E-17,-0.866025403784439,
-0.5));
#52321=DIRECTION('ref_axis',(0.,-0.5,0.866025403784439));
#52322=DIRECTION('',(1.,0.,0.));
#52323=DIRECTION('center_axis',(1.,0.,0.));
#52324=DIRECTION('ref_axis',(0.,0.,-1.));
#52325=DIRECTION('',(0.,-0.866025403784439,-0.5));
#52326=DIRECTION('',(0.,0.866025403784439,0.5));
#52327=DIRECTION('center_axis',(1.,0.,0.));
#52328=DIRECTION('ref_axis',(0.,0.,-1.));
#52329=DIRECTION('center_axis',(-1.,0.,0.));
#52330=DIRECTION('ref_axis',(0.,0.,-1.));
#52331=DIRECTION('',(-1.,0.,0.));
#52332=DIRECTION('',(1.,0.,0.));
#52333=DIRECTION('center_axis',(1.,0.,0.));
#52334=DIRECTION('ref_axis',(0.,0.,-1.));
#52335=DIRECTION('',(0.,0.707106781186548,0.707106781186547));
#52336=DIRECTION('center_axis',(-1.,0.,0.));
#52337=DIRECTION('ref_axis',(0.,1.,0.));
#52338=DIRECTION('',(0.,-0.707106781186547,0.707106781186548));
#52339=DIRECTION('center_axis',(1.,0.,0.));
#52340=DIRECTION('ref_axis',(0.,0.,-1.));
#52341=DIRECTION('center_axis',(-1.,0.,0.));
#52342=DIRECTION('ref_axis',(0.,-0.866025403784438,0.500000000000001));
#52343=DIRECTION('center_axis',(1.,0.,0.));
#52344=DIRECTION('ref_axis',(0.,0.,-1.));
#52345=DIRECTION('',(0.,0.965925826289068,-0.258819045102521));
#52346=DIRECTION('center_axis',(-1.,0.,0.));
#52347=DIRECTION('ref_axis',(0.,0.500000000000002,-0.866025403784438));
#52348=DIRECTION('',(0.,0.258819045102521,0.965925826289068));
#52349=DIRECTION('center_axis',(-1.,0.,0.));
#52350=DIRECTION('ref_axis',(0.,0.866025403784439,0.499999999999999));
#52351=DIRECTION('',(0.,-0.965925826289068,0.258819045102521));
#52352=DIRECTION('center_axis',(1.,0.,0.));
#52353=DIRECTION('ref_axis',(0.,0.,-1.));
#52354=DIRECTION('',(0.,0.866025403784438,-0.5));
#52355=DIRECTION('center_axis',(-1.,0.,0.));
#52356=DIRECTION('ref_axis',(0.,0.258819045102523,-0.965925826289068));
#52357=DIRECTION('',(0.,0.5,0.866025403784438));
#52358=DIRECTION('center_axis',(-1.,0.,0.));
#52359=DIRECTION('ref_axis',(0.,0.965925826289069,0.258819045102519));
#52360=DIRECTION('',(0.,-0.866025403784438,0.5));
#52361=DIRECTION('center_axis',(1.,0.,0.));
#52362=DIRECTION('ref_axis',(0.,0.,-1.));
#52363=DIRECTION('',(0.,0.707106781186547,-0.707106781186548));
#52364=DIRECTION('center_axis',(0.,0.707106781186547,-0.707106781186548));
#52365=DIRECTION('ref_axis',(0.,0.707106781186548,0.707106781186547));
#52366=DIRECTION('',(-1.,0.,0.));
#52367=DIRECTION('center_axis',(1.,0.,0.));
#52368=DIRECTION('ref_axis',(0.,1.,0.));
#52369=DIRECTION('',(1.,0.,0.));
#52370=DIRECTION('center_axis',(1.,0.,0.));
#52371=DIRECTION('ref_axis',(0.,0.965925826289069,0.258819045102519));
#52372=DIRECTION('',(-1.,0.,0.));
#52373=DIRECTION('',(1.,0.,0.));
#52374=DIRECTION('center_axis',(0.,0.5,0.866025403784438));
#52375=DIRECTION('ref_axis',(0.,-0.866025403784438,0.5));
#52376=DIRECTION('',(-1.,0.,0.));
#52377=DIRECTION('center_axis',(1.,0.,0.));
#52378=DIRECTION('ref_axis',(0.,0.258819045102523,-0.965925826289068));
#52379=DIRECTION('',(-1.,0.,0.));
#52380=DIRECTION('',(1.,0.,0.));
#52381=DIRECTION('center_axis',(0.,-0.5,-0.866025403784438));
#52382=DIRECTION('ref_axis',(0.,0.866025403784438,-0.5));
#52383=DIRECTION('',(1.,0.,0.));
#52384=DIRECTION('center_axis',(1.,0.,0.));
#52385=DIRECTION('ref_axis',(0.,0.866025403784439,0.499999999999999));
#52386=DIRECTION('',(-1.,0.,0.));
#52387=DIRECTION('',(1.,0.,0.));
#52388=DIRECTION('center_axis',(0.,0.258819045102521,0.965925826289068));
#52389=DIRECTION('ref_axis',(0.,-0.965925826289068,0.258819045102521));
#52390=DIRECTION('',(-1.,0.,0.));
#52391=DIRECTION('center_axis',(1.,0.,0.));
#52392=DIRECTION('ref_axis',(0.,0.500000000000002,-0.866025403784438));
#52393=DIRECTION('',(-1.,0.,0.));
#52394=DIRECTION('',(1.,0.,0.));
#52395=DIRECTION('center_axis',(0.,-0.258819045102521,-0.965925826289068));
#52396=DIRECTION('ref_axis',(0.,0.965925826289068,-0.258819045102521));
#52397=DIRECTION('',(1.,0.,0.));
#52398=DIRECTION('center_axis',(1.,0.,0.));
#52399=DIRECTION('ref_axis',(0.,0.707106781186548,0.707106781186547));
#52400=DIRECTION('center_axis',(-1.,0.,0.));
#52401=DIRECTION('ref_axis',(0.,0.707106781186548,0.707106781186547));
#52402=DIRECTION('',(-1.,0.,0.));
#52403=DIRECTION('',(1.,0.,0.));
#52404=DIRECTION('center_axis',(0.,1.22464679914735E-16,1.));
#52405=DIRECTION('ref_axis',(0.,-1.,1.22464679914735E-16));
#52406=DIRECTION('',(-1.,0.,0.));
#52407=DIRECTION('center_axis',(3.00652763009229E-17,1.28246463818759E-16,
1.));
#52408=DIRECTION('ref_axis',(1.,0.,-3.00652763009229E-17));
#52409=DIRECTION('',(1.,0.,0.));
#52410=DIRECTION('',(0.,-1.,1.22464679914735E-16));
#52411=DIRECTION('center_axis',(1.,0.,0.));
#52412=DIRECTION('ref_axis',(0.,0.707106781186548,-0.707106781186547));
#52413=DIRECTION('center_axis',(-1.,0.,0.));
#52414=DIRECTION('ref_axis',(0.,0.707106781186548,-0.707106781186547));
#52415=DIRECTION('',(-1.,0.,0.));
#52416=DIRECTION('',(1.,0.,0.));
#52417=DIRECTION('center_axis',(0.,-1.22464679914735E-16,-1.));
#52418=DIRECTION('ref_axis',(0.,1.,-1.22464679914735E-16));
#52419=DIRECTION('',(0.,-1.,1.22464679914735E-16));
#52420=DIRECTION('',(1.,0.,0.));
#52421=DIRECTION('center_axis',(-3.00652763009229E-17,-1.28246463818759E-16,
-1.));
#52422=DIRECTION('ref_axis',(1.,0.,-3.00652763009229E-17));
#52423=DIRECTION('',(1.,0.,0.));
#52424=DIRECTION('center_axis',(1.,0.,0.));
#52425=DIRECTION('ref_axis',(0.,0.,-1.));
#52426=DIRECTION('',(0.,-1.22464679914735E-16,-1.));
#52427=DIRECTION('',(0.,1.22464679914735E-16,1.));
#52428=DIRECTION('center_axis',(1.,0.,0.));
#52429=DIRECTION('ref_axis',(0.,0.866025403784439,-0.499999999999999));
#52430=DIRECTION('center_axis',(-1.,0.,0.));
#52431=DIRECTION('ref_axis',(0.,0.866025403784439,-0.499999999999999));
#52432=DIRECTION('',(-1.,0.,0.));
#52433=DIRECTION('',(1.,0.,0.));
#52434=DIRECTION('center_axis',(1.,0.,0.));
#52435=DIRECTION('ref_axis',(0.,0.,-1.));
#52436=DIRECTION('',(0.,-0.25881904510252,0.965925826289068));
#52437=DIRECTION('center_axis',(-1.,0.,0.));
#52438=DIRECTION('ref_axis',(0.,0.500000000000002,0.866025403784438));
#52439=DIRECTION('',(0.,-0.965925826289068,-0.25881904510252));
#52440=DIRECTION('center_axis',(1.,0.,0.));
#52441=DIRECTION('ref_axis',(0.,0.,-1.));
#52442=DIRECTION('center_axis',(-1.,0.,0.));
#52443=DIRECTION('ref_axis',(0.,-0.866025403784439,-0.5));
#52444=DIRECTION('center_axis',(1.,0.,0.));
#52445=DIRECTION('ref_axis',(0.,0.,-1.));
#52446=DIRECTION('',(0.,0.707106781186548,0.707106781186547));
#52447=DIRECTION('center_axis',(-1.,0.,0.));
#52448=DIRECTION('ref_axis',(0.,1.,0.));
#52449=DIRECTION('',(0.,-0.707106781186547,0.707106781186548));
#52450=DIRECTION('center_axis',(-1.,0.,0.));
#52451=DIRECTION('ref_axis',(0.,0.,1.));
#52452=DIRECTION('',(0.,-0.707106781186548,-0.707106781186547));
#52453=DIRECTION('center_axis',(1.,0.,0.));
#52454=DIRECTION('ref_axis',(0.,0.,-1.));
#52455=DIRECTION('',(0.,0.866025403784439,0.5));
#52456=DIRECTION('center_axis',(-1.,0.,0.));
#52457=DIRECTION('ref_axis',(0.,0.965925826289069,-0.25881904510252));
#52458=DIRECTION('',(0.,-0.5,0.866025403784439));
#52459=DIRECTION('center_axis',(-1.,0.,0.));
#52460=DIRECTION('ref_axis',(0.,0.258819045102516,0.965925826289069));
#52461=DIRECTION('',(0.,-0.866025403784439,-0.5));
#52462=DIRECTION('center_axis',(1.,0.,0.));
#52463=DIRECTION('ref_axis',(0.,0.,-1.));
#52464=DIRECTION('',(0.,0.965925826289068,0.25881904510252));
#52465=DIRECTION('center_axis',(0.,0.965925826289068,0.25881904510252));
#52466=DIRECTION('ref_axis',(0.,-0.25881904510252,0.965925826289068));
#52467=DIRECTION('',(-1.,0.,0.));
#52468=DIRECTION('center_axis',(1.,0.,0.));
#52469=DIRECTION('ref_axis',(0.,0.500000000000002,0.866025403784438));
#52470=DIRECTION('',(1.,0.,0.));
#52471=DIRECTION('center_axis',(1.,0.,0.));
#52472=DIRECTION('ref_axis',(0.,0.258819045102516,0.965925826289069));
#52473=DIRECTION('',(-1.,0.,0.));
#52474=DIRECTION('',(1.,0.,0.));
#52475=DIRECTION('center_axis',(0.,-0.5,0.866025403784439));
#52476=DIRECTION('ref_axis',(0.,-0.866025403784439,-0.5));
#52477=DIRECTION('',(-1.,0.,0.));
#52478=DIRECTION('center_axis',(1.,0.,0.));
#52479=DIRECTION('ref_axis',(0.,0.965925826289069,-0.25881904510252));
#52480=DIRECTION('',(-1.,0.,0.));
#52481=DIRECTION('',(1.,0.,0.));
#52482=DIRECTION('center_axis',(0.,0.5,-0.866025403784439));
#52483=DIRECTION('ref_axis',(0.,0.866025403784439,0.5));
#52484=DIRECTION('',(1.,0.,0.));
#52485=DIRECTION('center_axis',(1.,0.,0.));
#52486=DIRECTION('ref_axis',(0.,0.,1.));
#52487=DIRECTION('',(-1.,0.,0.));
#52488=DIRECTION('',(1.,0.,0.));
#52489=DIRECTION('center_axis',(0.,-0.707106781186547,0.707106781186548));
#52490=DIRECTION('ref_axis',(0.,-0.707106781186548,-0.707106781186547));
#52491=DIRECTION('',(-1.,0.,0.));
#52492=DIRECTION('center_axis',(1.,0.,0.));
#52493=DIRECTION('ref_axis',(0.,1.,0.));
#52494=DIRECTION('',(-1.,0.,0.));
#52495=DIRECTION('',(1.,0.,0.));
#52496=DIRECTION('center_axis',(0.,0.707106781186547,-0.707106781186548));
#52497=DIRECTION('ref_axis',(0.,0.707106781186548,0.707106781186547));
#52498=DIRECTION('',(1.,0.,0.));
#52499=DIRECTION('center_axis',(1.,0.,0.));
#52500=DIRECTION('ref_axis',(0.,-0.25881904510252,0.965925826289069));
#52501=DIRECTION('center_axis',(-1.,0.,0.));
#52502=DIRECTION('ref_axis',(0.,-0.25881904510252,0.965925826289069));
#52503=DIRECTION('',(-1.,0.,0.));
#52504=DIRECTION('',(1.,0.,0.));
#52505=DIRECTION('center_axis',(0.,-0.866025403784438,0.5));
#52506=DIRECTION('ref_axis',(0.,-0.5,-0.866025403784438));
#52507=DIRECTION('',(-1.,0.,0.));
#52508=DIRECTION('center_axis',(3.00652763009229E-17,-0.866025403784438,
0.5));
#52509=DIRECTION('ref_axis',(1.,0.,-6.01305526018457E-17));
#52510=DIRECTION('',(1.,0.,0.));
#52511=DIRECTION('',(0.,-0.5,-0.866025403784438));
#52512=DIRECTION('center_axis',(1.,0.,0.));
#52513=DIRECTION('ref_axis',(0.,0.965925826289069,0.258819045102516));
#52514=DIRECTION('center_axis',(-1.,0.,0.));
#52515=DIRECTION('ref_axis',(0.,0.965925826289069,0.258819045102516));
#52516=DIRECTION('',(-1.,0.,0.));
#52517=DIRECTION('',(1.,0.,0.));
#52518=DIRECTION('center_axis',(0.,0.866025403784438,-0.5));
#52519=DIRECTION('ref_axis',(0.,0.5,0.866025403784438));
#52520=DIRECTION('',(0.,-0.5,-0.866025403784438));
#52521=DIRECTION('',(1.,0.,0.));
#52522=DIRECTION('center_axis',(-3.00652763009229E-17,0.866025403784438,
-0.5));
#52523=DIRECTION('ref_axis',(1.,0.,-6.01305526018457E-17));
#52524=DIRECTION('',(1.,0.,0.));
#52525=DIRECTION('center_axis',(1.,0.,0.));
#52526=DIRECTION('ref_axis',(0.,0.,-1.));
#52527=DIRECTION('',(0.,0.866025403784438,-0.5));
#52528=DIRECTION('',(0.,-0.866025403784438,0.5));
#52529=DIRECTION('center_axis',(1.,0.,0.));
#52530=DIRECTION('ref_axis',(0.,0.866025403784441,0.499999999999996));
#52531=DIRECTION('center_axis',(-1.,0.,0.));
#52532=DIRECTION('ref_axis',(0.,0.866025403784441,0.499999999999996));
#52533=DIRECTION('',(-1.,0.,0.));
#52534=DIRECTION('',(1.,0.,0.));
#52535=DIRECTION('center_axis',(1.,0.,0.));
#52536=DIRECTION('ref_axis',(0.,0.,-1.));
#52537=DIRECTION('',(0.,-0.965925826289068,0.258819045102522));
#52538=DIRECTION('center_axis',(-1.,0.,0.));
#52539=DIRECTION('ref_axis',(0.,-0.500000000000004,0.866025403784436));
#52540=DIRECTION('',(0.,-0.258819045102522,-0.965925826289068));
#52541=DIRECTION('center_axis',(1.,0.,0.));
#52542=DIRECTION('ref_axis',(0.,0.,-1.));
#52543=DIRECTION('center_axis',(-1.,0.,0.));
#52544=DIRECTION('ref_axis',(0.,0.0101818638820808,-0.999948163480431));
#52545=DIRECTION('center_axis',(1.,0.,0.));
#52546=DIRECTION('ref_axis',(0.,0.,-1.));
#52547=DIRECTION('',(0.,-0.25881904510252,0.965925826289068));
#52548=DIRECTION('center_axis',(-1.,0.,0.));
#52549=DIRECTION('ref_axis',(0.,0.499999999999998,0.86602540378444));
#52550=DIRECTION('',(0.,-0.965925826289068,-0.25881904510252));
#52551=DIRECTION('center_axis',(-1.,0.,0.));
#52552=DIRECTION('ref_axis',(0.,-0.866025403784438,0.500000000000001));
#52553=DIRECTION('',(0.,0.25881904510252,-0.965925826289068));
#52554=DIRECTION('center_axis',(1.,0.,0.));
#52555=DIRECTION('ref_axis',(0.,0.,-1.));
#52556=DIRECTION('',(0.,1.83697019872103E-16,1.));
#52557=DIRECTION('center_axis',(-1.,0.,0.));
#52558=DIRECTION('ref_axis',(0.,0.707106781186547,0.707106781186548));
#52559=DIRECTION('',(0.,-1.,1.83697019872103E-16));
#52560=DIRECTION('center_axis',(-1.,0.,0.));
#52561=DIRECTION('ref_axis',(0.,-0.707106781186547,0.707106781186548));
#52562=DIRECTION('',(0.,-1.83697019872103E-16,-1.));
#52563=DIRECTION('center_axis',(1.,0.,0.));
#52564=DIRECTION('ref_axis',(0.,0.,-1.));
#52565=DIRECTION('',(0.,0.258819045102522,0.965925826289068));
#52566=DIRECTION('center_axis',(0.,0.258819045102522,0.965925826289068));
#52567=DIRECTION('ref_axis',(0.,-0.965925826289068,0.258819045102522));
#52568=DIRECTION('',(-1.,0.,0.));
#52569=DIRECTION('center_axis',(1.,0.,0.));
#52570=DIRECTION('ref_axis',(0.,-0.500000000000004,0.866025403784436));
#52571=DIRECTION('',(1.,0.,0.));
#52572=DIRECTION('center_axis',(1.,0.,0.));
#52573=DIRECTION('ref_axis',(0.,-0.707106781186547,0.707106781186548));
#52574=DIRECTION('',(-1.,0.,0.));
#52575=DIRECTION('',(1.,0.,0.));
#52576=DIRECTION('center_axis',(0.,-1.,1.83697019872103E-16));
#52577=DIRECTION('ref_axis',(0.,-1.83697019872103E-16,-1.));
#52578=DIRECTION('',(-1.,0.,0.));
#52579=DIRECTION('center_axis',(1.,0.,0.));
#52580=DIRECTION('ref_axis',(0.,0.707106781186547,0.707106781186548));
#52581=DIRECTION('',(-1.,0.,0.));
#52582=DIRECTION('',(1.,0.,0.));
#52583=DIRECTION('center_axis',(0.,1.,-1.83697019872103E-16));
#52584=DIRECTION('ref_axis',(0.,1.83697019872103E-16,1.));
#52585=DIRECTION('',(1.,0.,0.));
#52586=DIRECTION('center_axis',(1.,0.,0.));
#52587=DIRECTION('ref_axis',(0.,-0.866025403784438,0.500000000000001));
#52588=DIRECTION('',(-1.,0.,0.));
#52589=DIRECTION('',(1.,0.,0.));
#52590=DIRECTION('center_axis',(0.,-0.965925826289068,-0.25881904510252));
#52591=DIRECTION('ref_axis',(0.,0.25881904510252,-0.965925826289068));
#52592=DIRECTION('',(-1.,0.,0.));
#52593=DIRECTION('center_axis',(1.,0.,0.));
#52594=DIRECTION('ref_axis',(0.,0.499999999999998,0.86602540378444));
#52595=DIRECTION('',(-1.,0.,0.));
#52596=DIRECTION('',(1.,0.,0.));
#52597=DIRECTION('center_axis',(0.,0.965925826289068,0.25881904510252));
#52598=DIRECTION('ref_axis',(0.,-0.25881904510252,0.965925826289068));
#52599=DIRECTION('',(1.,0.,0.));
#52600=DIRECTION('center_axis',(1.,0.,0.));
#52601=DIRECTION('ref_axis',(0.,-0.965925826289068,0.258819045102523));
#52602=DIRECTION('center_axis',(-1.,0.,0.));
#52603=DIRECTION('ref_axis',(0.,-0.965925826289068,0.258819045102523));
#52604=DIRECTION('',(-1.,0.,0.));
#52605=DIRECTION('',(1.,0.,0.));
#52606=DIRECTION('center_axis',(0.,-0.866025403784439,-0.499999999999999));
#52607=DIRECTION('ref_axis',(0.,0.499999999999999,-0.866025403784439));
#52608=DIRECTION('',(-1.,0.,0.));
#52609=DIRECTION('center_axis',(3.00652763009229E-17,-0.866025403784439,
-0.499999999999999));
#52610=DIRECTION('ref_axis',(0.,0.499999999999999,-0.866025403784439));
#52611=DIRECTION('',(1.,0.,0.));
#52612=DIRECTION('',(0.,0.499999999999999,-0.866025403784439));
#52613=DIRECTION('center_axis',(1.,0.,0.));
#52614=DIRECTION('ref_axis',(0.,0.258819045102522,0.965925826289068));
#52615=DIRECTION('center_axis',(-1.,0.,0.));
#52616=DIRECTION('ref_axis',(0.,0.258819045102522,0.965925826289068));
#52617=DIRECTION('',(-1.,0.,0.));
#52618=DIRECTION('',(1.,0.,0.));
#52619=DIRECTION('center_axis',(0.,0.866025403784439,0.499999999999999));
#52620=DIRECTION('ref_axis',(0.,-0.499999999999999,0.866025403784439));
#52621=DIRECTION('',(0.,0.499999999999999,-0.866025403784439));
#52622=DIRECTION('',(1.,0.,0.));
#52623=DIRECTION('center_axis',(-3.00652763009229E-17,0.866025403784439,
0.499999999999999));
#52624=DIRECTION('ref_axis',(0.,0.499999999999999,-0.866025403784439));
#52625=DIRECTION('',(1.,0.,0.));
#52626=DIRECTION('center_axis',(1.,0.,0.));
#52627=DIRECTION('ref_axis',(0.,0.,-1.));
#52628=DIRECTION('',(0.,0.866025403784439,0.499999999999999));
#52629=DIRECTION('',(0.,-0.866025403784439,-0.499999999999999));
#52630=DIRECTION('center_axis',(1.,0.,0.));
#52631=DIRECTION('ref_axis',(0.,0.,1.));
#52632=DIRECTION('center_axis',(-1.,0.,0.));
#52633=DIRECTION('ref_axis',(0.,0.,1.));
#52634=DIRECTION('',(-1.,0.,0.));
#52635=DIRECTION('',(1.,0.,0.));
#52636=DIRECTION('center_axis',(1.,0.,0.));
#52637=DIRECTION('ref_axis',(0.,0.,-1.));
#52638=DIRECTION('',(0.,-0.707106781186548,-0.707106781186547));
#52639=DIRECTION('center_axis',(-1.,0.,0.));
#52640=DIRECTION('ref_axis',(0.,-1.,0.));
#52641=DIRECTION('',(0.,0.707106781186547,-0.707106781186548));
#52642=DIRECTION('center_axis',(1.,0.,0.));
#52643=DIRECTION('ref_axis',(0.,0.,-1.));
#52644=DIRECTION('center_axis',(-1.,0.,0.));
#52645=DIRECTION('ref_axis',(0.,0.866025403784439,-0.5));
#52646=DIRECTION('center_axis',(1.,0.,0.));
#52647=DIRECTION('ref_axis',(0.,0.,-1.));
#52648=DIRECTION('',(0.,-0.965925826289068,0.258819045102522));
#52649=DIRECTION('center_axis',(-1.,0.,0.));
#52650=DIRECTION('ref_axis',(0.,-0.499999999999996,0.866025403784441));
#52651=DIRECTION('',(0.,-0.258819045102522,-0.965925826289068));
#52652=DIRECTION('center_axis',(-1.,0.,0.));
#52653=DIRECTION('ref_axis',(0.,-0.866025403784437,-0.500000000000003));
#52654=DIRECTION('',(0.,0.965925826289068,-0.258819045102522));
#52655=DIRECTION('center_axis',(1.,0.,0.));
#52656=DIRECTION('ref_axis',(0.,0.,-1.));
#52657=DIRECTION('',(0.,-0.866025403784438,0.5));
#52658=DIRECTION('center_axis',(-1.,0.,0.));
#52659=DIRECTION('ref_axis',(0.,-0.258819045102516,0.965925826289069));
#52660=DIRECTION('',(0.,-0.5,-0.866025403784438));
#52661=DIRECTION('center_axis',(-1.,0.,0.));
#52662=DIRECTION('ref_axis',(0.,-0.965925826289069,-0.25881904510252));
#52663=DIRECTION('',(0.,0.866025403784438,-0.5));
#52664=DIRECTION('center_axis',(1.,0.,0.));
#52665=DIRECTION('ref_axis',(0.,0.,-1.));
#52666=DIRECTION('',(0.,-0.707106781186547,0.707106781186548));
#52667=DIRECTION('center_axis',(0.,-0.707106781186547,0.707106781186548));
#52668=DIRECTION('ref_axis',(0.,-0.707106781186548,-0.707106781186547));
#52669=DIRECTION('',(-1.,0.,0.));
#52670=DIRECTION('center_axis',(1.,0.,0.));
#52671=DIRECTION('ref_axis',(0.,-1.,0.));
#52672=DIRECTION('',(1.,0.,0.));
#52673=DIRECTION('center_axis',(1.,0.,0.));
#52674=DIRECTION('ref_axis',(0.,-0.965925826289069,-0.25881904510252));
#52675=DIRECTION('',(-1.,0.,0.));
#52676=DIRECTION('',(1.,0.,0.));
#52677=DIRECTION('center_axis',(0.,-0.5,-0.866025403784438));
#52678=DIRECTION('ref_axis',(0.,0.866025403784438,-0.5));
#52679=DIRECTION('',(-1.,0.,0.));
#52680=DIRECTION('center_axis',(1.,0.,0.));
#52681=DIRECTION('ref_axis',(0.,-0.258819045102516,0.965925826289069));
#52682=DIRECTION('',(-1.,0.,0.));
#52683=DIRECTION('',(1.,0.,0.));
#52684=DIRECTION('center_axis',(0.,0.5,0.866025403784438));
#52685=DIRECTION('ref_axis',(0.,-0.866025403784438,0.5));
#52686=DIRECTION('',(1.,0.,0.));
#52687=DIRECTION('center_axis',(0.921947479709935,0.342317807210672,0.181194270116296));
#52688=DIRECTION('ref_axis',(-0.127350909928393,0.709732301276181,-0.692864926421902));
#52689=DIRECTION('center_axis',(-0.902368117048407,0.426637457078594,-0.0609283312755491));
#52690=DIRECTION('ref_axis',(0.380530973474892,0.855128580231168,0.352067166174407));
#52691=DIRECTION('center_axis',(0.,0.,1.));
#52692=DIRECTION('ref_axis',(1.,0.,0.));
#52693=DIRECTION('center_axis',(0.,0.380708566256253,-0.924695078163125));
#52694=DIRECTION('ref_axis',(0.,0.924695078163125,0.380708566256253));
#52695=DIRECTION('center_axis',(0.,0.959811515577151,0.280645424985856));
#52696=DIRECTION('ref_axis',(0.193752945248173,0.275327293405562,-0.941623426701793));
#52697=DIRECTION('center_axis',(0.,0.,1.));
#52698=DIRECTION('ref_axis',(1.,0.,0.));
#52699=DIRECTION('center_axis',(0.,0.698552735211551,0.71555857630837));
#52700=DIRECTION('ref_axis',(-0.127350909928658,0.709732301276154,-0.69286492642188));
#52701=DIRECTION('center_axis',(0.,0.280132806031874,-0.959961254939338));
#52702=DIRECTION('ref_axis',(0.,0.959961254939338,0.280132806031874));
#52703=DIRECTION('center_axis',(1.,0.,0.));
#52704=DIRECTION('ref_axis',(0.,0.,-1.));
#52705=DIRECTION('center_axis',(-1.82730824943271E-14,0.691284430421512,
-0.722582753915983));
#52706=DIRECTION('ref_axis',(-1.,9.17044218340399E-12,8.79851747015455E-12));
#52707=DIRECTION('center_axis',(-1.,0.,0.));
#52708=DIRECTION('ref_axis',(0.,0.870686243840935,0.49183886058969));
#52709=DIRECTION('center_axis',(6.01305526018457E-17,-1.15635678080473E-17,
-1.));
#52710=DIRECTION('ref_axis',(-1.,0.,-6.01305526018457E-17));
#52711=DIRECTION('center_axis',(-3.00652763009229E-17,5.78178390402363E-18,
1.));
#52712=DIRECTION('ref_axis',(-1.,0.,-3.00652763009229E-17));
#52713=DIRECTION('center_axis',(3.00652763009229E-17,-5.78178390402363E-18,
-1.));
#52714=DIRECTION('ref_axis',(-1.,0.,-3.00652763009229E-17));
#52715=DIRECTION('center_axis',(0.921947479709923,-0.342317807210713,-0.181194270116276));
#52716=DIRECTION('ref_axis',(-0.127350909928437,-0.709732301276171,0.692864926421903));
#52717=DIRECTION('center_axis',(-0.902368117063134,-0.426637457049683,0.0609283312598752));
#52718=DIRECTION('ref_axis',(0.380530973451334,-0.855128580240046,-0.352067166178307));
#52719=DIRECTION('center_axis',(0.,0.,1.));
#52720=DIRECTION('ref_axis',(1.,0.,0.));
#52721=DIRECTION('center_axis',(0.,-0.380708566256254,0.924695078163125));
#52722=DIRECTION('ref_axis',(0.,-0.924695078163125,-0.380708566256254));
#52723=DIRECTION('center_axis',(0.,-0.959811515577153,-0.280645424985852));
#52724=DIRECTION('ref_axis',(0.193752945248172,-0.275327293405577,0.941623426701788));
#52725=DIRECTION('center_axis',(0.,0.,1.));
#52726=DIRECTION('ref_axis',(1.,0.,0.));
#52727=DIRECTION('center_axis',(0.,-0.698552735211554,-0.715558576308367));
#52728=DIRECTION('ref_axis',(-0.127350909928658,-0.709732301276152,0.692864926421882));
#52729=DIRECTION('center_axis',(0.,-0.280132806031875,0.959961254939338));
#52730=DIRECTION('ref_axis',(0.,-0.959961254939337,-0.280132806031875));
#52731=DIRECTION('center_axis',(1.,0.,0.));
#52732=DIRECTION('ref_axis',(0.,0.,-1.));
#52733=DIRECTION('center_axis',(1.,0.,0.));
#52734=DIRECTION('ref_axis',(0.,-0.866025403784439,-0.5));
#52735=DIRECTION('center_axis',(0.,0.610455145315576,-0.792050828897829));
#52736=DIRECTION('ref_axis',(0.,-0.792050828897829,-0.610455145315577));
#52737=DIRECTION('center_axis',(0.,0.,1.));
#52738=DIRECTION('ref_axis',(1.,0.,0.));
#52739=DIRECTION('center_axis',(-1.,0.,0.));
#52740=DIRECTION('ref_axis',(0.,-0.870686243840935,-0.49183886058969));
#52741=DIRECTION('center_axis',(0.,0.,1.));
#52742=DIRECTION('ref_axis',(-0.999813823611077,-0.0192955465379807,0.));
#52743=DIRECTION('center_axis',(0.,0.968968272584649,0.247185126422123));
#52744=DIRECTION('ref_axis',(-0.12735090992866,-0.245172477034519,0.961078666002477));
#52745=DIRECTION('center_axis',(-0.92194747970986,-0.328077744546277,-0.205858782154334));
#52746=DIRECTION('ref_axis',(-0.127350909928703,-0.245172477034506,0.961078666002475));
#52747=DIRECTION('center_axis',(1.,0.,0.));
#52748=DIRECTION('ref_axis',(0.,0.,-1.));
#52749=DIRECTION('center_axis',(-1.,0.,0.));
#52750=DIRECTION('ref_axis',(0.,0.866025403784439,-0.5));
#52751=DIRECTION('center_axis',(-1.9529598880904E-11,0.270415537393765,
0.962743702724687));
#52752=DIRECTION('ref_axis',(-0.127350909937141,0.954904778303183,-0.268213739603196));
#52753=DIRECTION('center_axis',(0.,0.,1.));
#52754=DIRECTION('ref_axis',(1.,0.,0.));
#52755=DIRECTION('center_axis',(-0.921947479709859,-0.0142400626646423,
0.387053052270546));
#52756=DIRECTION('ref_axis',(-0.127350909928659,0.954904778310657,-0.268213739580614));
#52757=DIRECTION('center_axis',(0.,0.971417236442194,0.237378501012646));
#52758=DIRECTION('ref_axis',(-8.49941231119091E-16,0.237378501012646,-0.971417236442194));
#52759=DIRECTION('center_axis',(0.,-0.270415537373097,0.962743702730493));
#52760=DIRECTION('ref_axis',(-0.127350909928659,0.954904778310663,0.268213739580592));
#52761=DIRECTION('center_axis',(1.,0.,0.));
#52762=DIRECTION('ref_axis',(0.,0.,-1.));
#52763=DIRECTION('center_axis',(-1.,0.,0.));
#52764=DIRECTION('ref_axis',(0.,0.00939817408142913,-0.999955836186746));
#52765=DIRECTION('center_axis',(-1.,0.,0.));
#52766=DIRECTION('ref_axis',(0.,0.00939817408142913,-0.999955836186746));
#52767=DIRECTION('center_axis',(4.04433668405939E-15,-0.971417236442194,
0.237378501012646));
#52768=DIRECTION('ref_axis',(-1.,-4.16333634234424E-15,0.));
#52769=DIRECTION('center_axis',(0.902368117344249,-0.266084211100932,0.339014709715361));
#52770=DIRECTION('ref_axis',(0.193752945248214,0.953133455025081,0.232371282906461));
#52771=DIRECTION('center_axis',(6.01305526018457E-17,-0.866025403784439,
-0.499999999999999));
#52772=DIRECTION('ref_axis',(-1.,-5.20745860967949E-17,-3.00652763009228E-17));
#52773=DIRECTION('center_axis',(-0.90236811705166,-0.266084211227944,0.339014710394468));
#52774=DIRECTION('ref_axis',(0.193752945269933,-0.953133455021166,-0.23237128290441));
#52775=DIRECTION('center_axis',(0.921947479709872,-0.0142400626646524,0.387053052270515));
#52776=DIRECTION('ref_axis',(-0.380530973451301,-0.219520083262134,0.89833574530283));
#52777=DIRECTION('center_axis',(0.,0.,1.));
#52778=DIRECTION('ref_axis',(1.,0.,0.));
#52779=DIRECTION('center_axis',(0.,-0.236859690294948,0.971543867827584));
#52780=DIRECTION('ref_axis',(0.193752945248171,-0.953133455025097,-0.23237128290643));
#52781=DIRECTION('center_axis',(0.,-0.99116371157183,-0.132644249265295));
#52782=DIRECTION('ref_axis',(0.,-0.132644249265295,0.99116371157183));
#52783=DIRECTION('center_axis',(1.,0.,0.));
#52784=DIRECTION('ref_axis',(0.,7.6571373978539E-16,1.));
#52785=DIRECTION('center_axis',(-1.72745658077656E-15,0.97141723644226,
0.237378501012378));
#52786=DIRECTION('ref_axis',(-1.,-3.0267455208844E-12,1.23789867245708E-11));
#52787=DIRECTION('center_axis',(-1.,0.,0.));
#52788=DIRECTION('ref_axis',(0.,-1.25707743249494E-14,1.));
#52789=DIRECTION('center_axis',(-1.,0.,0.));
#52790=DIRECTION('ref_axis',(0.,-1.25707743249494E-14,1.));
#52791=DIRECTION('center_axis',(1.43479105966359E-11,-0.971417236440792,
0.237378501018383));
#52792=DIRECTION('ref_axis',(-0.380530973451296,0.219520083262137,0.898335745302831));
#52793=DIRECTION('center_axis',(0.,0.,1.));
#52794=DIRECTION('ref_axis',(-0.75239437642935,0.65871291342852,0.));
#52795=DIRECTION('center_axis',(-0.92194747970986,-0.0142400626646407,-0.387053052270545));
#52796=DIRECTION('ref_axis',(-0.127350909928659,0.95490477831066,0.268213739580603));
#52797=DIRECTION('center_axis',(0.,0.,1.));
#52798=DIRECTION('ref_axis',(1.,0.,0.));
#52799=DIRECTION('center_axis',(0.,0.270415537373098,0.962743702730492));
#52800=DIRECTION('ref_axis',(-0.127350909928659,-0.954904778310663,0.268213739580592));
#52801=DIRECTION('center_axis',(1.,0.,0.));
#52802=DIRECTION('ref_axis',(0.,-1.01374804525729E-13,1.));
#52803=DIRECTION('center_axis',(1.3755159672E-15,0.991163711571829,-0.1326442492653));
#52804=DIRECTION('ref_axis',(0.380530973451305,0.122665180371209,0.916596657079165));
#52805=DIRECTION('center_axis',(1.,0.,0.));
#52806=DIRECTION('ref_axis',(0.,-0.0101818638820796,0.999948163480431));
#52807=DIRECTION('center_axis',(6.01305526018457E-17,0.866025403784439,
0.5));
#52808=DIRECTION('ref_axis',(-1.,5.20745860967949E-17,3.00652763009229E-17));
#52809=DIRECTION('center_axis',(0.,-0.968968272584649,0.247185126422125));
#52810=DIRECTION('ref_axis',(-0.127350909928658,0.245172477034511,0.961078666002479));
#52811=DIRECTION('center_axis',(0.921947479709867,-0.328077744546277,0.205858782154301));
#52812=DIRECTION('ref_axis',(-0.127350909928615,0.245172477034512,0.961078666002484));
#52813=DIRECTION('center_axis',(-0.902368117063139,-0.160553245843629,0.399943041640932));
#52814=DIRECTION('ref_axis',(0.380530973451339,-0.732463399868841,0.564529490900833));
#52815=DIRECTION('center_axis',(0.,0.,1.));
#52816=DIRECTION('ref_axis',(1.,0.,0.));
#52817=DIRECTION('center_axis',(0.,0.610455145315577,0.792050828897829));
#52818=DIRECTION('ref_axis',(0.,-0.792050828897829,0.610455145315577));
#52819=DIRECTION('center_axis',(0.,-0.722951825282204,0.690898442841732));
#52820=DIRECTION('ref_axis',(0.193752945248174,0.67780616161952,0.70925214379533));
#52821=DIRECTION('center_axis',(0.,0.,1.));
#52822=DIRECTION('ref_axis',(-0.999813823611077,0.0192955465379763,0.));
#52823=DIRECTION('center_axis',(0.,0.691284430410319,0.722582753926691));
#52824=DIRECTION('ref_axis',(0.,-0.722582753926691,0.691284430410319));
#52825=DIRECTION('center_axis',(1.,0.,0.));
#52826=DIRECTION('ref_axis',(0.,0.,-1.));
#52827=DIRECTION('center_axis',(1.,0.,0.));
#52828=DIRECTION('ref_axis',(0.,-0.866025403784438,0.500000000000001));
#52829=DIRECTION('center_axis',(0.,0.,1.));
#52830=DIRECTION('ref_axis',(1.,0.,0.));
#52831=DIRECTION('center_axis',(-1.,0.,0.));
#52832=DIRECTION('ref_axis',(0.,-0.866025403784438,0.500000000000001));
#52833=DIRECTION('center_axis',(1.,0.,0.));
#52834=DIRECTION('ref_axis',(0.,0.,-1.));
#52835=DIRECTION('center_axis',(1.,0.,0.));
#52836=DIRECTION('ref_axis',(0.,0.,-1.));
#52837=DIRECTION('center_axis',(-2.99590214590677E-14,-0.691284430421536,
0.72258275391596));
#52838=DIRECTION('ref_axis',(-1.,-9.15933995315774E-12,-8.80406858527768E-12));
#52839=DIRECTION('center_axis',(0.,0.,1.));
#52840=DIRECTION('ref_axis',(-0.999813823611077,0.0192955465379763,0.));
#52841=DIRECTION('center_axis',(0.,-0.968968272584649,-0.247185126422125));
#52842=DIRECTION('ref_axis',(-0.127350909928658,0.245172477034511,-0.961078666002479));
#52843=DIRECTION('center_axis',(-0.921947479709859,0.328077744546278,0.205858782154336));
#52844=DIRECTION('ref_axis',(-0.127350909928746,0.245172477034532,-0.961078666002462));
#52845=DIRECTION('center_axis',(6.01305526018457E-17,1.34028247722783E-16,
1.));
#52846=DIRECTION('ref_axis',(-1.,0.,6.01305526018457E-17));
#52847=DIRECTION('center_axis',(0.,0.,1.));
#52848=DIRECTION('ref_axis',(1.,0.,0.));
#52849=DIRECTION('center_axis',(6.57417704427592E-16,0.236859690294945,
-0.971543867827585));
#52850=DIRECTION('ref_axis',(1.,-2.77555756156295E-15,0.));
#52851=DIRECTION('center_axis',(2.64693773984223E-10,0.991163711556711,
0.132644249378273));
#52852=DIRECTION('ref_axis',(0.38053097345134,0.122665180375841,-0.916596657078531));
#52853=DIRECTION('center_axis',(0.,0.,1.));
#52854=DIRECTION('ref_axis',(1.,0.,0.));
#52855=DIRECTION('center_axis',(0.,-0.991163711571829,0.132644249265303));
#52856=DIRECTION('ref_axis',(0.380530973451305,-0.12266518037121,-0.916596657079165));
#52857=DIRECTION('center_axis',(0.,-0.236859690294949,-0.971543867827584));
#52858=DIRECTION('ref_axis',(0.193752945248173,-0.953133455025086,0.232371282906476));
#52859=DIRECTION('center_axis',(0.902368117063139,0.266084211206075,0.339014710381078));
#52860=DIRECTION('ref_axis',(0.193752945248083,-0.953133455025115,0.232371282906431));
#52861=DIRECTION('center_axis',(1.,0.,0.));
#52862=DIRECTION('ref_axis',(0.,0.,-1.));
#52863=DIRECTION('center_axis',(1.,0.,0.));
#52864=DIRECTION('ref_axis',(0.,0.0101818638820808,-0.999948163480431));
#52865=DIRECTION('center_axis',(0.,0.,1.));
#52866=DIRECTION('ref_axis',(-0.752394376425733,0.658712913432652,0.));
#52867=DIRECTION('center_axis',(-0.92194747970986,0.0142400626646414,0.387053052270544));
#52868=DIRECTION('ref_axis',(-0.127350909928614,-0.954904778310663,-0.268213739580614));
#52869=DIRECTION('center_axis',(0.,0.270415537373095,-0.962743702730493));
#52870=DIRECTION('ref_axis',(-0.127350909928658,-0.954904778310661,-0.268213739580602));
#52871=DIRECTION('center_axis',(-0.90236811706313,-0.160553245843604,-0.399943041640962));
#52872=DIRECTION('ref_axis',(0.193752945248216,0.677806161619511,-0.709252143795327));
#52873=DIRECTION('center_axis',(0.,0.,1.));
#52874=DIRECTION('ref_axis',(1.,0.,0.));
#52875=DIRECTION('center_axis',(0.,-0.722951825282205,-0.690898442841731));
#52876=DIRECTION('ref_axis',(0.193752945248172,0.677806161619523,-0.709252143795327));
#52877=DIRECTION('center_axis',(1.,0.,0.));
#52878=DIRECTION('ref_axis',(0.,1.,0.));
#52879=DIRECTION('',(-1.,0.,0.));
#52880=DIRECTION('center_axis',(0.,0.,1.));
#52881=DIRECTION('ref_axis',(1.,0.,0.));
#52882=DIRECTION('center_axis',(1.22464679914735E-16,-1.,0.));
#52883=DIRECTION('ref_axis',(-1.,-1.22464679914735E-16,0.));
#52884=DIRECTION('center_axis',(6.01305526018457E-17,-0.866025403784438,
0.5));
#52885=DIRECTION('ref_axis',(-1.,-5.20745860967949E-17,3.00652763009229E-17));
#52886=DIRECTION('center_axis',(0.,0.,1.));
#52887=DIRECTION('ref_axis',(1.,0.,0.));
#52888=DIRECTION('center_axis',(0.,0.236859690294946,0.971543867827584));
#52889=DIRECTION('ref_axis',(0.193752945248173,0.953133455025083,-0.232371282906487));
#52890=DIRECTION('center_axis',(0.902368117063138,-0.266084211206076,-0.33901471038108));
#52891=DIRECTION('ref_axis',(0.193752945248217,0.953133455025082,-0.232371282906453));
#52892=DIRECTION('center_axis',(0.,0.,1.));
#52893=DIRECTION('ref_axis',(1.,0.,0.));
#52894=DIRECTION('center_axis',(1.22464679914735E-16,-1.,0.));
#52895=DIRECTION('ref_axis',(-1.,-1.22464679914735E-16,0.));
#52896=DIRECTION('center_axis',(-0.902368117063139,0.160553245843631,0.399943041640932));
#52897=DIRECTION('ref_axis',(0.193752945248174,-0.677806161619514,0.709252143795335));
#52898=DIRECTION('center_axis',(0.,0.,1.));
#52899=DIRECTION('ref_axis',(1.,0.,0.));
#52900=DIRECTION('center_axis',(0.,0.722951825282206,0.690898442841729));
#52901=DIRECTION('ref_axis',(0.193752945248172,-0.677806161619518,0.709252143795333));
#52902=DIRECTION('center_axis',(0.,-0.610455145315576,0.79205082889783));
#52903=DIRECTION('ref_axis',(0.,0.79205082889783,0.610455145315576));
#52904=DIRECTION('center_axis',(1.,0.,0.));
#52905=DIRECTION('ref_axis',(0.,1.,0.));
#52906=DIRECTION('',(-1.,0.,0.));
#52907=DIRECTION('',(1.,0.,0.));
#52908=DIRECTION('center_axis',(1.,0.,0.));
#52909=DIRECTION('ref_axis',(0.,0.,-1.));
#52910=DIRECTION('center_axis',(1.,0.,0.));
#52911=DIRECTION('ref_axis',(0.,0.866025403784439,0.5));
#52912=DIRECTION('center_axis',(6.01305526018457E-17,0.866025403784439,
-0.5));
#52913=DIRECTION('ref_axis',(-1.,5.20745860967949E-17,-3.00652763009229E-17));
#52914=DIRECTION('center_axis',(-3.00652763009229E-17,-0.866025403784439,
0.5));
#52915=DIRECTION('ref_axis',(-1.,0.,-6.01305526018457E-17));
#52916=DIRECTION('center_axis',(3.00652763009229E-17,0.866025403784439,
-0.5));
#52917=DIRECTION('ref_axis',(-1.,0.,-6.01305526018457E-17));
#52918=DIRECTION('center_axis',(0.,0.,1.));
#52919=DIRECTION('ref_axis',(1.,0.,0.));
#52920=DIRECTION('center_axis',(1.,0.,0.));
#52921=DIRECTION('ref_axis',(0.,0.,-1.));
#52922=DIRECTION('center_axis',(1.,0.,0.));
#52923=DIRECTION('ref_axis',(0.,0.866025403784439,-0.5));
#52924=DIRECTION('center_axis',(0.,0.,1.));
#52925=DIRECTION('ref_axis',(1.,0.,0.));
#52926=DIRECTION('center_axis',(1.,0.,0.));
#52927=DIRECTION('ref_axis',(0.,-0.866025403784437,-0.500000000000003));
#52928=DIRECTION('',(-1.,0.,0.));
#52929=DIRECTION('',(1.,0.,0.));
#52930=DIRECTION('center_axis',(0.,-0.965925826289068,0.258819045102522));
#52931=DIRECTION('ref_axis',(0.,-0.258819045102522,-0.965925826289068));
#52932=DIRECTION('',(1.,0.,0.));
#52933=DIRECTION('center_axis',(1.,0.,0.));
#52934=DIRECTION('ref_axis',(0.,-0.499999999999996,0.866025403784441));
#52935=DIRECTION('',(-1.,0.,0.));
#52936=DIRECTION('center_axis',(0.,0.258819045102522,0.965925826289068));
#52937=DIRECTION('ref_axis',(0.,-0.965925826289068,0.258819045102522));
#52938=DIRECTION('',(1.,0.,0.));
#52939=DIRECTION('center_axis',(0.,-0.258819045102522,-0.965925826289068));
#52940=DIRECTION('ref_axis',(0.,0.965925826289068,-0.258819045102522));
#52941=DIRECTION('',(-1.,0.,0.));
#52942=DIRECTION('center_axis',(1.,0.,0.));
#52943=DIRECTION('ref_axis',(0.,1.,0.));
#52944=DIRECTION('center_axis',(0.,-0.866025403784438,0.5));
#52945=DIRECTION('ref_axis',(0.,-0.5,-0.866025403784438));
#52946=DIRECTION('center_axis',(1.,0.,0.));
#52947=DIRECTION('ref_axis',(0.,1.,0.));
#52948=DIRECTION('',(-1.,0.,0.));
#52949=DIRECTION('center_axis',(1.,0.,0.));
#52950=DIRECTION('ref_axis',(0.,1.,0.));
#52951=DIRECTION('',(1.,0.,0.));
#52952=DIRECTION('center_axis',(0.,-0.707106781186548,-0.707106781186547));
#52953=DIRECTION('ref_axis',(0.,0.707106781186547,-0.707106781186548));
#52954=DIRECTION('',(-1.,0.,0.));
#52955=DIRECTION('center_axis',(0.,0.707106781186548,0.707106781186547));
#52956=DIRECTION('ref_axis',(0.,-0.707106781186547,0.707106781186548));
#52957=DIRECTION('center_axis',(0.,0.499999999999999,-0.866025403784439));
#52958=DIRECTION('ref_axis',(0.,0.866025403784439,0.499999999999999));
#52959=DIRECTION('center_axis',(0.,-0.499999999999999,0.866025403784439));
#52960=DIRECTION('ref_axis',(0.,-0.866025403784439,-0.499999999999999));
#52961=DIRECTION('center_axis',(1.,0.,0.));
#52962=DIRECTION('ref_axis',(0.,1.,0.));
#52963=DIRECTION('center_axis',(0.,-0.25881904510252,0.965925826289068));
#52964=DIRECTION('ref_axis',(0.,-0.965925826289068,-0.25881904510252));
#52965=DIRECTION('center_axis',(1.,0.,0.));
#52966=DIRECTION('ref_axis',(0.,1.,0.));
#52967=DIRECTION('center_axis',(0.,1.83697019872103E-16,1.));
#52968=DIRECTION('ref_axis',(0.,-1.,1.83697019872103E-16));
#52969=DIRECTION('center_axis',(1.,0.,0.));
#52970=DIRECTION('ref_axis',(0.,1.,0.));
#52971=DIRECTION('center_axis',(1.,0.,0.));
#52972=DIRECTION('ref_axis',(0.,1.,0.));
#52973=DIRECTION('',(1.,0.,0.));
#52974=DIRECTION('center_axis',(0.,-0.965925826289068,0.258819045102522));
#52975=DIRECTION('ref_axis',(0.,-0.258819045102522,-0.965925826289068));
#52976=DIRECTION('center_axis',(0.,0.965925826289068,-0.258819045102522));
#52977=DIRECTION('ref_axis',(0.,0.258819045102522,0.965925826289068));
#52978=DIRECTION('center_axis',(0.,-0.5,-0.866025403784438));
#52979=DIRECTION('ref_axis',(0.,0.866025403784438,-0.5));
#52980=DIRECTION('center_axis',(0.,0.5,0.866025403784438));
#52981=DIRECTION('ref_axis',(0.,-0.866025403784438,0.5));
#52982=DIRECTION('center_axis',(1.,0.,0.));
#52983=DIRECTION('ref_axis',(0.,1.,0.));
#52984=DIRECTION('center_axis',(0.,0.707106781186548,0.707106781186547));
#52985=DIRECTION('ref_axis',(0.,-0.707106781186547,0.707106781186548));
#52986=DIRECTION('center_axis',(1.,0.,0.));
#52987=DIRECTION('ref_axis',(0.,1.,0.));
#52988=DIRECTION('center_axis',(0.,0.866025403784439,0.5));
#52989=DIRECTION('ref_axis',(0.,-0.5,0.866025403784439));
#52990=DIRECTION('center_axis',(1.,0.,0.));
#52991=DIRECTION('ref_axis',(0.,1.,0.));
#52992=DIRECTION('',(1.,0.,0.));
#52993=DIRECTION('center_axis',(0.,-0.25881904510252,0.965925826289068));
#52994=DIRECTION('ref_axis',(0.,-0.965925826289068,-0.25881904510252));
#52995=DIRECTION('',(-1.,0.,0.));
#52996=DIRECTION('center_axis',(0.,0.25881904510252,-0.965925826289068));
#52997=DIRECTION('ref_axis',(0.,0.965925826289068,0.25881904510252));
#52998=DIRECTION('center_axis',(0.,-1.,1.22464679914735E-16));
#52999=DIRECTION('ref_axis',(0.,-1.22464679914735E-16,-1.));
#53000=DIRECTION('center_axis',(0.,1.,-1.22464679914735E-16));
#53001=DIRECTION('ref_axis',(0.,1.22464679914735E-16,1.));
#53002=DIRECTION('center_axis',(1.,0.,0.));
#53003=DIRECTION('ref_axis',(0.,1.,0.));
#53004=DIRECTION('center_axis',(0.,0.965925826289068,-0.258819045102521));
#53005=DIRECTION('ref_axis',(0.,0.258819045102521,0.965925826289068));
#53006=DIRECTION('center_axis',(1.,0.,0.));
#53007=DIRECTION('ref_axis',(0.,1.,0.));
#53008=DIRECTION('center_axis',(0.,0.866025403784438,-0.5));
#53009=DIRECTION('ref_axis',(0.,0.5,0.866025403784438));
#53010=DIRECTION('center_axis',(1.,0.,0.));
#53011=DIRECTION('ref_axis',(0.,1.,0.));
#53012=DIRECTION('center_axis',(1.,0.,0.));
#53013=DIRECTION('ref_axis',(0.,1.,0.));
#53014=DIRECTION('',(1.,0.,0.));
#53015=DIRECTION('center_axis',(0.,0.707106781186548,0.707106781186547));
#53016=DIRECTION('ref_axis',(0.,-0.707106781186547,0.707106781186548));
#53017=DIRECTION('',(-1.,0.,0.));
#53018=DIRECTION('center_axis',(0.,-0.707106781186548,-0.707106781186547));
#53019=DIRECTION('ref_axis',(0.,0.707106781186547,-0.707106781186548));
#53020=DIRECTION('center_axis',(0.,-0.5,0.866025403784439));
#53021=DIRECTION('ref_axis',(0.,-0.866025403784439,-0.5));
#53022=DIRECTION('center_axis',(0.,0.5,-0.866025403784439));
#53023=DIRECTION('ref_axis',(0.,0.866025403784439,0.5));
#53024=DIRECTION('center_axis',(1.,0.,0.));
#53025=DIRECTION('ref_axis',(0.,1.,0.));
#53026=DIRECTION('center_axis',(0.,0.258819045102521,-0.965925826289068));
#53027=DIRECTION('ref_axis',(0.,0.965925826289068,0.258819045102521));
#53028=DIRECTION('center_axis',(1.,0.,0.));
#53029=DIRECTION('ref_axis',(0.,1.,0.));
#53030=DIRECTION('center_axis',(0.,-6.12323399573677E-17,-1.));
#53031=DIRECTION('ref_axis',(0.,1.,-6.12323399573677E-17));
#53032=DIRECTION('center_axis',(1.,0.,0.));
#53033=DIRECTION('ref_axis',(0.,1.,0.));
#53034=DIRECTION('center_axis',(1.,0.,0.));
#53035=DIRECTION('ref_axis',(0.,1.,0.));
#53036=DIRECTION('',(1.,0.,0.));
#53037=DIRECTION('center_axis',(0.,0.965925826289068,-0.258819045102521));
#53038=DIRECTION('ref_axis',(0.,0.258819045102521,0.965925826289068));
#53039=DIRECTION('center_axis',(0.,-0.965925826289068,0.258819045102521));
#53040=DIRECTION('ref_axis',(0.,-0.258819045102521,-0.965925826289068));
#53041=DIRECTION('center_axis',(0.,0.5,0.866025403784439));
#53042=DIRECTION('ref_axis',(0.,-0.866025403784439,0.5));
#53043=DIRECTION('',(1.,0.,0.));
#53044=DIRECTION('',(1.,0.,0.));
#53045=DIRECTION('center_axis',(0.,0.866025403784439,-0.5));
#53046=DIRECTION('ref_axis',(0.,0.5,0.866025403784439));
#53047=DIRECTION('',(-1.,0.,0.));
#53048=DIRECTION('center_axis',(0.,-0.866025403784439,0.5));
#53049=DIRECTION('ref_axis',(0.,-0.5,-0.866025403784439));
#53050=DIRECTION('center_axis',(1.,0.,0.));
#53051=DIRECTION('ref_axis',(0.,1.,0.));
#53052=DIRECTION('',(1.,0.,0.));
#53053=DIRECTION('center_axis',(0.,0.707106781186548,-0.707106781186548));
#53054=DIRECTION('ref_axis',(0.,0.707106781186548,0.707106781186548));
#53055=DIRECTION('',(-1.,0.,0.));
#53056=DIRECTION('center_axis',(0.,-0.707106781186548,0.707106781186548));
#53057=DIRECTION('ref_axis',(0.,-0.707106781186548,-0.707106781186548));
#53058=DIRECTION('center_axis',(0.,-0.5,0.866025403784439));
#53059=DIRECTION('ref_axis',(0.,-0.866025403784439,-0.5));
#53060=DIRECTION('',(1.,0.,0.));
#53061=DIRECTION('center_axis',(0.,0.5,-0.866025403784439));
#53062=DIRECTION('ref_axis',(0.,0.866025403784439,0.5));
#53063=DIRECTION('',(-1.,0.,0.));
#53064=DIRECTION('center_axis',(1.,0.,0.));
#53065=DIRECTION('ref_axis',(0.,1.,0.));
#53066=DIRECTION('center_axis',(0.,-0.965925826289068,-0.258819045102521));
#53067=DIRECTION('ref_axis',(0.,0.258819045102521,-0.965925826289068));
#53068=DIRECTION('center_axis',(1.,0.,0.));
#53069=DIRECTION('ref_axis',(0.,1.,0.));
#53070=DIRECTION('center_axis',(1.,0.,0.));
#53071=DIRECTION('ref_axis',(0.,1.,0.));
#53072=DIRECTION('',(1.,0.,0.));
#53073=DIRECTION('center_axis',(0.,0.,-1.));
#53074=DIRECTION('ref_axis',(0.,1.,0.));
#53075=DIRECTION('',(1.,0.,0.));
#53076=DIRECTION('center_axis',(0.,1.,0.));
#53077=DIRECTION('ref_axis',(0.,0.,1.));
#53078=DIRECTION('',(1.,0.,0.));
#53079=DIRECTION('center_axis',(0.,0.,1.));
#53080=DIRECTION('ref_axis',(0.,-1.,0.));
#78381=CARTESIAN_POINT('',(0.,0.,0.));
#78382=CARTESIAN_POINT('Origin',(141.,11.5,0.3));
#78383=CARTESIAN_POINT('',(159.,11.1,0.3));
#78384=CARTESIAN_POINT('',(159.,11.5,0.7));
#78385=CARTESIAN_POINT('Origin',(159.,11.5,0.3));
#78386=CARTESIAN_POINT('',(141.,11.5,0.7));
#78387=CARTESIAN_POINT('',(141.,11.5,0.7));
#78388=CARTESIAN_POINT('',(141.,11.1,0.3));
#78389=CARTESIAN_POINT('Origin',(141.,11.5,0.3));
#78390=CARTESIAN_POINT('',(141.,11.1,0.3));
#78391=CARTESIAN_POINT('Origin',(159.,12.,0.));
#78392=CARTESIAN_POINT('',(159.,11.1,-0.3));
#78393=CARTESIAN_POINT('',(159.,11.1,0.7));
#78394=CARTESIAN_POINT('',(159.,11.5,-0.7));
#78395=CARTESIAN_POINT('Origin',(159.,11.5,-0.3));
#78396=CARTESIAN_POINT('',(159.,12.4,-0.7));
#78397=CARTESIAN_POINT('',(159.,11.1,-0.7));
#78398=CARTESIAN_POINT('',(159.,12.4,0.7));
#78399=CARTESIAN_POINT('',(159.,12.4,-0.7));
#78400=CARTESIAN_POINT('',(159.,12.2,0.7));
#78401=CARTESIAN_POINT('Origin',(141.,11.1,0.7));
#78402=CARTESIAN_POINT('',(141.,11.1,-0.3));
#78403=CARTESIAN_POINT('',(141.,11.1,0.7));
#78404=CARTESIAN_POINT('',(141.,11.1,-0.3));
#78405=CARTESIAN_POINT('Origin',(141.,11.5,-0.3));
#78406=CARTESIAN_POINT('',(141.,11.5,-0.7));
#78407=CARTESIAN_POINT('Origin',(141.,11.5,-0.3));
#78408=CARTESIAN_POINT('',(141.,11.5,-0.7));
#78409=CARTESIAN_POINT('Origin',(141.,11.185792715855,2.68664127079227));
#78410=CARTESIAN_POINT('',(159.,11.289320333896,2.30027094027664));
#78411=CARTESIAN_POINT('',(159.,10.7994223853394,2.58311365275126));
#78412=CARTESIAN_POINT('Origin',(159.,11.185792715855,2.68664127079227));
#78413=CARTESIAN_POINT('',(141.,10.7994223853394,2.58311365275126));
#78414=CARTESIAN_POINT('',(141.,10.7994223853394,2.58311365275126));
#78415=CARTESIAN_POINT('',(141.,11.289320333896,2.30027094027664));
#78416=CARTESIAN_POINT('Origin',(141.,11.185792715855,2.68664127079227));
#78417=CARTESIAN_POINT('',(141.,11.289320333896,2.30027094027664));
#78418=CARTESIAN_POINT('Origin',(141.,10.9029500033804,2.19674332223563));
#78419=CARTESIAN_POINT('',(141.,11.7525454562834,2.42439173773413));
#78420=CARTESIAN_POINT('',(141.,10.9029500033804,2.19674332223563));
#78421=CARTESIAN_POINT('',(159.,11.7525454562834,2.42439173773413));
#78422=CARTESIAN_POINT('',(150.,11.7525454562834,2.42439173773413));
#78423=CARTESIAN_POINT('',(159.,10.9029500033804,2.19674332223563));
#78424=CARTESIAN_POINT('Origin',(141.,21.1660104885167,0.));
#78425=CARTESIAN_POINT('',(141.,20.0629605711151,5.85470862826488));
#78426=CARTESIAN_POINT('',(141.,15.1018066893986,14.4476792155782));
#78427=CARTESIAN_POINT('Origin',(141.,-1.33226762955019E-14,0.));
#78428=CARTESIAN_POINT('',(141.,20.0629605711151,-5.8547086282649));
#78429=CARTESIAN_POINT('Ctrl Pts',(141.,20.0629999218784,-5.85467024331719));
#78430=CARTESIAN_POINT('Ctrl Pts',(141.,19.2430532730423,-5.01409266439642));
#78431=CARTESIAN_POINT('Ctrl Pts',(141.,17.9072203962775,-2.91890983500256));
#78432=CARTESIAN_POINT('Ctrl Pts',(141.,17.325103889108,1.48733530859094));
#78433=CARTESIAN_POINT('Ctrl Pts',(141.,18.7423719290453,4.50197105960825));
#78434=CARTESIAN_POINT('Ctrl Pts',(141.,20.0629605711151,5.8547086282649));
#78435=CARTESIAN_POINT('',(141.,15.1018066893909,-14.4476792155788));
#78436=CARTESIAN_POINT('Origin',(141.,-1.33226762955019E-14,0.));
#78437=CARTESIAN_POINT('',(141.,4.96115388173191,-20.3023878438326));
#78438=CARTESIAN_POINT('Ctrl Pts',(141.,4.96115388172977,-20.3023878438239));
#78439=CARTESIAN_POINT('Ctrl Pts',(141.,5.30196057289897,-19.0890348724825));
#78440=CARTESIAN_POINT('Ctrl Pts',(141.,6.52826244821434,-16.8178412826011));
#78441=CARTESIAN_POINT('Ctrl Pts',(141.,10.1360629310422,-14.2220750860635));
#78442=CARTESIAN_POINT('Ctrl Pts',(141.,13.3527862418892,-14.0038442289584));
#78443=CARTESIAN_POINT('Ctrl Pts',(141.,15.1017679586878,-14.4478317858267));
#78444=CARTESIAN_POINT('',(141.,-4.96115388172423,-20.3023878438437));
#78445=CARTESIAN_POINT('Origin',(141.,-1.33226762955019E-14,0.));
#78446=CARTESIAN_POINT('',(141.,-15.1018066893986,-14.4476792155782));
#78447=CARTESIAN_POINT('Ctrl Pts',(141.,-15.101806689398,-14.4476792155806));
#78448=CARTESIAN_POINT('Ctrl Pts',(141.,-13.9043899707631,-14.1422165793404));
#78449=CARTESIAN_POINT('Ctrl Pts',(141.,-11.3772954300591,-14.0593422845693));
#78450=CARTESIAN_POINT('Ctrl Pts',(141.,-7.30575619982706,-15.8297568135614));
#78451=CARTESIAN_POINT('Ctrl Pts',(141.,-5.46240877807713,-18.5178010570987));
#78452=CARTESIAN_POINT('Ctrl Pts',(141.,-4.96115388172423,-20.3023878438437));
#78453=CARTESIAN_POINT('',(141.,-20.0629605711152,-5.85470862826491));
#78454=CARTESIAN_POINT('Origin',(141.,-1.33226762955019E-14,0.));
#78455=CARTESIAN_POINT('',(141.,-20.0629605711152,5.85470862826493));
#78456=CARTESIAN_POINT('Ctrl Pts',(141.,-20.0630732716319,5.85459886340055));
#78457=CARTESIAN_POINT('Ctrl Pts',(141.,-18.8040685238622,4.56192213590864));
#78458=CARTESIAN_POINT('Ctrl Pts',(141.,-17.3846996032413,1.66705330562719));
#78459=CARTESIAN_POINT('Ctrl Pts',(141.,-17.8288251260465,-2.75531450942628));
#78460=CARTESIAN_POINT('Ctrl Pts',(141.,-19.1825681430686,-4.95288358249382));
#78461=CARTESIAN_POINT('Ctrl Pts',(141.,-20.0629605711152,-5.85470862826492));
#78462=CARTESIAN_POINT('',(141.,-15.1018066893909,14.4476792155788));
#78463=CARTESIAN_POINT('Origin',(141.,-1.33226762955019E-14,0.));
#78464=CARTESIAN_POINT('',(141.,-4.96115388171984,20.3023878438501));
#78465=CARTESIAN_POINT('Ctrl Pts',(141.,-4.96115388172225,20.3023878438507));
#78466=CARTESIAN_POINT('Ctrl Pts',(141.,-5.29532381288502,19.1126633184215));
#78467=CARTESIAN_POINT('Ctrl Pts',(141.,-6.48710099582796,16.8826952544151));
#78468=CARTESIAN_POINT('Ctrl Pts',(141.,-10.0560944361583,14.2418489097857));
#78469=CARTESIAN_POINT('Ctrl Pts',(141.,-13.3056816013333,13.9894852586423));
#78470=CARTESIAN_POINT('Ctrl Pts',(141.,-15.1018066893909,14.4476792155788));
#78471=CARTESIAN_POINT('',(141.,4.96115388171986,20.30238784385));
#78472=CARTESIAN_POINT('Origin',(141.,-1.33226762955019E-14,0.));
#78473=CARTESIAN_POINT('Ctrl Pts',(141.,15.1018066893979,14.4476792155806));
#78474=CARTESIAN_POINT('Ctrl Pts',(141.,13.9043899707623,14.1422165793403));
#78475=CARTESIAN_POINT('Ctrl Pts',(141.,11.3772954300569,14.0593422845694));
#78476=CARTESIAN_POINT('Ctrl Pts',(141.,7.30575619982316,15.829756813564));
#78477=CARTESIAN_POINT('Ctrl Pts',(141.,5.46240877807393,18.5178010571043));
#78478=CARTESIAN_POINT('Ctrl Pts',(141.,4.96115388172226,20.3023878438507));
#78479=CARTESIAN_POINT('',(141.,11.9795659353751,0.7));
#78480=CARTESIAN_POINT('',(141.,12.4,0.7));
#78481=CARTESIAN_POINT('Origin',(141.,0.,0.));
#78482=CARTESIAN_POINT('',(141.,10.6441309582779,3.1626691485247));
#78483=CARTESIAN_POINT('',(141.,10.5406033402369,3.54903947904033));
#78484=CARTESIAN_POINT('',(141.,10.9269736707525,3.65256709708134));
#78485=CARTESIAN_POINT('Origin',(141.,11.0305012887935,3.26619676656571));
#78486=CARTESIAN_POINT('',(141.,11.3901987931398,3.77668789453882));
#78487=CARTESIAN_POINT('',(141.,11.7963069144127,3.8855042376736));
#78488=CARTESIAN_POINT('',(141.,10.7246084263455,5.38356518503845));
#78489=CARTESIAN_POINT('Origin',(141.,0.,0.));
#78490=CARTESIAN_POINT('',(141.,10.309292143521,5.14378221735089));
#78491=CARTESIAN_POINT('',(141.,9.96288198200727,4.94378221735089));
#78492=CARTESIAN_POINT('',(141.,9.76288198200727,5.29019237886467));
#78493=CARTESIAN_POINT('Origin',(141.,10.109292143521,5.49019237886467));
#78494=CARTESIAN_POINT('',(141.,9.46288198200727,5.80980762113533));
#78495=CARTESIAN_POINT('',(141.,9.26288198200727,6.1562177826491));
#78496=CARTESIAN_POINT('',(141.,9.60929214352104,6.35621778264911));
#78497=CARTESIAN_POINT('Origin',(141.,9.80929214352104,6.00980762113533));
#78498=CARTESIAN_POINT('',(141.,10.0246084263455,6.59600075033667));
#78499=CARTESIAN_POINT('',(141.,10.388715006927,6.80621778264911));
#78500=CARTESIAN_POINT('',(141.,8.9658070554057,7.97585756174453));
#78501=CARTESIAN_POINT('Origin',(141.,0.,0.));
#78502=CARTESIAN_POINT('',(141.,8.62670273047588,7.63675323681471));
#78503=CARTESIAN_POINT('',(141.,8.34386001800126,7.35391052434009));
#78504=CARTESIAN_POINT('',(141.,8.06101730552664,7.63675323681471));
#78505=CARTESIAN_POINT('Origin',(141.,8.34386001800126,7.91959594928933));
#78506=CARTESIAN_POINT('',(141.,7.63675323681471,8.06101730552664));
#78507=CARTESIAN_POINT('',(141.,7.35391052434009,8.34386001800126));
#78508=CARTESIAN_POINT('',(141.,7.63675323681471,8.62670273047588));
#78509=CARTESIAN_POINT('Origin',(141.,7.91959594928933,8.34386001800126));
#78510=CARTESIAN_POINT('',(141.,7.97585756174453,8.9658070554057));
#78511=CARTESIAN_POINT('',(141.,8.27314933988261,9.26309883354377));
#78512=CARTESIAN_POINT('',(141.,6.59600075033667,10.0246084263455));
#78513=CARTESIAN_POINT('Origin',(141.,0.,0.));
#78514=CARTESIAN_POINT('',(141.,6.35621778264911,9.60929214352104));
#78515=CARTESIAN_POINT('',(141.,6.15621778264911,9.26288198200727));
#78516=CARTESIAN_POINT('',(141.,5.80980762113533,9.46288198200727));
#78517=CARTESIAN_POINT('Origin',(141.,6.00980762113533,9.80929214352104));
#78518=CARTESIAN_POINT('',(141.,5.29019237886467,9.76288198200727));
#78519=CARTESIAN_POINT('',(141.,4.94378221735089,9.96288198200727));
#78520=CARTESIAN_POINT('',(141.,5.14378221735089,10.309292143521));
#78521=CARTESIAN_POINT('Origin',(141.,5.49019237886467,10.109292143521));
#78522=CARTESIAN_POINT('',(141.,5.38356518503846,10.7246084263455));
#78523=CARTESIAN_POINT('',(141.,5.59378221735089,11.088715006927));
#78524=CARTESIAN_POINT('',(141.,3.77668789453883,11.3901987931398));
#78525=CARTESIAN_POINT('Origin',(141.,0.,0.));
#78526=CARTESIAN_POINT('',(141.,3.65256709708134,10.9269736707525));
#78527=CARTESIAN_POINT('',(141.,3.54903947904033,10.5406033402369));
#78528=CARTESIAN_POINT('',(141.,3.1626691485247,10.6441309582779));
#78529=CARTESIAN_POINT('Origin',(141.,3.26619676656571,11.0305012887935));
#78530=CARTESIAN_POINT('',(141.,2.58311365275126,10.7994223853394));
#78531=CARTESIAN_POINT('',(141.,2.19674332223563,10.9029500033804));
#78532=CARTESIAN_POINT('',(141.,2.30027094027664,11.289320333896));
#78533=CARTESIAN_POINT('Origin',(141.,2.68664127079227,11.185792715855));
#78534=CARTESIAN_POINT('',(141.,2.42439173773413,11.7525454562834));
#78535=CARTESIAN_POINT('',(141.,2.53320808086891,12.1586535775562));
#78536=CARTESIAN_POINT('',(141.,0.700000000000001,11.9795659353751));
#78537=CARTESIAN_POINT('Origin',(141.,0.,0.));
#78538=CARTESIAN_POINT('',(141.,0.700000000000001,11.5));
#78539=CARTESIAN_POINT('',(141.,0.700000000000001,11.1));
#78540=CARTESIAN_POINT('',(141.,0.300000000000001,11.1));
#78541=CARTESIAN_POINT('Origin',(141.,0.300000000000001,11.5));
#78542=CARTESIAN_POINT('',(141.,-0.299999999999999,11.1));
#78543=CARTESIAN_POINT('',(141.,-0.699999999999999,11.1));
#78544=CARTESIAN_POINT('',(141.,-0.699999999999999,11.5));
#78545=CARTESIAN_POINT('Origin',(141.,-0.299999999999999,11.5));
#78546=CARTESIAN_POINT('',(141.,-0.699999999999999,11.9795659353751));
#78547=CARTESIAN_POINT('',(141.,-0.699999999999999,12.4));
#78548=CARTESIAN_POINT('',(141.,-2.42439173773413,11.7525454562834));
#78549=CARTESIAN_POINT('Origin',(141.,0.,0.));
#78550=CARTESIAN_POINT('',(141.,-2.30027094027664,11.289320333896));
#78551=CARTESIAN_POINT('',(141.,-2.19674332223563,10.9029500033804));
#78552=CARTESIAN_POINT('',(141.,-2.58311365275126,10.7994223853394));
#78553=CARTESIAN_POINT('Origin',(141.,-2.68664127079227,11.185792715855));
#78554=CARTESIAN_POINT('',(141.,-3.1626691485247,10.6441309582779));
#78555=CARTESIAN_POINT('',(141.,-3.54903947904033,10.5406033402369));
#78556=CARTESIAN_POINT('',(141.,-3.65256709708133,10.9269736707525));
#78557=CARTESIAN_POINT('Origin',(141.,-3.26619676656571,11.0305012887935));
#78558=CARTESIAN_POINT('',(141.,-3.77668789453882,11.3901987931398));
#78559=CARTESIAN_POINT('',(141.,-3.8855042376736,11.7963069144127));
#78560=CARTESIAN_POINT('',(141.,-5.38356518503845,10.7246084263455));
#78561=CARTESIAN_POINT('Origin',(141.,0.,0.));
#78562=CARTESIAN_POINT('',(141.,-5.14378221735089,10.309292143521));
#78563=CARTESIAN_POINT('',(141.,-4.94378221735089,9.96288198200727));
#78564=CARTESIAN_POINT('',(141.,-5.29019237886467,9.76288198200727));
#78565=CARTESIAN_POINT('Origin',(141.,-5.49019237886467,10.109292143521));
#78566=CARTESIAN_POINT('',(141.,-5.80980762113533,9.46288198200727));
#78567=CARTESIAN_POINT('',(141.,-6.1562177826491,9.26288198200727));
#78568=CARTESIAN_POINT('',(141.,-6.3562177826491,9.60929214352105));
#78569=CARTESIAN_POINT('Origin',(141.,-6.00980762113533,9.80929214352104));
#78570=CARTESIAN_POINT('',(141.,-6.59600075033666,10.0246084263455));
#78571=CARTESIAN_POINT('',(141.,-6.8062177826491,10.388715006927));
#78572=CARTESIAN_POINT('',(141.,-7.97585756174453,8.9658070554057));
#78573=CARTESIAN_POINT('Origin',(141.,0.,0.));
#78574=CARTESIAN_POINT('',(141.,-7.63675323681471,8.62670273047588));
#78575=CARTESIAN_POINT('',(141.,-7.35391052434009,8.34386001800126));
#78576=CARTESIAN_POINT('',(141.,-7.63675323681471,8.06101730552664));
#78577=CARTESIAN_POINT('Origin',(141.,-7.91959594928933,8.34386001800126));
#78578=CARTESIAN_POINT('',(141.,-8.06101730552664,7.63675323681471));
#78579=CARTESIAN_POINT('',(141.,-8.34386001800126,7.35391052434009));
#78580=CARTESIAN_POINT('',(141.,-8.62670273047588,7.63675323681471));
#78581=CARTESIAN_POINT('Origin',(141.,-8.34386001800126,7.91959594928933));
#78582=CARTESIAN_POINT('',(141.,-8.9658070554057,7.97585756174453));
#78583=CARTESIAN_POINT('',(141.,-9.26309883354377,8.27314933988261));
#78584=CARTESIAN_POINT('',(141.,-10.0246084263455,6.59600075033667));
#78585=CARTESIAN_POINT('Origin',(141.,0.,0.));
#78586=CARTESIAN_POINT('',(141.,-9.60929214352104,6.35621778264911));
#78587=CARTESIAN_POINT('',(141.,-9.26288198200727,6.15621778264911));
#78588=CARTESIAN_POINT('',(141.,-9.46288198200727,5.80980762113533));
#78589=CARTESIAN_POINT('Origin',(141.,-9.80929214352104,6.00980762113534));
#78590=CARTESIAN_POINT('',(141.,-9.76288198200727,5.29019237886467));
#78591=CARTESIAN_POINT('',(141.,-9.96288198200727,4.9437822173509));
#78592=CARTESIAN_POINT('',(141.,-10.309292143521,5.1437822173509));
#78593=CARTESIAN_POINT('Origin',(141.,-10.109292143521,5.49019237886467));
#78594=CARTESIAN_POINT('',(141.,-10.7246084263455,5.38356518503846));
#78595=CARTESIAN_POINT('',(141.,-11.088715006927,5.5937822173509));
#78596=CARTESIAN_POINT('',(141.,-11.3901987931398,3.77668789453883));
#78597=CARTESIAN_POINT('Origin',(141.,0.,0.));
#78598=CARTESIAN_POINT('',(141.,-10.9269736707525,3.65256709708134));
#78599=CARTESIAN_POINT('',(141.,-10.5406033402369,3.54903947904033));
#78600=CARTESIAN_POINT('',(141.,-10.6441309582779,3.1626691485247));
#78601=CARTESIAN_POINT('Origin',(141.,-11.0305012887935,3.26619676656571));
#78602=CARTESIAN_POINT('',(141.,-10.7994223853394,2.58311365275126));
#78603=CARTESIAN_POINT('',(141.,-10.9029500033804,2.19674332223564));
#78604=CARTESIAN_POINT('',(141.,-11.289320333896,2.30027094027664));
#78605=CARTESIAN_POINT('Origin',(141.,-11.185792715855,2.68664127079227));
#78606=CARTESIAN_POINT('',(141.,-11.7525454562834,2.42439173773413));
#78607=CARTESIAN_POINT('',(141.,-12.1586535775562,2.53320808086891));
#78608=CARTESIAN_POINT('',(141.,-11.9795659353751,0.700000000000002));
#78609=CARTESIAN_POINT('Origin',(141.,0.,0.));
#78610=CARTESIAN_POINT('',(141.,-11.5,0.700000000000001));
#78611=CARTESIAN_POINT('',(141.,-11.1,0.700000000000001));
#78612=CARTESIAN_POINT('',(141.,-11.1,0.300000000000001));
#78613=CARTESIAN_POINT('Origin',(141.,-11.5,0.300000000000001));
#78614=CARTESIAN_POINT('',(141.,-11.1,-0.299999999999998));
#78615=CARTESIAN_POINT('',(141.,-11.1,-0.699999999999999));
#78616=CARTESIAN_POINT('',(141.,-11.5,-0.699999999999999));
#78617=CARTESIAN_POINT('Origin',(141.,-11.5,-0.299999999999998));
#78618=CARTESIAN_POINT('',(141.,-11.9795659353751,-0.699999999999998));
#78619=CARTESIAN_POINT('',(141.,-12.4,-0.699999999999998));
#78620=CARTESIAN_POINT('',(141.,-11.7525454562834,-2.42439173773412));
#78621=CARTESIAN_POINT('Origin',(141.,0.,0.));
#78622=CARTESIAN_POINT('',(141.,-11.2893203338961,-2.30027094027664));
#78623=CARTESIAN_POINT('',(141.,-10.9029500033804,-2.19674332223563));
#78624=CARTESIAN_POINT('',(141.,-10.7994223853394,-2.58311365275126));
#78625=CARTESIAN_POINT('Origin',(141.,-11.185792715855,-2.68664127079226));
#78626=CARTESIAN_POINT('',(141.,-10.6441309582779,-3.1626691485247));
#78627=CARTESIAN_POINT('',(141.,-10.5406033402369,-3.54903947904032));
#78628=CARTESIAN_POINT('',(141.,-10.9269736707525,-3.65256709708133));
#78629=CARTESIAN_POINT('Origin',(141.,-11.0305012887935,-3.2661967665657));
#78630=CARTESIAN_POINT('',(141.,-11.3901987931398,-3.77668789453882));
#78631=CARTESIAN_POINT('',(141.,-11.7963069144127,-3.8855042376736));
#78632=CARTESIAN_POINT('',(141.,-10.7246084263455,-5.38356518503845));
#78633=CARTESIAN_POINT('Origin',(141.,0.,0.));
#78634=CARTESIAN_POINT('',(141.,-10.309292143521,-5.14378221735089));
#78635=CARTESIAN_POINT('',(141.,-9.96288198200727,-4.94378221735089));
#78636=CARTESIAN_POINT('',(141.,-9.76288198200727,-5.29019237886466));
#78637=CARTESIAN_POINT('Origin',(141.,-10.109292143521,-5.49019237886466));
#78638=CARTESIAN_POINT('',(141.,-9.46288198200727,-5.80980762113533));
#78639=CARTESIAN_POINT('',(141.,-9.26288198200727,-6.1562177826491));
#78640=CARTESIAN_POINT('',(141.,-9.60929214352105,-6.3562177826491));
#78641=CARTESIAN_POINT('Origin',(141.,-9.80929214352104,-6.00980762113533));
#78642=CARTESIAN_POINT('',(141.,-10.0246084263455,-6.59600075033666));
#78643=CARTESIAN_POINT('',(141.,-10.388715006927,-6.8062177826491));
#78644=CARTESIAN_POINT('',(141.,-8.9658070554057,-7.97585756174453));
#78645=CARTESIAN_POINT('Origin',(141.,0.,0.));
#78646=CARTESIAN_POINT('',(141.,-8.62670273047588,-7.63675323681471));
#78647=CARTESIAN_POINT('',(141.,-8.34386001800126,-7.35391052434009));
#78648=CARTESIAN_POINT('',(141.,-8.06101730552665,-7.63675323681471));
#78649=CARTESIAN_POINT('Origin',(141.,-8.34386001800126,-7.91959594928933));
#78650=CARTESIAN_POINT('',(141.,-7.63675323681472,-8.06101730552664));
#78651=CARTESIAN_POINT('',(141.,-7.3539105243401,-8.34386001800125));
#78652=CARTESIAN_POINT('',(141.,-7.63675323681472,-8.62670273047588));
#78653=CARTESIAN_POINT('Origin',(141.,-7.91959594928934,-8.34386001800125));
#78654=CARTESIAN_POINT('',(141.,-7.97585756174453,-8.96580705540569));
#78655=CARTESIAN_POINT('',(141.,-8.27314933988261,-9.26309883354377));
#78656=CARTESIAN_POINT('',(141.,-6.59600075033667,-10.0246084263455));
#78657=CARTESIAN_POINT('Origin',(141.,0.,0.));
#78658=CARTESIAN_POINT('',(141.,-6.35621778264911,-9.60929214352104));
#78659=CARTESIAN_POINT('',(141.,-6.15621778264911,-9.26288198200726));
#78660=CARTESIAN_POINT('',(141.,-5.80980762113534,-9.46288198200726));
#78661=CARTESIAN_POINT('Origin',(141.,-6.00980762113534,-9.80929214352104));
#78662=CARTESIAN_POINT('',(141.,-5.29019237886467,-9.76288198200726));
#78663=CARTESIAN_POINT('',(141.,-4.9437822173509,-9.96288198200727));
#78664=CARTESIAN_POINT('',(141.,-5.1437822173509,-10.309292143521));
#78665=CARTESIAN_POINT('Origin',(141.,-5.49019237886467,-10.109292143521));
#78666=CARTESIAN_POINT('',(141.,-5.38356518503846,-10.7246084263455));
#78667=CARTESIAN_POINT('',(141.,-5.5937822173509,-11.088715006927));
#78668=CARTESIAN_POINT('',(141.,-3.77668789453883,-11.3901987931398));
#78669=CARTESIAN_POINT('Origin',(141.,0.,0.));
#78670=CARTESIAN_POINT('',(141.,-3.65256709708134,-10.9269736707525));
#78671=CARTESIAN_POINT('',(141.,-3.54903947904034,-10.5406033402369));
#78672=CARTESIAN_POINT('',(141.,-3.16266914852471,-10.6441309582779));
#78673=CARTESIAN_POINT('Origin',(141.,-3.26619676656572,-11.0305012887935));
#78674=CARTESIAN_POINT('',(141.,-2.58311365275127,-10.7994223853394));
#78675=CARTESIAN_POINT('',(141.,-2.19674332223564,-10.9029500033804));
#78676=CARTESIAN_POINT('',(141.,-2.30027094027665,-11.289320333896));
#78677=CARTESIAN_POINT('Origin',(141.,-2.68664127079228,-11.185792715855));
#78678=CARTESIAN_POINT('',(141.,-2.42439173773414,-11.7525454562834));
#78679=CARTESIAN_POINT('',(141.,-2.53320808086892,-12.1586535775562));
#78680=CARTESIAN_POINT('',(141.,-0.700000000000002,-11.9795659353751));
#78681=CARTESIAN_POINT('Origin',(141.,0.,0.));
#78682=CARTESIAN_POINT('',(141.,-0.700000000000002,-11.5));
#78683=CARTESIAN_POINT('',(141.,-0.700000000000002,-11.1));
#78684=CARTESIAN_POINT('',(141.,-0.300000000000002,-11.1));
#78685=CARTESIAN_POINT('Origin',(141.,-0.300000000000002,-11.5));
#78686=CARTESIAN_POINT('',(141.,0.299999999999998,-11.1));
#78687=CARTESIAN_POINT('',(141.,0.699999999999998,-11.1));
#78688=CARTESIAN_POINT('',(141.,0.699999999999998,-11.5));
#78689=CARTESIAN_POINT('Origin',(141.,0.299999999999998,-11.5));
#78690=CARTESIAN_POINT('',(141.,0.699999999999998,-11.9795659353751));
#78691=CARTESIAN_POINT('',(141.,0.699999999999998,-12.4));
#78692=CARTESIAN_POINT('',(141.,2.42439173773412,-11.7525454562834));
#78693=CARTESIAN_POINT('Origin',(141.,0.,0.));
#78694=CARTESIAN_POINT('',(141.,2.30027094027664,-11.2893203338961));
#78695=CARTESIAN_POINT('',(141.,2.19674332223563,-10.9029500033804));
#78696=CARTESIAN_POINT('',(141.,2.58311365275125,-10.7994223853394));
#78697=CARTESIAN_POINT('Origin',(141.,2.68664127079226,-11.185792715855));
#78698=CARTESIAN_POINT('',(141.,3.1626691485247,-10.6441309582779));
#78699=CARTESIAN_POINT('',(141.,3.54903947904032,-10.5406033402369));
#78700=CARTESIAN_POINT('',(141.,3.65256709708133,-10.9269736707525));
#78701=CARTESIAN_POINT('Origin',(141.,3.2661967665657,-11.0305012887935));
#78702=CARTESIAN_POINT('',(141.,3.77668789453882,-11.3901987931398));
#78703=CARTESIAN_POINT('',(141.,3.8855042376736,-11.7963069144127));
#78704=CARTESIAN_POINT('',(141.,5.38356518503845,-10.7246084263456));
#78705=CARTESIAN_POINT('Origin',(141.,0.,0.));
#78706=CARTESIAN_POINT('',(141.,5.14378221735088,-10.309292143521));
#78707=CARTESIAN_POINT('',(141.,4.94378221735088,-9.96288198200727));
#78708=CARTESIAN_POINT('',(141.,5.29019237886466,-9.76288198200727));
#78709=CARTESIAN_POINT('Origin',(141.,5.49019237886466,-10.109292143521));
#78710=CARTESIAN_POINT('',(141.,5.80980762113532,-9.46288198200727));
#78711=CARTESIAN_POINT('',(141.,6.1562177826491,-9.26288198200727));
#78712=CARTESIAN_POINT('',(141.,6.3562177826491,-9.60929214352105));
#78713=CARTESIAN_POINT('Origin',(141.,6.00980762113532,-9.80929214352105));
#78714=CARTESIAN_POINT('',(141.,6.59600075033666,-10.0246084263456));
#78715=CARTESIAN_POINT('',(141.,6.8062177826491,-10.388715006927));
#78716=CARTESIAN_POINT('',(141.,7.97585756174453,-8.9658070554057));
#78717=CARTESIAN_POINT('Origin',(141.,0.,0.));
#78718=CARTESIAN_POINT('',(141.,7.63675323681471,-8.62670273047588));
#78719=CARTESIAN_POINT('',(141.,7.35391052434009,-8.34386001800126));
#78720=CARTESIAN_POINT('',(141.,7.63675323681471,-8.06101730552664));
#78721=CARTESIAN_POINT('Origin',(141.,7.91959594928933,-8.34386001800126));
#78722=CARTESIAN_POINT('',(141.,8.06101730552664,-7.63675323681472));
#78723=CARTESIAN_POINT('',(141.,8.34386001800126,-7.35391052434009));
#78724=CARTESIAN_POINT('',(141.,8.62670273047588,-7.63675323681471));
#78725=CARTESIAN_POINT('Origin',(141.,8.34386001800126,-7.91959594928933));
#78726=CARTESIAN_POINT('',(141.,8.96580705540569,-7.97585756174453));
#78727=CARTESIAN_POINT('',(141.,9.26309883354377,-8.27314933988261));
#78728=CARTESIAN_POINT('',(141.,10.0246084263455,-6.59600075033667));
#78729=CARTESIAN_POINT('Origin',(141.,0.,0.));
#78730=CARTESIAN_POINT('',(141.,9.60929214352104,-6.35621778264911));
#78731=CARTESIAN_POINT('',(141.,9.26288198200726,-6.15621778264911));
#78732=CARTESIAN_POINT('',(141.,9.46288198200726,-5.80980762113534));
#78733=CARTESIAN_POINT('Origin',(141.,9.80929214352104,-6.00980762113534));
#78734=CARTESIAN_POINT('',(141.,9.76288198200726,-5.29019237886467));
#78735=CARTESIAN_POINT('',(141.,9.96288198200727,-4.9437822173509));
#78736=CARTESIAN_POINT('',(141.,10.309292143521,-5.1437822173509));
#78737=CARTESIAN_POINT('Origin',(141.,10.109292143521,-5.49019237886467));
#78738=CARTESIAN_POINT('',(141.,10.7246084263455,-5.38356518503846));
#78739=CARTESIAN_POINT('',(141.,11.088715006927,-5.5937822173509));
#78740=CARTESIAN_POINT('',(141.,11.3901987931398,-3.77668789453883));
#78741=CARTESIAN_POINT('Origin',(141.,0.,0.));
#78742=CARTESIAN_POINT('',(141.,10.9269736707525,-3.65256709708134));
#78743=CARTESIAN_POINT('',(141.,10.5406033402369,-3.54903947904034));
#78744=CARTESIAN_POINT('',(141.,10.6441309582779,-3.16266914852471));
#78745=CARTESIAN_POINT('Origin',(141.,11.0305012887935,-3.26619676656572));
#78746=CARTESIAN_POINT('',(141.,10.7994223853394,-2.58311365275127));
#78747=CARTESIAN_POINT('',(141.,10.9029500033804,-2.19674332223564));
#78748=CARTESIAN_POINT('',(141.,11.289320333896,-2.30027094027665));
#78749=CARTESIAN_POINT('Origin',(141.,11.185792715855,-2.68664127079228));
#78750=CARTESIAN_POINT('',(141.,11.7525454562834,-2.42439173773414));
#78751=CARTESIAN_POINT('',(141.,12.1586535775562,-2.53320808086892));
#78752=CARTESIAN_POINT('',(141.,11.9795659353751,-0.7));
#78753=CARTESIAN_POINT('Origin',(141.,0.,0.));
#78754=CARTESIAN_POINT('',(141.,11.1,-0.7));
#78755=CARTESIAN_POINT('Origin',(141.,11.0305012887935,3.26619676656571));
#78756=CARTESIAN_POINT('',(159.,10.6441309582779,3.1626691485247));
#78757=CARTESIAN_POINT('',(159.,10.9269736707525,3.65256709708134));
#78758=CARTESIAN_POINT('Origin',(159.,11.0305012887935,3.26619676656571));
#78759=CARTESIAN_POINT('',(141.,10.9269736707525,3.65256709708134));
#78760=CARTESIAN_POINT('',(141.,10.6441309582779,3.1626691485247));
#78761=CARTESIAN_POINT('Origin',(141.,11.7963069144127,3.8855042376736));
#78762=CARTESIAN_POINT('',(159.,11.3901987931398,3.77668789453882));
#78763=CARTESIAN_POINT('',(159.,11.7963069144127,3.8855042376736));
#78764=CARTESIAN_POINT('',(150.,11.3901987931398,3.77668789453882));
#78765=CARTESIAN_POINT('Origin',(159.,12.,0.));
#78766=CARTESIAN_POINT('',(159.,11.9468127170547,1.12856807664441));
#78767=CARTESIAN_POINT('Origin',(159.,0.,0.));
#78768=CARTESIAN_POINT('',(159.,19.325905913425,7.95671795563006));
#78769=CARTESIAN_POINT('Ctrl Pts',(159.,19.3259059134355,7.95671795563314));
#78770=CARTESIAN_POINT('Ctrl Pts',(159.,17.3255467234756,7.37182014405471));
#78771=CARTESIAN_POINT('Ctrl Pts',(159.,14.5165477492305,5.77538011759181));
#78772=CARTESIAN_POINT('Ctrl Pts',(159.,12.445579418008,2.87212152134714));
#78773=CARTESIAN_POINT('Ctrl Pts',(159.,12.0234100907472,1.50200893235404));
#78774=CARTESIAN_POINT('Ctrl Pts',(159.,11.9469717453788,1.12853552863424));
#78775=CARTESIAN_POINT('',(159.,16.5536728370359,12.7583664943589));
#78776=CARTESIAN_POINT('Origin',(159.,-1.33226762955019E-14,0.));
#78777=CARTESIAN_POINT('',(159.,6.95077498280155,9.7819592689022));
#78778=CARTESIAN_POINT('Ctrl Pts',(159.,6.95092542742434,9.78241301256989));
#78779=CARTESIAN_POINT('Ctrl Pts',(159.,7.80418402739543,9.49950253045326));
#78780=CARTESIAN_POINT('Ctrl Pts',(159.,9.77882982348217,9.32502435050667));
#78781=CARTESIAN_POINT('Ctrl Pts',(159.,13.2082488270869,10.2260207456149));
#78782=CARTESIAN_POINT('Ctrl Pts',(159.,15.423567841049,11.6783667562432));
#78783=CARTESIAN_POINT('Ctrl Pts',(159.,16.5536728370359,12.7583664943589));
#78784=CARTESIAN_POINT('',(159.,7.97585756174453,8.9658070554057));
#78785=CARTESIAN_POINT('Origin',(159.,0.,0.));
#78786=CARTESIAN_POINT('',(159.,7.63675323681471,8.62670273047588));
#78787=CARTESIAN_POINT('',(159.,8.27314933988261,9.26309883354377));
#78788=CARTESIAN_POINT('',(159.,7.63675323681471,8.06101730552664));
#78789=CARTESIAN_POINT('Origin',(159.,7.91959594928933,8.34386001800126));
#78790=CARTESIAN_POINT('',(159.,8.06101730552664,7.63675323681471));
#78791=CARTESIAN_POINT('',(159.,7.35391052434009,8.34386001800126));
#78792=CARTESIAN_POINT('',(159.,8.62670273047588,7.63675323681471));
#78793=CARTESIAN_POINT('Origin',(159.,8.34386001800126,7.91959594928933));
#78794=CARTESIAN_POINT('',(159.,8.9658070554057,7.97585756174453));
#78795=CARTESIAN_POINT('',(159.,8.34386001800126,7.35391052434009));
#78796=CARTESIAN_POINT('',(159.,10.0246084263455,6.59600075033667));
#78797=CARTESIAN_POINT('Origin',(159.,0.,0.));
#78798=CARTESIAN_POINT('',(159.,9.60929214352104,6.35621778264911));
#78799=CARTESIAN_POINT('',(159.,10.388715006927,6.80621778264911));
#78800=CARTESIAN_POINT('',(159.,9.46288198200727,5.80980762113533));
#78801=CARTESIAN_POINT('Origin',(159.,9.80929214352104,6.00980762113533));
#78802=CARTESIAN_POINT('',(159.,9.76288198200727,5.29019237886467));
#78803=CARTESIAN_POINT('',(159.,9.26288198200727,6.1562177826491));
#78804=CARTESIAN_POINT('',(159.,10.309292143521,5.14378221735089));
#78805=CARTESIAN_POINT('Origin',(159.,10.109292143521,5.49019237886467));
#78806=CARTESIAN_POINT('',(159.,10.7246084263455,5.38356518503845));
#78807=CARTESIAN_POINT('',(159.,9.96288198200727,4.94378221735089));
#78808=CARTESIAN_POINT('Origin',(159.,0.,0.));
#78809=CARTESIAN_POINT('',(159.,10.5406033402369,3.54903947904033));
#78810=CARTESIAN_POINT('Origin',(141.,10.109292143521,5.49019237886467));
#78811=CARTESIAN_POINT('',(141.,9.76288198200727,5.29019237886467));
#78812=CARTESIAN_POINT('',(141.,10.309292143521,5.14378221735089));
#78813=CARTESIAN_POINT('Origin',(141.,9.26288198200727,6.1562177826491));
#78814=CARTESIAN_POINT('',(141.,9.46288198200727,5.80980762113533));
#78815=CARTESIAN_POINT('Origin',(141.,9.80929214352104,6.00980762113533));
#78816=CARTESIAN_POINT('',(141.,9.60929214352104,6.35621778264911));
#78817=CARTESIAN_POINT('Origin',(141.,7.91959594928933,8.34386001800126));
#78818=CARTESIAN_POINT('',(141.,7.63675323681471,8.62670273047588));
#78819=CARTESIAN_POINT('',(141.,7.63675323681471,8.06101730552664));
#78820=CARTESIAN_POINT('Origin',(141.,7.35391052434009,8.34386001800126));
#78821=CARTESIAN_POINT('',(141.,8.06101730552664,7.63675323681471));
#78822=CARTESIAN_POINT('Origin',(141.,8.34386001800126,7.91959594928933));
#78823=CARTESIAN_POINT('',(141.,8.62670273047588,7.63675323681471));
#78824=CARTESIAN_POINT('Origin',(141.,5.49019237886467,10.109292143521));
#78825=CARTESIAN_POINT('',(159.,5.29019237886467,9.76288198200727));
#78826=CARTESIAN_POINT('',(159.,5.14378221735089,10.309292143521));
#78827=CARTESIAN_POINT('Origin',(159.,5.49019237886467,10.109292143521));
#78828=CARTESIAN_POINT('',(141.,5.14378221735089,10.309292143521));
#78829=CARTESIAN_POINT('',(141.,5.29019237886467,9.76288198200727));
#78830=CARTESIAN_POINT('Origin',(159.,12.,0.));
#78831=CARTESIAN_POINT('',(159.,5.80980762113533,9.46288198200727));
#78832=CARTESIAN_POINT('',(159.,4.94378221735089,9.96288198200727));
#78833=CARTESIAN_POINT('',(159.,6.35621778264911,9.60929214352104));
#78834=CARTESIAN_POINT('Origin',(159.,6.00980762113533,9.80929214352104));
#78835=CARTESIAN_POINT('',(159.,6.80621778264911,10.388715006927));
#78836=CARTESIAN_POINT('',(159.,6.15621778264911,9.26288198200727));
#78837=CARTESIAN_POINT('',(159.,5.59378221735089,11.088715006927));
#78838=CARTESIAN_POINT('',(159.,6.80621778264911,10.388715006927));
#78839=CARTESIAN_POINT('',(159.,3.99378221735089,8.31743371481684));
#78840=CARTESIAN_POINT('Origin',(141.,4.94378221735089,9.96288198200727));
#78841=CARTESIAN_POINT('',(141.,5.80980762113533,9.46288198200727));
#78842=CARTESIAN_POINT('Origin',(141.,6.00980762113533,9.80929214352104));
#78843=CARTESIAN_POINT('',(141.,6.35621778264911,9.60929214352104));
#78844=CARTESIAN_POINT('Origin',(141.,2.68664127079227,11.185792715855));
#78845=CARTESIAN_POINT('',(159.,2.58311365275126,10.7994223853394));
#78846=CARTESIAN_POINT('',(159.,2.30027094027664,11.289320333896));
#78847=CARTESIAN_POINT('Origin',(159.,2.68664127079227,11.185792715855));
#78848=CARTESIAN_POINT('',(141.,2.30027094027664,11.289320333896));
#78849=CARTESIAN_POINT('',(141.,2.58311365275126,10.7994223853394));
#78850=CARTESIAN_POINT('Origin',(159.,12.,0.));
#78851=CARTESIAN_POINT('',(159.,3.1626691485247,10.6441309582779));
#78852=CARTESIAN_POINT('',(159.,2.19674332223563,10.9029500033804));
#78853=CARTESIAN_POINT('',(159.,3.65256709708134,10.9269736707525));
#78854=CARTESIAN_POINT('Origin',(159.,3.26619676656571,11.0305012887935));
#78855=CARTESIAN_POINT('',(159.,3.77668789453883,11.3901987931398));
#78856=CARTESIAN_POINT('',(159.,3.54903947904033,10.5406033402369));
#78857=CARTESIAN_POINT('',(159.,4.99603773425319,10.9105273455466));
#78858=CARTESIAN_POINT('Origin',(159.,0.,0.));
#78859=CARTESIAN_POINT('',(159.,2.77223307638908,20.715084449989));
#78860=CARTESIAN_POINT('Ctrl Pts',(159.,2.77223307638908,20.715084449989));
#78861=CARTESIAN_POINT('Ctrl Pts',(159.,2.27856692641562,18.6901796628404));
#78862=CARTESIAN_POINT('Ctrl Pts',(159.,2.25666246318025,15.4594048368281));
#78863=CARTESIAN_POINT('Ctrl Pts',(159.,3.73545952488756,12.2142321737801));
#78864=CARTESIAN_POINT('Ctrl Pts',(159.,4.71092715448988,11.1635802020065));
#78865=CARTESIAN_POINT('Ctrl Pts',(159.,4.99614489241639,10.9106481821829));
#78866=CARTESIAN_POINT('',(159.,-2.77223307638907,20.715084449989));
#78867=CARTESIAN_POINT('Origin',(159.,-1.33226762955019E-14,0.));
#78868=CARTESIAN_POINT('',(159.,-4.99603773425319,10.9105273455466));
#78869=CARTESIAN_POINT('Ctrl Pts',(159.,-4.9961924138399,10.9107016057014));
#78870=CARTESIAN_POINT('Ctrl Pts',(159.,-4.32378633865339,11.5075500836844));
#78871=CARTESIAN_POINT('Ctrl Pts',(159.,-3.48628190063569,12.6916836134711));
#78872=CARTESIAN_POINT('Ctrl Pts',(159.,-2.26648621108045,15.9916186244315));
#78873=CARTESIAN_POINT('Ctrl Pts',(159.,-2.27856657179338,18.6901782082677));
#78874=CARTESIAN_POINT('Ctrl Pts',(159.,-2.7722330763911,20.7150844499973));
#78875=CARTESIAN_POINT('',(159.,-3.77668789453882,11.3901987931398));
#78876=CARTESIAN_POINT('Origin',(159.,0.,0.));
#78877=CARTESIAN_POINT('',(159.,-3.65256709708133,10.9269736707525));
#78878=CARTESIAN_POINT('',(159.,-3.8855042376736,11.7963069144127));
#78879=CARTESIAN_POINT('',(159.,-3.1626691485247,10.6441309582779));
#78880=CARTESIAN_POINT('Origin',(159.,-3.26619676656571,11.0305012887935));
#78881=CARTESIAN_POINT('',(159.,-2.58311365275126,10.7994223853394));
#78882=CARTESIAN_POINT('',(159.,-3.54903947904033,10.5406033402369));
#78883=CARTESIAN_POINT('',(159.,-2.30027094027664,11.289320333896));
#78884=CARTESIAN_POINT('Origin',(159.,-2.68664127079227,11.185792715855));
#78885=CARTESIAN_POINT('',(159.,-2.42439173773413,11.7525454562834));
#78886=CARTESIAN_POINT('',(159.,-2.19674332223563,10.9029500033804));
#78887=CARTESIAN_POINT('',(159.,-0.699999999999999,11.9795659353751));
#78888=CARTESIAN_POINT('Origin',(159.,0.,0.));
#78889=CARTESIAN_POINT('',(159.,-0.699999999999999,11.5));
#78890=CARTESIAN_POINT('',(159.,-0.699999999999999,12.4));
#78891=CARTESIAN_POINT('',(159.,-0.299999999999999,11.1));
#78892=CARTESIAN_POINT('Origin',(159.,-0.299999999999999,11.5));
#78893=CARTESIAN_POINT('',(159.,0.300000000000001,11.1));
#78894=CARTESIAN_POINT('',(159.,-0.699999999999999,11.1));
#78895=CARTESIAN_POINT('',(159.,0.700000000000001,11.5));
#78896=CARTESIAN_POINT('Origin',(159.,0.300000000000001,11.5));
#78897=CARTESIAN_POINT('',(159.,0.700000000000001,11.9795659353751));
#78898=CARTESIAN_POINT('',(159.,0.700000000000001,11.1));
#78899=CARTESIAN_POINT('',(159.,2.42439173773413,11.7525454562834));
#78900=CARTESIAN_POINT('Origin',(159.,0.,0.));
#78901=CARTESIAN_POINT('',(159.,2.53320808086891,12.1586535775562));
#78902=CARTESIAN_POINT('Origin',(141.,2.19674332223563,10.9029500033804));
#78903=CARTESIAN_POINT('',(141.,3.1626691485247,10.6441309582779));
#78904=CARTESIAN_POINT('Origin',(141.,3.26619676656571,11.0305012887935));
#78905=CARTESIAN_POINT('',(141.,3.65256709708134,10.9269736707525));
#78906=CARTESIAN_POINT('Origin',(141.,0.300000000000001,11.5));
#78907=CARTESIAN_POINT('',(141.,0.3,11.1));
#78908=CARTESIAN_POINT('',(141.,0.700000000000001,11.5));
#78909=CARTESIAN_POINT('Origin',(141.,0.700000000000001,11.1));
#78910=CARTESIAN_POINT('',(150.,0.700000000000001,11.9795659353751));
#78911=CARTESIAN_POINT('Origin',(141.,-0.299999999999999,11.5));
#78912=CARTESIAN_POINT('',(141.,-0.699999999999999,11.5));
#78913=CARTESIAN_POINT('',(141.,-0.299999999999999,11.1));
#78914=CARTESIAN_POINT('Origin',(141.,-0.699999999999999,12.4));
#78915=CARTESIAN_POINT('',(150.,-0.699999999999999,11.9795659353751));
#78916=CARTESIAN_POINT('Origin',(141.,-2.68664127079227,11.185792715855));
#78917=CARTESIAN_POINT('',(141.,-2.58311365275126,10.7994223853394));
#78918=CARTESIAN_POINT('',(141.,-2.30027094027664,11.289320333896));
#78919=CARTESIAN_POINT('Origin',(141.,-2.19674332223563,10.9029500033804));
#78920=CARTESIAN_POINT('',(150.,-2.42439173773413,11.7525454562834));
#78921=CARTESIAN_POINT('Origin',(141.,-3.26619676656571,11.0305012887935));
#78922=CARTESIAN_POINT('',(141.,-3.65256709708133,10.9269736707525));
#78923=CARTESIAN_POINT('',(141.,-3.1626691485247,10.6441309582779));
#78924=CARTESIAN_POINT('Origin',(141.,-3.8855042376736,11.7963069144127));
#78925=CARTESIAN_POINT('',(150.,-3.77668789453882,11.3901987931398));
#78926=CARTESIAN_POINT('Origin',(141.,-5.49019237886467,10.109292143521));
#78927=CARTESIAN_POINT('',(159.,-5.14378221735089,10.309292143521));
#78928=CARTESIAN_POINT('',(159.,-5.29019237886467,9.76288198200727));
#78929=CARTESIAN_POINT('Origin',(159.,-5.49019237886467,10.109292143521));
#78930=CARTESIAN_POINT('',(141.,-5.29019237886467,9.76288198200727));
#78931=CARTESIAN_POINT('',(141.,-5.14378221735089,10.309292143521));
#78932=CARTESIAN_POINT('Origin',(141.,-4.94378221735089,9.96288198200727));
#78933=CARTESIAN_POINT('',(158.9865805553,-5.38356518503845,10.7246084263455));
#78934=CARTESIAN_POINT('',(150.,-5.38356518503845,10.7246084263455));
#78935=CARTESIAN_POINT('',(158.90010356288,-5.46511181578873,10.8658513339894));
#78936=CARTESIAN_POINT('Ctrl Pts',(158.986559824909,-5.38356357140902,10.7246063109672));
#78937=CARTESIAN_POINT('Ctrl Pts',(158.983100450767,-5.39013238902449,10.7359837190316));
#78938=CARTESIAN_POINT('Ctrl Pts',(158.978981181889,-5.39662057891906,10.7472214948867));
#78939=CARTESIAN_POINT('Ctrl Pts',(158.974203058392,-5.40300077120318,10.7582726051936));
#78940=CARTESIAN_POINT('Ctrl Pts',(158.966341561968,-5.41349816811402,10.7764551122452));
#78941=CARTESIAN_POINT('Ctrl Pts',(158.956755169878,-5.42362836369358,10.794003783507));
#78942=CARTESIAN_POINT('Ctrl Pts',(158.945582783954,-5.43329794081402,10.8107514019392));
#78943=CARTESIAN_POINT('Ctrl Pts',(158.934457379365,-5.44292685610521,10.827428594458));
#78944=CARTESIAN_POINT('Ctrl Pts',(158.921758537818,-5.45209972369878,10.8433124198025));
#78945=CARTESIAN_POINT('Ctrl Pts',(158.90758039377,-5.4607067410701,10.8582180101945));
#78946=CARTESIAN_POINT('Ctrl Pts',(158.905132179272,-5.46219295990413,10.8607918366686));
#78947=CARTESIAN_POINT('Ctrl Pts',(158.902639768354,-5.46366224948018,10.8633364271282));
#78948=CARTESIAN_POINT('Ctrl Pts',(158.900103540126,-5.46511396702284,10.8658507367904));
#78949=CARTESIAN_POINT('',(158.671029640456,-5.59378221735089,11.088715006927));
#78950=CARTESIAN_POINT('Origin',(145.,0.606217782649105,0.350000000000004));
#78951=CARTESIAN_POINT('',(159.,-5.59378221735089,11.088715006927));
#78952=CARTESIAN_POINT('',(141.,-5.59378221735089,11.088715006927));
#78953=CARTESIAN_POINT('',(159.,-4.94378221735089,9.96288198200727));
#78954=CARTESIAN_POINT('Origin',(141.,-6.00980762113533,9.80929214352104));
#78955=CARTESIAN_POINT('',(159.,-5.80980762113533,9.46288198200727));
#78956=CARTESIAN_POINT('',(159.,-6.3562177826491,9.60929214352104));
#78957=CARTESIAN_POINT('Origin',(159.,-6.00980762113533,9.80929214352104));
#78958=CARTESIAN_POINT('',(141.,-6.3562177826491,9.60929214352105));
#78959=CARTESIAN_POINT('',(141.,-5.80980762113533,9.46288198200727));
#78960=CARTESIAN_POINT('Origin',(141.,-6.8062177826491,10.388715006927));
#78961=CARTESIAN_POINT('',(159.,-6.8062177826491,10.388715006927));
#78962=CARTESIAN_POINT('',(159.,-2.20621778264911,2.42128129211021));
#78963=CARTESIAN_POINT('',(158.671029640456,-6.8062177826491,10.388715006927));
#78964=CARTESIAN_POINT('',(141.,-6.8062177826491,10.388715006927));
#78965=CARTESIAN_POINT('',(158.90010356288,-6.67754738108544,10.1658513339903));
#78966=CARTESIAN_POINT('Origin',(145.,-0.606217782649109,-0.349999999999996));
#78967=CARTESIAN_POINT('',(158.9865805553,-6.59600075033666,10.0246084263455));
#78968=CARTESIAN_POINT('Ctrl Pts',(158.900103510001,-6.67754593940625,10.1658536372963));
#78969=CARTESIAN_POINT('Ctrl Pts',(158.91477396803,-6.66914935312545,10.1513094162624));
#78970=CARTESIAN_POINT('Ctrl Pts',(158.927981140646,-6.66017043629784,10.1357525005376));
#78971=CARTESIAN_POINT('Ctrl Pts',(158.939637573624,-6.65071619580703,10.1193757733851));
#78972=CARTESIAN_POINT('Ctrl Pts',(158.951366829843,-6.64120289021064,10.1028967330834));
#78973=CARTESIAN_POINT('Ctrl Pts',(158.961526674818,-6.63120781888615,10.0855865098866));
#78974=CARTESIAN_POINT('Ctrl Pts',(158.969986224631,-6.62083026982913,10.0676132383608));
#78975=CARTESIAN_POINT('Ctrl Pts',(158.971442586,-6.61904371358417,10.0645190337167));
#78976=CARTESIAN_POINT('Ctrl Pts',(158.972848438657,-6.61724580860058,10.0614051333514));
#78977=CARTESIAN_POINT('Ctrl Pts',(158.974202964379,-6.6154370489256,10.0582723479436));
#78978=CARTESIAN_POINT('Ctrl Pts',(158.978981106332,-6.60905657911191,10.0472213260729));
#78979=CARTESIAN_POINT('Ctrl Pts',(158.98310039351,-6.60256845353527,10.0359834557292));
#78980=CARTESIAN_POINT('Ctrl Pts',(158.986559783722,-6.59599971918856,10.0246059568635));
#78981=CARTESIAN_POINT('',(150.,-6.59600075033666,10.0246084263455));
#78982=CARTESIAN_POINT('Origin',(159.,12.,0.));
#78983=CARTESIAN_POINT('',(159.,-5.59378221735089,11.088715006927));
#78984=CARTESIAN_POINT('',(159.,-6.1562177826491,9.26288198200727));
#78985=CARTESIAN_POINT('Origin',(141.,-8.34386001800126,7.91959594928933));
#78986=CARTESIAN_POINT('',(159.,-8.06101730552664,7.63675323681471));
#78987=CARTESIAN_POINT('',(159.,-8.62670273047588,7.63675323681471));
#78988=CARTESIAN_POINT('Origin',(159.,-8.34386001800126,7.91959594928933));
#78989=CARTESIAN_POINT('',(141.,-8.62670273047588,7.63675323681471));
#78990=CARTESIAN_POINT('',(141.,-8.06101730552664,7.63675323681471));
#78991=CARTESIAN_POINT('Origin',(159.,12.,0.));
#78992=CARTESIAN_POINT('',(159.,-7.63675323681471,8.06101730552664));
#78993=CARTESIAN_POINT('',(159.,-8.34386001800126,7.35391052434009));
#78994=CARTESIAN_POINT('',(159.,-7.63675323681471,8.62670273047588));
#78995=CARTESIAN_POINT('Origin',(159.,-7.91959594928933,8.34386001800126));
#78996=CARTESIAN_POINT('',(159.,-7.97585756174453,8.9658070554057));
#78997=CARTESIAN_POINT('',(159.,-7.35391052434009,8.34386001800126));
#78998=CARTESIAN_POINT('',(159.,-6.95077498280155,9.7819592689022));
#78999=CARTESIAN_POINT('Origin',(159.,0.,0.));
#79000=CARTESIAN_POINT('',(159.,-16.5536728370359,12.7583664943589));
#79001=CARTESIAN_POINT('Ctrl Pts',(159.,-16.5536728370359,12.7583664943589));
#79002=CARTESIAN_POINT('Ctrl Pts',(159.,-15.423567841049,11.6783667562433));
#79003=CARTESIAN_POINT('Ctrl Pts',(159.,-13.2082488270869,10.226020745615));
#79004=CARTESIAN_POINT('Ctrl Pts',(159.,-9.77882982348215,9.32502435050667));
#79005=CARTESIAN_POINT('Ctrl Pts',(159.,-7.80418402739541,9.49950253045326));
#79006=CARTESIAN_POINT('Ctrl Pts',(159.,-6.95092542742432,9.7824130125699));
#79007=CARTESIAN_POINT('',(159.,-19.325905913425,7.95671795563007));
#79008=CARTESIAN_POINT('Origin',(159.,-1.33226762955019E-14,0.));
#79009=CARTESIAN_POINT('',(159.,-11.9468127170547,1.12856807664439));
#79010=CARTESIAN_POINT('Ctrl Pts',(159.,-11.9472897183348,1.12846964567391));
#79011=CARTESIAN_POINT('Ctrl Pts',(159.,-12.1377264827052,2.05134558432588));
#79012=CARTESIAN_POINT('Ctrl Pts',(159.,-13.0341386662615,3.92229908516933));
#79013=CARTESIAN_POINT('Ctrl Pts',(159.,-15.5784481954706,6.39368319782361));
#79014=CARTESIAN_POINT('Ctrl Pts',(159.,-17.909806185795,7.54294547449438));
#79015=CARTESIAN_POINT('Ctrl Pts',(159.,-19.325893536257,7.95676028538056));
#79016=CARTESIAN_POINT('',(159.,-11.7525454562834,2.42439173773413));
#79017=CARTESIAN_POINT('Origin',(159.,0.,0.));
#79018=CARTESIAN_POINT('',(159.,-11.289320333896,2.30027094027664));
#79019=CARTESIAN_POINT('',(159.,-12.1586535775562,2.53320808086891));
#79020=CARTESIAN_POINT('',(159.,-10.7994223853394,2.58311365275126));
#79021=CARTESIAN_POINT('Origin',(159.,-11.185792715855,2.68664127079227));
#79022=CARTESIAN_POINT('',(159.,-10.6441309582779,3.1626691485247));
#79023=CARTESIAN_POINT('',(159.,-10.9029500033804,2.19674332223564));
#79024=CARTESIAN_POINT('',(159.,-10.9269736707525,3.65256709708134));
#79025=CARTESIAN_POINT('Origin',(159.,-11.0305012887935,3.26619676656571));
#79026=CARTESIAN_POINT('',(159.,-11.3901987931398,3.77668789453883));
#79027=CARTESIAN_POINT('',(159.,-10.5406033402369,3.54903947904033));
#79028=CARTESIAN_POINT('',(159.,-10.7246084263455,5.38356518503846));
#79029=CARTESIAN_POINT('Origin',(159.,0.,0.));
#79030=CARTESIAN_POINT('',(159.,-10.309292143521,5.1437822173509));
#79031=CARTESIAN_POINT('',(159.,-11.088715006927,5.5937822173509));
#79032=CARTESIAN_POINT('',(159.,-9.76288198200727,5.29019237886467));
#79033=CARTESIAN_POINT('Origin',(159.,-10.109292143521,5.49019237886467));
#79034=CARTESIAN_POINT('',(159.,-9.46288198200727,5.80980762113533));
#79035=CARTESIAN_POINT('',(159.,-9.96288198200727,4.9437822173509));
#79036=CARTESIAN_POINT('',(159.,-9.60929214352104,6.35621778264911));
#79037=CARTESIAN_POINT('Origin',(159.,-9.80929214352104,6.00980762113534));
#79038=CARTESIAN_POINT('',(159.,-10.0246084263455,6.59600075033667));
#79039=CARTESIAN_POINT('',(159.,-9.26288198200727,6.15621778264911));
#79040=CARTESIAN_POINT('',(159.,-8.9658070554057,7.97585756174453));
#79041=CARTESIAN_POINT('Origin',(159.,0.,0.));
#79042=CARTESIAN_POINT('',(159.,-9.26309883354377,8.27314933988261));
#79043=CARTESIAN_POINT('Origin',(141.,-8.34386001800126,7.35391052434009));
#79044=CARTESIAN_POINT('',(141.,-7.63675323681471,8.06101730552664));
#79045=CARTESIAN_POINT('Origin',(141.,-7.91959594928933,8.34386001800126));
#79046=CARTESIAN_POINT('',(141.,-7.63675323681471,8.62670273047588));
#79047=CARTESIAN_POINT('Origin',(141.,-9.80929214352104,6.00980762113534));
#79048=CARTESIAN_POINT('',(141.,-9.46288198200727,5.80980762113533));
#79049=CARTESIAN_POINT('',(141.,-9.60929214352104,6.35621778264911));
#79050=CARTESIAN_POINT('Origin',(141.,-9.26288198200727,6.15621778264911));
#79051=CARTESIAN_POINT('',(150.,-10.0246084263455,6.59600075033667));
#79052=CARTESIAN_POINT('Origin',(141.,-10.109292143521,5.49019237886467));
#79053=CARTESIAN_POINT('',(141.,-10.309292143521,5.1437822173509));
#79054=CARTESIAN_POINT('',(141.,-9.76288198200727,5.29019237886467));
#79055=CARTESIAN_POINT('Origin',(141.,-11.088715006927,5.5937822173509));
#79056=CARTESIAN_POINT('',(150.,-10.7246084263455,5.38356518503846));
#79057=CARTESIAN_POINT('Origin',(141.,-11.0305012887935,3.26619676656571));
#79058=CARTESIAN_POINT('',(141.,-10.6441309582779,3.1626691485247));
#79059=CARTESIAN_POINT('',(141.,-10.9269736707525,3.65256709708134));
#79060=CARTESIAN_POINT('Origin',(141.,-10.5406033402369,3.54903947904033));
#79061=CARTESIAN_POINT('',(150.,-11.3901987931398,3.77668789453883));
#79062=CARTESIAN_POINT('Origin',(141.,-11.185792715855,2.68664127079227));
#79063=CARTESIAN_POINT('',(141.,-11.289320333896,2.30027094027664));
#79064=CARTESIAN_POINT('',(141.,-10.7994223853394,2.58311365275126));
#79065=CARTESIAN_POINT('Origin',(141.,-12.1586535775562,2.53320808086891));
#79066=CARTESIAN_POINT('',(150.,-11.7525454562834,2.42439173773413));
#79067=CARTESIAN_POINT('Origin',(141.,-11.5,0.300000000000001));
#79068=CARTESIAN_POINT('',(159.,-11.5,0.700000000000001));
#79069=CARTESIAN_POINT('',(159.,-11.1,0.300000000000001));
#79070=CARTESIAN_POINT('Origin',(159.,-11.5,0.300000000000001));
#79071=CARTESIAN_POINT('',(141.,-11.1,0.300000000000001));
#79072=CARTESIAN_POINT('',(141.,-11.5,0.700000000000001));
#79073=CARTESIAN_POINT('Origin',(141.,-11.1,0.700000000000001));
#79074=CARTESIAN_POINT('',(158.9865805553,-11.9795659353751,0.700000000000002));
#79075=CARTESIAN_POINT('',(150.,-11.9795659353751,0.700000000000002));
#79076=CARTESIAN_POINT('',(158.90010356288,-12.1426591968742,0.699999999999098));
#79077=CARTESIAN_POINT('Ctrl Pts',(158.986559794035,-11.9795632850285,0.70000034124336));
#79078=CARTESIAN_POINT('Ctrl Pts',(158.983092985643,-11.9927290439857,0.700000368005176));
#79079=CARTESIAN_POINT('Ctrl Pts',(158.978970927741,-12.0057044345014,0.700000397309329));
#79080=CARTESIAN_POINT('Ctrl Pts',(158.974202995356,-12.0184378742667,0.700000533998414));
#79081=CARTESIAN_POINT('Ctrl Pts',(158.968537668188,-12.0335679340913,0.70000069641439));
#79082=CARTESIAN_POINT('Ctrl Pts',(158.96196068147,-12.0483567216063,0.700000957224616));
#79083=CARTESIAN_POINT('Ctrl Pts',(158.954513252864,-12.0627266959769,0.700000963176014));
#79084=CARTESIAN_POINT('Ctrl Pts',(158.94418889197,-12.082647773346,0.700000971426428));
#79085=CARTESIAN_POINT('Ctrl Pts',(158.932243096067,-12.1016692830454,0.700000125593032));
#79086=CARTESIAN_POINT('Ctrl Pts',(158.918794292536,-12.1195876530581,0.699998810214279));
#79087=CARTESIAN_POINT('Ctrl Pts',(158.912855160605,-12.1275005921719,0.6999982293293));
#79088=CARTESIAN_POINT('Ctrl Pts',(158.906622332495,-12.1351980550098,0.699997625884581));
#79089=CARTESIAN_POINT('Ctrl Pts',(158.90010351009,-12.142660453513,0.699997406838469));
#79090=CARTESIAN_POINT('',(158.671029640456,-12.4,0.700000000000002));
#79091=CARTESIAN_POINT('Origin',(145.,-4.46675525190797E-15,0.7));
#79092=CARTESIAN_POINT('',(159.,-12.4,0.700000000000002));
#79093=CARTESIAN_POINT('',(141.,-12.4,0.700000000000002));
#79094=CARTESIAN_POINT('',(159.,-11.1,0.700000000000001));
#79095=CARTESIAN_POINT('Origin',(141.,-11.5,-0.299999999999998));
#79096=CARTESIAN_POINT('',(159.,-11.1,-0.299999999999998));
#79097=CARTESIAN_POINT('',(159.,-11.5,-0.699999999999999));
#79098=CARTESIAN_POINT('Origin',(159.,-11.5,-0.299999999999998));
#79099=CARTESIAN_POINT('',(141.,-11.5,-0.699999999999999));
#79100=CARTESIAN_POINT('',(141.,-11.1,-0.299999999999998));
#79101=CARTESIAN_POINT('Origin',(141.,-12.4,-0.699999999999998));
#79102=CARTESIAN_POINT('',(159.,-12.4,-0.699999999999998));
#79103=CARTESIAN_POINT('',(159.,-0.2,-0.7));
#79104=CARTESIAN_POINT('',(158.671029640456,-12.4,-0.699999999999998));
#79105=CARTESIAN_POINT('',(141.,-12.4,-0.699999999999998));
#79106=CARTESIAN_POINT('',(158.90010356288,-12.1426591968742,-0.699999999999095));
#79107=CARTESIAN_POINT('Origin',(145.,-4.64630030125423E-15,-0.7));
#79108=CARTESIAN_POINT('',(158.9865805553,-11.9795659353751,-0.699999999999998));
#79109=CARTESIAN_POINT('Ctrl Pts',(158.900103509945,-12.1426604728543,-0.69999760074457));
#79110=CARTESIAN_POINT('Ctrl Pts',(158.914773977722,-12.1258665032419,-0.699998054035066));
#79111=CARTESIAN_POINT('Ctrl Pts',(158.927981161929,-12.1079043488789,-0.700000541470431));
#79112=CARTESIAN_POINT('Ctrl Pts',(158.939637604677,-12.0889945541585,-0.700001292268434));
#79113=CARTESIAN_POINT('Ctrl Pts',(158.951366856424,-12.0699666442236,-0.700002047756106));
#79114=CARTESIAN_POINT('Ctrl Pts',(158.96152669892,-12.0499780272482,-0.700001173353097));
#79115=CARTESIAN_POINT('Ctrl Pts',(158.969986244937,-12.0292239544123,-0.700000587878722));
#79116=CARTESIAN_POINT('Ctrl Pts',(158.971442590703,-12.0256510551061,-0.700000487086892));
#79117=CARTESIAN_POINT('Ctrl Pts',(158.972848428754,-12.0220554248935,-0.700000405865112));
#79118=CARTESIAN_POINT('Ctrl Pts',(158.974202940878,-12.018438012829,-0.700000366731693));
#79119=CARTESIAN_POINT('Ctrl Pts',(158.97898110036,-12.0056772767285,-0.700000228685149));
#79120=CARTESIAN_POINT('Ctrl Pts',(158.983100399885,-11.9927008953148,-0.700000282335582));
#79121=CARTESIAN_POINT('Ctrl Pts',(158.98655979805,-11.9795632865321,-0.70000034104977));
#79122=CARTESIAN_POINT('',(150.,-11.9795659353751,-0.699999999999998));
#79123=CARTESIAN_POINT('Origin',(159.,12.,0.));
#79124=CARTESIAN_POINT('',(159.,-12.4,0.700000000000002));
#79125=CARTESIAN_POINT('',(159.,-11.1,-0.699999999999999));
#79126=CARTESIAN_POINT('Origin',(141.,-11.0305012887935,-3.2661967665657));
#79127=CARTESIAN_POINT('',(159.,-10.6441309582779,-3.1626691485247));
#79128=CARTESIAN_POINT('',(159.,-10.9269736707525,-3.65256709708133));
#79129=CARTESIAN_POINT('Origin',(159.,-11.0305012887935,-3.2661967665657));
#79130=CARTESIAN_POINT('',(141.,-10.9269736707525,-3.65256709708133));
#79131=CARTESIAN_POINT('',(141.,-10.6441309582779,-3.1626691485247));
#79132=CARTESIAN_POINT('Origin',(159.,12.,0.));
#79133=CARTESIAN_POINT('',(159.,-10.7994223853394,-2.58311365275126));
#79134=CARTESIAN_POINT('',(159.,-10.5406033402369,-3.54903947904032));
#79135=CARTESIAN_POINT('',(159.,-11.2893203338961,-2.30027094027664));
#79136=CARTESIAN_POINT('Origin',(159.,-11.185792715855,-2.68664127079226));
#79137=CARTESIAN_POINT('',(159.,-11.7525454562834,-2.42439173773412));
#79138=CARTESIAN_POINT('',(159.,-10.9029500033804,-2.19674332223563));
#79139=CARTESIAN_POINT('',(159.,-11.9468127170547,-1.12856807664441));
#79140=CARTESIAN_POINT('Origin',(159.,0.,0.));
#79141=CARTESIAN_POINT('',(159.,-19.325905913425,-7.95671795563007));
#79142=CARTESIAN_POINT('Ctrl Pts',(159.,-19.325905913425,-7.95671795563007));
#79143=CARTESIAN_POINT('Ctrl Pts',(159.,-17.8256365211145,-7.51804459699146));
#79144=CARTESIAN_POINT('Ctrl Pts',(159.,-15.4601181289741,-6.3256760822434));
#79145=CARTESIAN_POINT('Ctrl Pts',(159.,-12.9651541198957,-3.80622087996466));
#79146=CARTESIAN_POINT('Ctrl Pts',(159.,-12.1289065769249,-2.00887379866001));
#79147=CARTESIAN_POINT('Ctrl Pts',(159.,-11.9472815380172,-1.1284713591759));
#79148=CARTESIAN_POINT('',(159.,-16.5536728370359,-12.7583664943589));
#79149=CARTESIAN_POINT('Origin',(159.,-1.33226762955019E-14,0.));
#79150=CARTESIAN_POINT('',(159.,-6.95077498280155,-9.7819592689022));
#79151=CARTESIAN_POINT('Ctrl Pts',(159.,-6.95092542742433,-9.7824130125699));
#79152=CARTESIAN_POINT('Ctrl Pts',(159.,-7.80418402739543,-9.49950253045326));
#79153=CARTESIAN_POINT('Ctrl Pts',(159.,-9.77882982348219,-9.32502435050667));
#79154=CARTESIAN_POINT('Ctrl Pts',(159.,-13.2082488270869,-10.226020745615));
#79155=CARTESIAN_POINT('Ctrl Pts',(159.,-15.423567841049,-11.6783667562432));
#79156=CARTESIAN_POINT('Ctrl Pts',(159.,-16.5536728370359,-12.7583664943589));
#79157=CARTESIAN_POINT('',(159.,-7.97585756174453,-8.96580705540569));
#79158=CARTESIAN_POINT('Origin',(159.,0.,0.));
#79159=CARTESIAN_POINT('',(159.,-7.63675323681472,-8.62670273047588));
#79160=CARTESIAN_POINT('',(159.,-8.27314933988261,-9.26309883354377));
#79161=CARTESIAN_POINT('',(159.,-7.63675323681472,-8.06101730552664));
#79162=CARTESIAN_POINT('Origin',(159.,-7.91959594928934,-8.34386001800125));
#79163=CARTESIAN_POINT('',(159.,-8.06101730552665,-7.63675323681471));
#79164=CARTESIAN_POINT('',(159.,-7.3539105243401,-8.34386001800125));
#79165=CARTESIAN_POINT('',(159.,-8.62670273047588,-7.63675323681471));
#79166=CARTESIAN_POINT('Origin',(159.,-8.34386001800126,-7.91959594928933));
#79167=CARTESIAN_POINT('',(159.,-8.9658070554057,-7.97585756174453));
#79168=CARTESIAN_POINT('',(159.,-8.34386001800126,-7.35391052434009));
#79169=CARTESIAN_POINT('',(159.,-10.0246084263455,-6.59600075033666));
#79170=CARTESIAN_POINT('Origin',(159.,0.,0.));
#79171=CARTESIAN_POINT('',(159.,-9.60929214352105,-6.3562177826491));
#79172=CARTESIAN_POINT('',(159.,-10.388715006927,-6.8062177826491));
#79173=CARTESIAN_POINT('',(159.,-9.46288198200727,-5.80980762113533));
#79174=CARTESIAN_POINT('Origin',(159.,-9.80929214352104,-6.00980762113533));
#79175=CARTESIAN_POINT('',(159.,-9.76288198200727,-5.29019237886466));
#79176=CARTESIAN_POINT('',(159.,-9.26288198200727,-6.1562177826491));
#79177=CARTESIAN_POINT('',(159.,-10.309292143521,-5.14378221735089));
#79178=CARTESIAN_POINT('Origin',(159.,-10.109292143521,-5.49019237886466));
#79179=CARTESIAN_POINT('',(159.,-10.7246084263455,-5.38356518503845));
#79180=CARTESIAN_POINT('',(159.,-9.96288198200727,-4.94378221735089));
#79181=CARTESIAN_POINT('',(159.,-11.3901987931398,-3.77668789453882));
#79182=CARTESIAN_POINT('Origin',(159.,0.,0.));
#79183=CARTESIAN_POINT('',(159.,-11.7963069144127,-3.8855042376736));
#79184=CARTESIAN_POINT('Origin',(141.,-10.5406033402369,-3.54903947904032));
#79185=CARTESIAN_POINT('',(141.,-10.7994223853394,-2.58311365275126));
#79186=CARTESIAN_POINT('Origin',(141.,-11.185792715855,-2.68664127079226));
#79187=CARTESIAN_POINT('',(141.,-11.2893203338961,-2.30027094027664));
#79188=CARTESIAN_POINT('Origin',(141.,-10.109292143521,-5.49019237886466));
#79189=CARTESIAN_POINT('',(141.,-9.76288198200727,-5.29019237886466));
#79190=CARTESIAN_POINT('',(141.,-10.309292143521,-5.14378221735089));
#79191=CARTESIAN_POINT('Origin',(141.,-9.96288198200727,-4.94378221735089));
#79192=CARTESIAN_POINT('',(150.,-10.7246084263455,-5.38356518503845));
#79193=CARTESIAN_POINT('Origin',(141.,-9.80929214352104,-6.00980762113533));
#79194=CARTESIAN_POINT('',(141.,-9.60929214352105,-6.3562177826491));
#79195=CARTESIAN_POINT('',(141.,-9.46288198200727,-5.80980762113533));
#79196=CARTESIAN_POINT('Origin',(141.,-10.388715006927,-6.8062177826491));
#79197=CARTESIAN_POINT('',(150.,-10.0246084263455,-6.59600075033666));
#79198=CARTESIAN_POINT('Origin',(141.,-8.34386001800126,-7.91959594928933));
#79199=CARTESIAN_POINT('',(141.,-8.06101730552665,-7.63675323681471));
#79200=CARTESIAN_POINT('',(141.,-8.62670273047588,-7.63675323681471));
#79201=CARTESIAN_POINT('Origin',(141.,-8.34386001800126,-7.35391052434009));
#79202=CARTESIAN_POINT('',(150.,-8.9658070554057,-7.97585756174453));
#79203=CARTESIAN_POINT('Origin',(141.,-7.91959594928934,-8.34386001800125));
#79204=CARTESIAN_POINT('',(141.,-7.63675323681472,-8.62670273047588));
#79205=CARTESIAN_POINT('',(141.,-7.63675323681472,-8.06101730552664));
#79206=CARTESIAN_POINT('Origin',(141.,-8.27314933988261,-9.26309883354377));
#79207=CARTESIAN_POINT('',(150.,-7.97585756174453,-8.96580705540569));
#79208=CARTESIAN_POINT('Origin',(141.,-6.00980762113534,-9.80929214352104));
#79209=CARTESIAN_POINT('',(159.,-6.35621778264911,-9.60929214352104));
#79210=CARTESIAN_POINT('',(159.,-5.80980762113534,-9.46288198200726));
#79211=CARTESIAN_POINT('Origin',(159.,-6.00980762113534,-9.80929214352104));
#79212=CARTESIAN_POINT('',(141.,-5.80980762113534,-9.46288198200726));
#79213=CARTESIAN_POINT('',(141.,-6.35621778264911,-9.60929214352104));
#79214=CARTESIAN_POINT('Origin',(141.,-6.15621778264911,-9.26288198200726));
#79215=CARTESIAN_POINT('',(158.9865805553,-6.59600075033667,-10.0246084263455));
#79216=CARTESIAN_POINT('',(150.,-6.59600075033667,-10.0246084263455));
#79217=CARTESIAN_POINT('',(158.90010356288,-6.67754738108544,-10.1658513339903));
#79218=CARTESIAN_POINT('Ctrl Pts',(158.986559783722,-6.59599971918857,-10.0246059568635));
#79219=CARTESIAN_POINT('Ctrl Pts',(158.983100403821,-6.60256843395615,-10.0359834218172));
#79220=CARTESIAN_POINT('Ctrl Pts',(158.978981130879,-6.60905654044642,-10.0472212590995));
#79221=CARTESIAN_POINT('Ctrl Pts',(158.974203007079,-6.61543699190687,-10.0582722491853));
#79222=CARTESIAN_POINT('Ctrl Pts',(158.966341570957,-6.62593473405228,-10.0764544178127));
#79223=CARTESIAN_POINT('Ctrl Pts',(158.956755276001,-6.6360671734963,-10.0940017110895));
#79224=CARTESIAN_POINT('Ctrl Pts',(158.945583009388,-6.64573620403147,-10.1107496127459));
#79225=CARTESIAN_POINT('Ctrl Pts',(158.934457797467,-6.65536451111544,-10.1274269765802));
#79226=CARTESIAN_POINT('Ctrl Pts',(158.921759191497,-6.66453378582627,-10.1433127600987));
#79227=CARTESIAN_POINT('Ctrl Pts',(158.907581310124,-6.67313882951024,-10.1582194335506));
#79228=CARTESIAN_POINT('Ctrl Pts',(158.905132791899,-6.67462491940813,-10.1607938140699));
#79229=CARTESIAN_POINT('Ctrl Pts',(158.902640065462,-6.67609415059741,-10.1633389084977));
#79230=CARTESIAN_POINT('Ctrl Pts',(158.900103510001,-6.67754593940626,-10.1658536372963));
#79231=CARTESIAN_POINT('',(158.671029640456,-6.80621778264911,-10.388715006927));
#79232=CARTESIAN_POINT('Origin',(145.,-0.606217782649109,0.349999999999996));
#79233=CARTESIAN_POINT('',(159.,-6.80621778264911,-10.388715006927));
#79234=CARTESIAN_POINT('',(141.,-6.80621778264911,-10.388715006927));
#79235=CARTESIAN_POINT('',(159.,-6.15621778264911,-9.26288198200726));
#79236=CARTESIAN_POINT('Origin',(141.,-5.49019237886467,-10.109292143521));
#79237=CARTESIAN_POINT('',(159.,-5.29019237886467,-9.76288198200726));
#79238=CARTESIAN_POINT('',(159.,-5.1437822173509,-10.309292143521));
#79239=CARTESIAN_POINT('Origin',(159.,-5.49019237886467,-10.109292143521));
#79240=CARTESIAN_POINT('',(141.,-5.1437822173509,-10.309292143521));
#79241=CARTESIAN_POINT('',(141.,-5.29019237886467,-9.76288198200726));
#79242=CARTESIAN_POINT('Origin',(141.,-5.5937822173509,-11.088715006927));
#79243=CARTESIAN_POINT('',(159.,-5.5937822173509,-11.088715006927));
#79244=CARTESIAN_POINT('',(159.,-0.993782217350893,-3.1212812921102));
#79245=CARTESIAN_POINT('',(158.671029640456,-5.5937822173509,-11.088715006927));
#79246=CARTESIAN_POINT('',(141.,-5.5937822173509,-11.088715006927));
#79247=CARTESIAN_POINT('',(158.90010356288,-5.46511181578902,-10.8658513339891));
#79248=CARTESIAN_POINT('Origin',(145.,0.606217782649103,-0.350000000000003));
#79249=CARTESIAN_POINT('',(158.9865805553,-5.38356518503846,-10.7246084263455));
#79250=CARTESIAN_POINT('Ctrl Pts',(158.900103547043,-5.46511172210221,-10.8658524499821));
#79251=CARTESIAN_POINT('Ctrl Pts',(158.914774492576,-5.45671463864709,-10.8513079345424));
#79252=CARTESIAN_POINT('Ctrl Pts',(158.927982071263,-5.44773161925394,-10.8357527130695));
#79253=CARTESIAN_POINT('Ctrl Pts',(158.939638804435,-5.43827616198394,-10.8193759328616));
#79254=CARTESIAN_POINT('Ctrl Pts',(158.951368187913,-5.42876177380632,-10.8028970847692));
#79255=CARTESIAN_POINT('Ctrl Pts',(158.961528099835,-5.41876833333645,-10.7855854378059));
#79256=CARTESIAN_POINT('Ctrl Pts',(158.969987634148,-5.40839177230826,-10.7676110674777));
#79257=CARTESIAN_POINT('Ctrl Pts',(158.971443507408,-5.40660598160524,-10.7645177051067));
#79258=CARTESIAN_POINT('Ctrl Pts',(158.97284890317,-5.40480881166948,-10.7614046807561));
#79259=CARTESIAN_POINT('Ctrl Pts',(158.974203003918,-5.40300071696492,-10.7582728268913));
#79260=CARTESIAN_POINT('Ctrl Pts',(158.978981150563,-5.39662058486286,-10.7472216129632));
#79261=CARTESIAN_POINT('Ctrl Pts',(158.983100437627,-5.39013241397558,-10.7359837622487));
#79262=CARTESIAN_POINT('Ctrl Pts',(158.986559824909,-5.38356357140904,-10.7246063109672));
#79263=CARTESIAN_POINT('',(150.,-5.38356518503846,-10.7246084263455));
#79264=CARTESIAN_POINT('Origin',(159.,12.,0.));
#79265=CARTESIAN_POINT('',(159.,-6.80621778264911,-10.388715006927));
#79266=CARTESIAN_POINT('',(159.,-4.9437822173509,-9.96288198200727));
#79267=CARTESIAN_POINT('Origin',(141.,-2.68664127079228,-11.185792715855));
#79268=CARTESIAN_POINT('',(159.,-2.58311365275127,-10.7994223853394));
#79269=CARTESIAN_POINT('',(159.,-2.30027094027665,-11.289320333896));
#79270=CARTESIAN_POINT('Origin',(159.,-2.68664127079228,-11.185792715855));
#79271=CARTESIAN_POINT('',(141.,-2.30027094027665,-11.289320333896));
#79272=CARTESIAN_POINT('',(141.,-2.58311365275127,-10.7994223853394));
#79273=CARTESIAN_POINT('Origin',(159.,12.,0.));
#79274=CARTESIAN_POINT('',(159.,-3.16266914852471,-10.6441309582779));
#79275=CARTESIAN_POINT('',(159.,-2.19674332223564,-10.9029500033804));
#79276=CARTESIAN_POINT('',(159.,-3.65256709708134,-10.9269736707525));
#79277=CARTESIAN_POINT('Origin',(159.,-3.26619676656572,-11.0305012887935));
#79278=CARTESIAN_POINT('',(159.,-3.77668789453883,-11.3901987931398));
#79279=CARTESIAN_POINT('',(159.,-3.54903947904034,-10.5406033402369));
#79280=CARTESIAN_POINT('',(159.,-4.99603773425309,-10.9105273455467));
#79281=CARTESIAN_POINT('Origin',(159.,0.,0.));
#79282=CARTESIAN_POINT('',(159.,-2.77223307638909,-20.715084449989));
#79283=CARTESIAN_POINT('Ctrl Pts',(159.,-2.77223307638909,-20.715084449989));
#79284=CARTESIAN_POINT('Ctrl Pts',(159.,-2.27857807033076,-18.6902253726123));
#79285=CARTESIAN_POINT('Ctrl Pts',(159.,-2.25665265374671,-15.4594257282765));
#79286=CARTESIAN_POINT('Ctrl Pts',(159.,-3.73546525438224,-12.2142250696204));
#79287=CARTESIAN_POINT('Ctrl Pts',(159.,-4.71092906162781,-11.1635784596492));
#79288=CARTESIAN_POINT('Ctrl Pts',(159.,-4.9961448774954,-10.9106481653666));
#79289=CARTESIAN_POINT('',(159.,2.77223307638906,-20.715084449989));
#79290=CARTESIAN_POINT('Origin',(159.,-1.33226762955019E-14,0.));
#79291=CARTESIAN_POINT('',(159.,4.996037734253,-10.9105273455467));
#79292=CARTESIAN_POINT('Ctrl Pts',(159.,4.99635577373304,-10.9108848512975));
#79293=CARTESIAN_POINT('Ctrl Pts',(159.,4.32472250848347,-11.5083723707476));
#79294=CARTESIAN_POINT('Ctrl Pts',(159.,3.1862921761307,-13.1312444431996));
#79295=CARTESIAN_POINT('Ctrl Pts',(159.,2.25185337892959,-16.5517472098717));
#79296=CARTESIAN_POINT('Ctrl Pts',(159.,2.40199310172352,-19.1964453917219));
#79297=CARTESIAN_POINT('Ctrl Pts',(159.,2.77223307638906,-20.715084449989));
#79298=CARTESIAN_POINT('',(159.,3.77668789453882,-11.3901987931398));
#79299=CARTESIAN_POINT('Origin',(159.,0.,0.));
#79300=CARTESIAN_POINT('',(159.,3.65256709708133,-10.9269736707525));
#79301=CARTESIAN_POINT('',(159.,3.8855042376736,-11.7963069144127));
#79302=CARTESIAN_POINT('',(159.,3.1626691485247,-10.6441309582779));
#79303=CARTESIAN_POINT('Origin',(159.,3.2661967665657,-11.0305012887935));
#79304=CARTESIAN_POINT('',(159.,2.58311365275125,-10.7994223853394));
#79305=CARTESIAN_POINT('',(159.,3.54903947904032,-10.5406033402369));
#79306=CARTESIAN_POINT('',(159.,2.30027094027664,-11.2893203338961));
#79307=CARTESIAN_POINT('Origin',(159.,2.68664127079226,-11.185792715855));
#79308=CARTESIAN_POINT('',(159.,2.42439173773412,-11.7525454562834));
#79309=CARTESIAN_POINT('',(159.,2.19674332223563,-10.9029500033804));
#79310=CARTESIAN_POINT('',(159.,0.699999999999998,-11.9795659353751));
#79311=CARTESIAN_POINT('Origin',(159.,0.,0.));
#79312=CARTESIAN_POINT('',(159.,0.699999999999998,-11.5));
#79313=CARTESIAN_POINT('',(159.,0.699999999999998,-12.4));
#79314=CARTESIAN_POINT('',(159.,0.299999999999998,-11.1));
#79315=CARTESIAN_POINT('Origin',(159.,0.299999999999998,-11.5));
#79316=CARTESIAN_POINT('',(159.,-0.300000000000002,-11.1));
#79317=CARTESIAN_POINT('',(159.,0.699999999999998,-11.1));
#79318=CARTESIAN_POINT('',(159.,-0.700000000000002,-11.5));
#79319=CARTESIAN_POINT('Origin',(159.,-0.300000000000002,-11.5));
#79320=CARTESIAN_POINT('',(159.,-0.700000000000002,-11.9795659353751));
#79321=CARTESIAN_POINT('',(159.,-0.700000000000002,-11.1));
#79322=CARTESIAN_POINT('',(159.,-2.42439173773414,-11.7525454562834));
#79323=CARTESIAN_POINT('Origin',(159.,0.,0.));
#79324=CARTESIAN_POINT('',(159.,-2.53320808086892,-12.1586535775562));
#79325=CARTESIAN_POINT('Origin',(141.,-2.19674332223564,-10.9029500033804));
#79326=CARTESIAN_POINT('',(141.,-3.16266914852471,-10.6441309582779));
#79327=CARTESIAN_POINT('Origin',(141.,-3.26619676656572,-11.0305012887935));
#79328=CARTESIAN_POINT('',(141.,-3.65256709708134,-10.9269736707525));
#79329=CARTESIAN_POINT('Origin',(141.,-0.300000000000002,-11.5));
#79330=CARTESIAN_POINT('',(141.,-0.300000000000002,-11.1));
#79331=CARTESIAN_POINT('',(141.,-0.700000000000002,-11.5));
#79332=CARTESIAN_POINT('Origin',(141.,-0.700000000000002,-11.1));
#79333=CARTESIAN_POINT('',(150.,-0.700000000000002,-11.9795659353751));
#79334=CARTESIAN_POINT('Origin',(141.,0.299999999999998,-11.5));
#79335=CARTESIAN_POINT('',(141.,0.699999999999998,-11.5));
#79336=CARTESIAN_POINT('',(141.,0.299999999999998,-11.1));
#79337=CARTESIAN_POINT('Origin',(141.,0.699999999999998,-12.4));
#79338=CARTESIAN_POINT('',(150.,0.699999999999998,-11.9795659353751));
#79339=CARTESIAN_POINT('Origin',(141.,2.68664127079226,-11.185792715855));
#79340=CARTESIAN_POINT('',(141.,2.58311365275125,-10.7994223853394));
#79341=CARTESIAN_POINT('',(141.,2.30027094027664,-11.2893203338961));
#79342=CARTESIAN_POINT('Origin',(141.,2.19674332223563,-10.9029500033804));
#79343=CARTESIAN_POINT('',(150.,2.42439173773412,-11.7525454562834));
#79344=CARTESIAN_POINT('Origin',(141.,3.2661967665657,-11.0305012887935));
#79345=CARTESIAN_POINT('',(141.,3.65256709708133,-10.9269736707525));
#79346=CARTESIAN_POINT('',(141.,3.1626691485247,-10.6441309582779));
#79347=CARTESIAN_POINT('Origin',(141.,3.8855042376736,-11.7963069144127));
#79348=CARTESIAN_POINT('',(150.,3.77668789453882,-11.3901987931398));
#79349=CARTESIAN_POINT('Origin',(141.,5.49019237886466,-10.109292143521));
#79350=CARTESIAN_POINT('',(159.,5.14378221735088,-10.309292143521));
#79351=CARTESIAN_POINT('',(159.,5.29019237886466,-9.76288198200727));
#79352=CARTESIAN_POINT('Origin',(159.,5.49019237886466,-10.109292143521));
#79353=CARTESIAN_POINT('',(141.,5.29019237886466,-9.76288198200727));
#79354=CARTESIAN_POINT('',(141.,5.14378221735088,-10.309292143521));
#79355=CARTESIAN_POINT('Origin',(141.,4.94378221735088,-9.96288198200727));
#79356=CARTESIAN_POINT('',(158.9865805553,5.38356518503844,-10.7246084263456));
#79357=CARTESIAN_POINT('',(150.,5.38356518503844,-10.7246084263456));
#79358=CARTESIAN_POINT('',(158.90010356288,5.46511181578919,-10.865851333989));
#79359=CARTESIAN_POINT('Ctrl Pts',(158.986559824909,5.38356357140901,-10.7246063109672));
#79360=CARTESIAN_POINT('Ctrl Pts',(158.983100454493,5.3901323819486,-10.7359837067761));
#79361=CARTESIAN_POINT('Ctrl Pts',(158.978981190712,5.39662057531156,-10.747221479738));
#79362=CARTESIAN_POINT('Ctrl Pts',(158.974203073473,5.40300078113434,-10.7582725963848));
#79363=CARTESIAN_POINT('Ctrl Pts',(158.966341639814,5.41349813025692,-10.7764549925109));
#79364=CARTESIAN_POINT('Ctrl Pts',(158.956755336441,5.42362831019785,-10.7940035864906));
#79365=CARTESIAN_POINT('Ctrl Pts',(158.945583060576,5.43329790108699,-10.8107511607416));
#79366=CARTESIAN_POINT('Ctrl Pts',(158.934457818847,5.44292678398894,-10.8274282294205));
#79367=CARTESIAN_POINT('Ctrl Pts',(158.92175917638,5.45209965266851,-10.8433119712718));
#79368=CARTESIAN_POINT('Ctrl Pts',(158.907581262213,5.46070670256199,-10.8582175186421));
#79369=CARTESIAN_POINT('Ctrl Pts',(158.905132759071,5.46219312633743,-10.8607916828762));
#79370=CARTESIAN_POINT('Ctrl Pts',(158.902640048576,5.46366261725136,-10.8633366044588));
#79371=CARTESIAN_POINT('Ctrl Pts',(158.900103509962,5.46511453225733,-10.8658512381826));
#79372=CARTESIAN_POINT('',(158.671029640456,5.59378221735088,-11.088715006927));
#79373=CARTESIAN_POINT('Origin',(145.,-0.606217782649104,-0.350000000000003));
#79374=CARTESIAN_POINT('',(159.,5.59378221735088,-11.088715006927));
#79375=CARTESIAN_POINT('',(141.,5.59378221735088,-11.088715006927));
#79376=CARTESIAN_POINT('',(159.,4.94378221735088,-9.96288198200727));
#79377=CARTESIAN_POINT('Origin',(141.,6.00980762113532,-9.80929214352105));
#79378=CARTESIAN_POINT('',(159.,5.80980762113532,-9.46288198200727));
#79379=CARTESIAN_POINT('',(159.,6.3562177826491,-9.60929214352105));
#79380=CARTESIAN_POINT('Origin',(159.,6.00980762113532,-9.80929214352105));
#79381=CARTESIAN_POINT('',(141.,6.3562177826491,-9.60929214352105));
#79382=CARTESIAN_POINT('',(141.,5.80980762113532,-9.46288198200727));
#79383=CARTESIAN_POINT('Origin',(141.,6.8062177826491,-10.388715006927));
#79384=CARTESIAN_POINT('',(159.,6.8062177826491,-10.388715006927));
#79385=CARTESIAN_POINT('',(159.,5.2062177826491,-7.61743371481684));
#79386=CARTESIAN_POINT('',(158.671029640456,6.8062177826491,-10.388715006927));
#79387=CARTESIAN_POINT('',(141.,6.8062177826491,-10.388715006927));
#79388=CARTESIAN_POINT('',(158.90010356288,6.67754738108543,-10.1658513339903));
#79389=CARTESIAN_POINT('Origin',(145.,0.60621778264911,0.349999999999996));
#79390=CARTESIAN_POINT('',(158.9865805553,6.59600075033666,-10.0246084263456));
#79391=CARTESIAN_POINT('Ctrl Pts',(158.900103540746,6.67754564938124,-10.1658529710382));
#79392=CARTESIAN_POINT('Ctrl Pts',(158.914774152864,6.66914902772228,-10.1513087288062));
#79393=CARTESIAN_POINT('Ctrl Pts',(158.927981450421,6.66017005788987,-10.1357517526872));
#79394=CARTESIAN_POINT('Ctrl Pts',(158.93963797463,6.65071574485167,-10.119374924506));
#79395=CARTESIAN_POINT('Ctrl Pts',(158.951367297619,6.64120238655755,-10.1028958177132));
#79396=CARTESIAN_POINT('Ctrl Pts',(158.961527181933,6.63120724474112,-10.0855854903495));
#79397=CARTESIAN_POINT('Ctrl Pts',(158.969986738622,6.62082960661215,-10.0676120757298));
#79398=CARTESIAN_POINT('Ctrl Pts',(158.971442914857,6.61904326359534,-10.0645182423069));
#79399=CARTESIAN_POINT('Ctrl Pts',(158.972848594337,6.61724557419846,-10.0614047170532));
#79400=CARTESIAN_POINT('Ctrl Pts',(158.974202959128,6.61543703228241,-10.0582723103369));
#79401=CARTESIAN_POINT('Ctrl Pts',(158.978981100772,6.60905657297234,-10.047221312061));
#79402=CARTESIAN_POINT('Ctrl Pts',(158.983100388343,6.60256845278364,-10.0359834539291));
#79403=CARTESIAN_POINT('Ctrl Pts',(158.986559779189,6.59599971852914,-10.0246059552843));
#79404=CARTESIAN_POINT('',(150.,6.59600075033666,-10.0246084263456));
#79405=CARTESIAN_POINT('Origin',(159.,12.,0.));
#79406=CARTESIAN_POINT('',(159.,5.59378221735088,-11.088715006927));
#79407=CARTESIAN_POINT('',(159.,6.1562177826491,-9.26288198200727));
#79408=CARTESIAN_POINT('Origin',(141.,8.34386001800126,-7.91959594928933));
#79409=CARTESIAN_POINT('',(159.,8.06101730552664,-7.63675323681472));
#79410=CARTESIAN_POINT('',(159.,8.62670273047588,-7.63675323681471));
#79411=CARTESIAN_POINT('Origin',(159.,8.34386001800126,-7.91959594928933));
#79412=CARTESIAN_POINT('',(141.,8.62670273047588,-7.63675323681471));
#79413=CARTESIAN_POINT('',(141.,8.06101730552664,-7.63675323681472));
#79414=CARTESIAN_POINT('Origin',(159.,12.,0.));
#79415=CARTESIAN_POINT('',(159.,7.63675323681471,-8.06101730552664));
#79416=CARTESIAN_POINT('',(159.,8.34386001800126,-7.35391052434009));
#79417=CARTESIAN_POINT('',(159.,7.63675323681471,-8.62670273047588));
#79418=CARTESIAN_POINT('Origin',(159.,7.91959594928933,-8.34386001800126));
#79419=CARTESIAN_POINT('',(159.,7.97585756174453,-8.9658070554057));
#79420=CARTESIAN_POINT('',(159.,7.35391052434009,-8.34386001800126));
#79421=CARTESIAN_POINT('',(159.,6.95077498280154,-9.78195926890221));
#79422=CARTESIAN_POINT('Origin',(159.,0.,0.));
#79423=CARTESIAN_POINT('',(159.,16.5536728370359,-12.7583664943589));
#79424=CARTESIAN_POINT('Ctrl Pts',(159.,16.5538196356257,-12.7582128920027));
#79425=CARTESIAN_POINT('Ctrl Pts',(159.,15.0944978202573,-11.3611439084094));
#79426=CARTESIAN_POINT('Ctrl Pts',(159.,12.816383606647,-10.0169387079855));
#79427=CARTESIAN_POINT('Ctrl Pts',(159.,9.35994040489882,-9.36183283938932));
#79428=CARTESIAN_POINT('Ctrl Pts',(159.,7.84517772049527,-9.48461709213552));
#79429=CARTESIAN_POINT('Ctrl Pts',(159.,6.95085137174832,-9.78218885206826));
#79430=CARTESIAN_POINT('',(159.,19.325905913425,-7.95671795563006));
#79431=CARTESIAN_POINT('Origin',(159.,-1.33226762955019E-14,0.));
#79432=CARTESIAN_POINT('',(159.,11.9468127170547,-1.12856807664441));
#79433=CARTESIAN_POINT('Ctrl Pts',(159.,11.9472897183348,-1.12846964567393));
#79434=CARTESIAN_POINT('Ctrl Pts',(159.,12.1377264827052,-2.05134558432589));
#79435=CARTESIAN_POINT('Ctrl Pts',(159.,13.0341386662615,-3.92229908516933));
#79436=CARTESIAN_POINT('Ctrl Pts',(159.,15.5784481954706,-6.3936831978236));
#79437=CARTESIAN_POINT('Ctrl Pts',(159.,17.909806185795,-7.54294547449437));
#79438=CARTESIAN_POINT('Ctrl Pts',(159.,19.325893536257,-7.95676028538055));
#79439=CARTESIAN_POINT('',(159.,11.7525454562834,-2.42439173773414));
#79440=CARTESIAN_POINT('Origin',(159.,0.,0.));
#79441=CARTESIAN_POINT('',(159.,11.289320333896,-2.30027094027665));
#79442=CARTESIAN_POINT('',(159.,12.1586535775562,-2.53320808086892));
#79443=CARTESIAN_POINT('',(159.,10.7994223853394,-2.58311365275127));
#79444=CARTESIAN_POINT('Origin',(159.,11.185792715855,-2.68664127079228));
#79445=CARTESIAN_POINT('',(159.,10.6441309582779,-3.16266914852471));
#79446=CARTESIAN_POINT('',(159.,10.9029500033804,-2.19674332223564));
#79447=CARTESIAN_POINT('',(159.,10.9269736707525,-3.65256709708134));
#79448=CARTESIAN_POINT('Origin',(159.,11.0305012887935,-3.26619676656572));
#79449=CARTESIAN_POINT('',(159.,11.3901987931398,-3.77668789453883));
#79450=CARTESIAN_POINT('',(159.,10.5406033402369,-3.54903947904034));
#79451=CARTESIAN_POINT('',(159.,10.7246084263455,-5.38356518503846));
#79452=CARTESIAN_POINT('Origin',(159.,0.,0.));
#79453=CARTESIAN_POINT('',(159.,10.309292143521,-5.1437822173509));
#79454=CARTESIAN_POINT('',(159.,11.088715006927,-5.5937822173509));
#79455=CARTESIAN_POINT('',(159.,9.76288198200726,-5.29019237886467));
#79456=CARTESIAN_POINT('Origin',(159.,10.109292143521,-5.49019237886467));
#79457=CARTESIAN_POINT('',(159.,9.46288198200726,-5.80980762113534));
#79458=CARTESIAN_POINT('',(159.,9.96288198200727,-4.9437822173509));
#79459=CARTESIAN_POINT('',(159.,9.60929214352104,-6.35621778264911));
#79460=CARTESIAN_POINT('Origin',(159.,9.80929214352104,-6.00980762113534));
#79461=CARTESIAN_POINT('',(159.,10.0246084263455,-6.59600075033667));
#79462=CARTESIAN_POINT('',(159.,9.26288198200726,-6.15621778264911));
#79463=CARTESIAN_POINT('',(159.,8.96580705540569,-7.97585756174453));
#79464=CARTESIAN_POINT('Origin',(159.,0.,0.));
#79465=CARTESIAN_POINT('',(159.,9.26309883354377,-8.27314933988261));
#79466=CARTESIAN_POINT('Origin',(141.,8.34386001800126,-7.35391052434009));
#79467=CARTESIAN_POINT('',(141.,7.63675323681471,-8.06101730552664));
#79468=CARTESIAN_POINT('Origin',(141.,7.91959594928933,-8.34386001800126));
#79469=CARTESIAN_POINT('',(141.,7.63675323681471,-8.62670273047588));
#79470=CARTESIAN_POINT('Origin',(141.,9.80929214352104,-6.00980762113534));
#79471=CARTESIAN_POINT('',(141.,9.46288198200726,-5.80980762113534));
#79472=CARTESIAN_POINT('',(141.,9.60929214352104,-6.35621778264911));
#79473=CARTESIAN_POINT('Origin',(141.,9.26288198200726,-6.15621778264911));
#79474=CARTESIAN_POINT('',(150.,10.0246084263455,-6.59600075033667));
#79475=CARTESIAN_POINT('Origin',(141.,10.109292143521,-5.49019237886467));
#79476=CARTESIAN_POINT('',(141.,10.309292143521,-5.1437822173509));
#79477=CARTESIAN_POINT('',(141.,9.76288198200726,-5.29019237886467));
#79478=CARTESIAN_POINT('Origin',(141.,11.088715006927,-5.5937822173509));
#79479=CARTESIAN_POINT('',(150.,10.7246084263455,-5.38356518503846));
#79480=CARTESIAN_POINT('Ctrl Pts',(158.677501178077,19.4360368307981,7.5800685849479));
#79481=CARTESIAN_POINT('Ctrl Pts',(156.381203869193,20.54678879986,7.43235132395997));
#79482=CARTESIAN_POINT('Ctrl Pts',(150.574304154338,22.2091125962063,6.9698415017293));
#79483=CARTESIAN_POINT('Ctrl Pts',(144.528109095534,21.4890932564754,6.16328954336132));
#79484=CARTESIAN_POINT('Ctrl Pts',(141.349059636028,20.3468534916255,5.57756265769612));
#79485=CARTESIAN_POINT('Ctrl Pts',(158.718387254562,19.5275359561361,7.61523551402801));
#79486=CARTESIAN_POINT('Ctrl Pts',(156.408397941026,20.6382004576914,7.47160753709084));
#79487=CARTESIAN_POINT('Ctrl Pts',(150.570403331328,22.2915836339626,7.01742228506264));
#79488=CARTESIAN_POINT('Ctrl Pts',(144.506261956165,21.5466300695078,6.21332634097748));
#79489=CARTESIAN_POINT('Ctrl Pts',(141.323496046579,20.3898842138692,5.62633961062338));
#79490=CARTESIAN_POINT('Ctrl Pts',(158.782431134995,19.6850146075886,7.76943529932877));
#79491=CARTESIAN_POINT('Ctrl Pts',(156.446860908445,20.7920792075557,7.62520489711286));
#79492=CARTESIAN_POINT('Ctrl Pts',(150.553817907369,22.4210857940526,7.16682494530977));
#79493=CARTESIAN_POINT('Ctrl Pts',(144.463812566537,21.6299226567777,6.34863932743448));
#79494=CARTESIAN_POINT('Ctrl Pts',(141.277191350935,20.4492386022585,5.74981169034822));
#79495=CARTESIAN_POINT('Ctrl Pts',(158.773699287394,19.699237028914,7.99834618950255));
#79496=CARTESIAN_POINT('Ctrl Pts',(156.432983097381,20.8042024238597,7.84408931627428));
#79497=CARTESIAN_POINT('Ctrl Pts',(150.529915338416,22.4257371082507,7.35943202981002));
#79498=CARTESIAN_POINT('Ctrl Pts',(144.438077279155,21.6247079944739,6.50990685306487));
#79499=CARTESIAN_POINT('Ctrl Pts',(141.252831675804,20.439567890367,5.89202809689228));
#79500=CARTESIAN_POINT('Ctrl Pts',(158.752212389358,19.6679573455318,8.09754482209984));
#79501=CARTESIAN_POINT('Ctrl Pts',(156.415119735441,20.7729290836719,7.93974319689782));
#79502=CARTESIAN_POINT('Ctrl Pts',(150.519347812546,22.3964776400354,7.44565874710652));
#79503=CARTESIAN_POINT('Ctrl Pts',(144.431524035377,21.6001740912567,6.58404508740874));
#79504=CARTESIAN_POINT('Ctrl Pts',(141.247787610619,20.4180572183914,5.95833178982708));
#79505=CARTESIAN_POINT('',(141.349059636028,20.3468534916255,5.57756265769611));
#79506=CARTESIAN_POINT('',(141.247787610619,20.4180572183914,5.95833178982708));
#79507=CARTESIAN_POINT('Origin',(141.4,20.0629605711151,5.85470862826487));
#79508=CARTESIAN_POINT('',(158.752212389369,19.6679573455318,8.09754482209984));
#79509=CARTESIAN_POINT('Ctrl Pts',(141.247787610619,20.4180572183914,5.95833178982708));
#79510=CARTESIAN_POINT('Ctrl Pts',(144.431524035377,21.6001740912567,6.58404508740874));
#79511=CARTESIAN_POINT('Ctrl Pts',(150.519347812546,22.3964776400354,7.44565874710652));
#79512=CARTESIAN_POINT('Ctrl Pts',(156.415119735441,20.7729290836719,7.93974319689782));
#79513=CARTESIAN_POINT('Ctrl Pts',(158.752212389358,19.6679573455318,8.09754482209984));
#79514=CARTESIAN_POINT('',(158.677501178088,19.4360368307978,7.58006858495009));
#79515=CARTESIAN_POINT('Origin',(158.599999999977,19.3259059134356,7.95671795562854));
#79516=CARTESIAN_POINT('Ctrl Pts',(158.677501178077,19.4360368307981,7.5800685849479));
#79517=CARTESIAN_POINT('Ctrl Pts',(156.381203869193,20.54678879986,7.43235132395997));
#79518=CARTESIAN_POINT('Ctrl Pts',(150.574304154338,22.2091125962063,6.9698415017293));
#79519=CARTESIAN_POINT('Ctrl Pts',(144.528109095534,21.4890932564754,6.16328954336132));
#79520=CARTESIAN_POINT('Ctrl Pts',(141.349059636028,20.3468534916255,5.57756265769612));
#79521=CARTESIAN_POINT('Origin',(158.6,19.325905913425,7.95671795563006));
#79522=CARTESIAN_POINT('Origin',(158.6,19.325905913425,7.95671795563006));
#79523=CARTESIAN_POINT('Origin',(158.6,19.325905913425,7.95671795563006));
#79524=CARTESIAN_POINT('Origin',(141.4,20.0629605711151,5.8547086282649));
#79525=CARTESIAN_POINT('Origin',(141.4,20.0629605711151,5.8547086282649));
#79526=CARTESIAN_POINT('Origin',(141.4,20.0629605711151,5.8547086282649));
#79527=CARTESIAN_POINT('Origin',(141.4,-1.33226762955019E-14,0.));
#79528=CARTESIAN_POINT('',(141.247787610619,15.3690953033624,14.7033903521377));
#79529=CARTESIAN_POINT('Origin',(141.4,15.1018066893949,14.4476792155747));
#79530=CARTESIAN_POINT('Origin',(141.247787610619,-1.33226762955019E-14,
0.));
#79531=CARTESIAN_POINT('Ctrl Pts',(141.349059636029,20.3468534916256,5.57756265769615));
#79532=CARTESIAN_POINT('Ctrl Pts',(141.334944065294,19.0862450920565,4.28886000353212));
#79533=CARTESIAN_POINT('Ctrl Pts',(141.315294799213,17.7320519040805,1.41692890345054));
#79534=CARTESIAN_POINT('Ctrl Pts',(141.323853738701,18.2994122920083,-2.86411526335879));
#79535=CARTESIAN_POINT('Ctrl Pts',(141.341466311039,19.6554156350548,-4.91714460851181));
#79536=CARTESIAN_POINT('Ctrl Pts',(141.35099653485,20.5213284072429,-5.75063643972609));
#79537=CARTESIAN_POINT('Ctrl Pts',(141.253636400131,20.338086471499,5.58612132234197));
#79538=CARTESIAN_POINT('Ctrl Pts',(141.242312365216,19.073415591963,4.29777681393181));
#79539=CARTESIAN_POINT('Ctrl Pts',(141.226869919812,17.7120787416654,1.42046269813161));
#79540=CARTESIAN_POINT('Ctrl Pts',(141.233574221952,18.2826163222716,-2.87109194893078));
#79541=CARTESIAN_POINT('Ctrl Pts',(141.247535627121,19.6445240874608,-4.92605388059928));
#79542=CARTESIAN_POINT('Ctrl Pts',(141.255191724905,20.5131188531463,-5.75914863555039));
#79543=CARTESIAN_POINT('Ctrl Pts',(141.072655152543,20.2690429983793,5.65352392024688));
#79544=CARTESIAN_POINT('Ctrl Pts',(141.068892342451,18.9878871037982,4.3512184780695));
#79545=CARTESIAN_POINT('Ctrl Pts',(141.063918977558,17.6071300866525,1.43898453555387));
#79546=CARTESIAN_POINT('Ctrl Pts',(141.066067920863,18.1859079098207,-2.90785906028693));
#79547=CARTESIAN_POINT('Ctrl Pts',(141.070620810551,19.5664939038525,-4.9863946813355));
#79548=CARTESIAN_POINT('Ctrl Pts',(141.073169850154,20.446341636345,-5.82838756610873));
#79549=CARTESIAN_POINT('Ctrl Pts',(141.,20.1318020119142,5.78750326121559));
#79550=CARTESIAN_POINT('Ctrl Pts',(141.00005964716,18.8243827965449,4.45167416745548));
#79551=CARTESIAN_POINT('Ctrl Pts',(141.000111472017,17.4192753208646,1.47114471514573));
#79552=CARTESIAN_POINT('Ctrl Pts',(141.000089306832,18.0079935750164,-2.97350659035009));
#79553=CARTESIAN_POINT('Ctrl Pts',(141.000040664939,19.4147163530666,-5.10302987964926));
#79554=CARTESIAN_POINT('Ctrl Pts',(141.,20.3127539068716,-5.96689995053429));
#79555=CARTESIAN_POINT('Ctrl Pts',(141.,20.0629605711151,5.8547086282649));
#79556=CARTESIAN_POINT('Ctrl Pts',(141.,18.7423719290453,4.50197105960825));
#79557=CARTESIAN_POINT('Ctrl Pts',(141.,17.325103889108,1.48733530859094));
#79558=CARTESIAN_POINT('Ctrl Pts',(141.,17.9187830382146,-3.00643154973687));
#79559=CARTESIAN_POINT('Ctrl Pts',(141.,19.3385812068509,-5.16147477539438));
#79560=CARTESIAN_POINT('Ctrl Pts',(141.,20.2457418776486,-6.03638234977459));
#79561=CARTESIAN_POINT('',(141.35099653485,20.5213284072429,-5.75063643972609));
#79562=CARTESIAN_POINT('Ctrl Pts',(141.349059636029,20.3468534916256,5.57756265769615));
#79563=CARTESIAN_POINT('Ctrl Pts',(141.334944065294,19.0862450920565,4.28886000353212));
#79564=CARTESIAN_POINT('Ctrl Pts',(141.315294799213,17.7320519040805,1.41692890345054));
#79565=CARTESIAN_POINT('Ctrl Pts',(141.323853738701,18.2994122920083,-2.86411526335879));
#79566=CARTESIAN_POINT('Ctrl Pts',(141.341466311039,19.6554156350548,-4.91714460851181));
#79567=CARTESIAN_POINT('Ctrl Pts',(141.35099653485,20.5213284072429,-5.75063643972609));
#79568=CARTESIAN_POINT('',(141.247787610619,20.4785660328527,-5.74692191779778));
#79569=CARTESIAN_POINT('Ctrl Pts',(141.35099653485,20.5213284072429,-5.75063643972609));
#79570=CARTESIAN_POINT('Ctrl Pts',(141.330560704654,20.5137748167918,-5.74685601366356));
#79571=CARTESIAN_POINT('Ctrl Pts',(141.310156580835,20.5056600402487,-5.74483779825721));
#79572=CARTESIAN_POINT('Ctrl Pts',(141.289961208009,20.4970792409922,-5.74467715710179));
#79573=CARTESIAN_POINT('Ctrl Pts',(141.275805268531,20.4910645327719,-5.74456455574041));
#79574=CARTESIAN_POINT('Ctrl Pts',(141.261752456281,20.4848204622714,-5.74536524920425));
#79575=CARTESIAN_POINT('Ctrl Pts',(141.247876796842,20.4783760618823,-5.74711947126434));
#79576=CARTESIAN_POINT('Ctrl Pts',(141.247876796842,20.4783760618823,-5.74711947126434));
#79577=CARTESIAN_POINT('Ctrl Pts',(141.228735529468,20.4694854666257,-5.74953877225964));
#79578=CARTESIAN_POINT('Ctrl Pts',(141.210454828721,20.4590667155478,-5.75235173741459));
#79579=CARTESIAN_POINT('Ctrl Pts',(141.193143805759,20.4473243089558,-5.75548786843929));
#79580=CARTESIAN_POINT('Ctrl Pts',(141.174820448736,20.4348952163033,-5.75880739776838));
#79581=CARTESIAN_POINT('Ctrl Pts',(141.157582524869,20.4209829410011,-5.76248903869804));
#79582=CARTESIAN_POINT('Ctrl Pts',(141.141550765423,20.4057898716458,-5.76648978816904));
#79583=CARTESIAN_POINT('Ctrl Pts',(141.13748945568,20.4019410264336,-5.76750329407009));
#79584=CARTESIAN_POINT('Ctrl Pts',(141.133505554007,20.3980098031508,-5.76853746952612));
#79585=CARTESIAN_POINT('Ctrl Pts',(141.129601061254,20.3939991380149,-5.76959198976122));
#79586=CARTESIAN_POINT('Ctrl Pts',(141.119160038773,20.3832741994654,-5.7724118872937));
#79587=CARTESIAN_POINT('Ctrl Pts',(141.109327541683,20.3720247222901,-5.77536706357361));
#79588=CARTESIAN_POINT('Ctrl Pts',(141.100132111297,20.3603105911578,-5.77844384099908));
#79589=CARTESIAN_POINT('Ctrl Pts',(141.086528119571,20.3429803590415,-5.78299571653738));
#79590=CARTESIAN_POINT('Ctrl Pts',(141.074316653251,20.3246348424351,-5.78781162882103));
#79591=CARTESIAN_POINT('Ctrl Pts',(141.063474024023,20.3055174940941,-5.79280132232444));
#79592=CARTESIAN_POINT('Ctrl Pts',(141.054045723591,20.2888938413038,-5.79714015273392));
#79593=CARTESIAN_POINT('Ctrl Pts',(141.045652621678,20.2716856939377,-5.80161136328767));
#79594=CARTESIAN_POINT('Ctrl Pts',(141.038293791978,20.2540354485553,-5.80617767088919));
#79595=CARTESIAN_POINT('Ctrl Pts',(141.029039527751,20.2318389796744,-5.81192013522221));
#79596=CARTESIAN_POINT('Ctrl Pts',(141.021438364409,20.2089860408799,-5.81779952711935));
#79597=CARTESIAN_POINT('Ctrl Pts',(141.015506370272,20.1857209999792,-5.82373720562914));
#79598=CARTESIAN_POINT('Ctrl Pts',(141.009416318352,20.1618360628539,-5.82983309338117));
#79599=CARTESIAN_POINT('Ctrl Pts',(141.005084928868,20.1375159088067,-5.8359912292933));
#79600=CARTESIAN_POINT('Ctrl Pts',(141.002571460327,20.1130064233281,-5.84215575124877));
#79601=CARTESIAN_POINT('Ctrl Pts',(141.000971072835,20.0974006286362,-5.84608085461723));
#79602=CARTESIAN_POINT('Ctrl Pts',(141.000108573519,20.0817177433566,-5.85000909601594));
#79603=CARTESIAN_POINT('Ctrl Pts',(141.000009602977,20.0660199650679,-5.85392963093109));
#79604=CARTESIAN_POINT('Ctrl Pts',(141.00000327861,20.0650168532613,-5.85418015904973));
#79605=CARTESIAN_POINT('Ctrl Pts',(141.000000075094,20.0640136905676,-5.85443064334051));
#79606=CARTESIAN_POINT('Ctrl Pts',(141.,20.0630104930043,-5.85468108040702));
#79607=CARTESIAN_POINT('Origin',(145.,4.5565277765811E-15,0.));
#79608=CARTESIAN_POINT('',(158.90010356288,12.1426591968742,0.699999999999097));
#79609=CARTESIAN_POINT('Ctrl Pts',(158.900103550553,12.1426600159095,0.699999891305436));
#79610=CARTESIAN_POINT('Ctrl Pts',(158.897779282747,12.2097338674886,1.18520292174833));
#79611=CARTESIAN_POINT('Ctrl Pts',(158.883475379338,12.6251819210183,2.63123643667199));
#79612=CARTESIAN_POINT('Ctrl Pts',(158.810748226743,14.7506827036296,5.50198934279456));
#79613=CARTESIAN_POINT('Ctrl Pts',(158.727432361316,17.4952316963631,7.02285824374443));
#79614=CARTESIAN_POINT('Ctrl Pts',(158.677501178099,19.4360368307974,7.58006858495228));
#79615=CARTESIAN_POINT('',(158.671029640456,12.4,0.7));
#79616=CARTESIAN_POINT('Origin',(145.,4.56057502531392E-15,0.7));
#79617=CARTESIAN_POINT('',(158.671029640456,12.4,-0.7));
#79618=CARTESIAN_POINT('Ctrl Pts',(158.671029640456,12.4,0.700000000000001));
#79619=CARTESIAN_POINT('Ctrl Pts',(158.642904819311,12.4,0.461338723738069));
#79620=CARTESIAN_POINT('Ctrl Pts',(158.629834412239,12.4,0.225792129208252));
#79621=CARTESIAN_POINT('Ctrl Pts',(158.629834412239,12.4,-0.225792129208251));
#79622=CARTESIAN_POINT('Ctrl Pts',(158.642904819311,12.4,-0.461338723738072));
#79623=CARTESIAN_POINT('Ctrl Pts',(158.671029640456,12.4,-0.700000000000001));
#79624=CARTESIAN_POINT('',(158.90010356288,12.1426591968742,-0.699999999999096));
#79625=CARTESIAN_POINT('Origin',(145.,4.55248052784828E-15,-0.7));
#79626=CARTESIAN_POINT('',(158.666552508001,19.866378214229,-7.69531573590556));
#79627=CARTESIAN_POINT('Ctrl Pts',(158.666552508001,19.8663782142289,-7.69531573590556));
#79628=CARTESIAN_POINT('Ctrl Pts',(158.70506309762,18.3356178296976,-7.31472446391732));
#79629=CARTESIAN_POINT('Ctrl Pts',(158.774612832515,15.8996513054051,-6.19397172155973));
#79630=CARTESIAN_POINT('Ctrl Pts',(158.863666938984,13.1911946894156,-3.64707236877049));
#79631=CARTESIAN_POINT('Ctrl Pts',(158.895220191772,12.283511760518,-1.71833536753633));
#79632=CARTESIAN_POINT('Ctrl Pts',(158.900103498665,12.1426607830635,-0.699999789453025));
#79633=CARTESIAN_POINT('Ctrl Pts',(141.35099653485,20.5213284072429,-5.75063643972609));
#79634=CARTESIAN_POINT('Ctrl Pts',(142.287870643948,20.8676203492237,-5.92394886527689));
#79635=CARTESIAN_POINT('Ctrl Pts',(143.328786142491,21.1776705740629,-6.09955485968982));
#79636=CARTESIAN_POINT('Ctrl Pts',(145.518850226888,21.6539319276962,-6.43375287746594));
#79637=CARTESIAN_POINT('Ctrl Pts',(146.670814422246,21.8087401867444,-6.59062276867075));
#79638=CARTESIAN_POINT('Ctrl Pts',(148.904844084702,21.9552803760224,-6.86857637330707));
#79639=CARTESIAN_POINT('Ctrl Pts',(150.200551186099,21.9423178409899,-7.01286833228401));
#79640=CARTESIAN_POINT('Ctrl Pts',(152.772096807936,21.6842975391536,-7.26584990074203));
#79641=CARTESIAN_POINT('Ctrl Pts',(154.047891554348,21.439140020175,-7.37488260408839));
#79642=CARTESIAN_POINT('Ctrl Pts',(156.319421579519,20.8197376369026,-7.54846485300653));
#79643=CARTESIAN_POINT('Ctrl Pts',(157.50927066846,20.3972306783393,-7.62820062110564));
#79644=CARTESIAN_POINT('Ctrl Pts',(158.666552508001,19.8663782142289,-7.69531573590556));
#79645=CARTESIAN_POINT('Ctrl Pts',(158.677501178099,-19.4360368307872,-7.58006858494935));
#79646=CARTESIAN_POINT('Ctrl Pts',(156.381203869213,-20.5467887998532,-7.43235132396155));
#79647=CARTESIAN_POINT('Ctrl Pts',(150.574304154351,-22.2091125962071,-6.96984150173096));
#79648=CARTESIAN_POINT('Ctrl Pts',(144.528109095539,-21.489093256477,-6.16328954336215));
#79649=CARTESIAN_POINT('Ctrl Pts',(141.349059636028,-20.3468534916256,-5.57756265769614));
#79650=CARTESIAN_POINT('Ctrl Pts',(158.718387254585,-19.5275359561253,-7.61523551402943));
#79651=CARTESIAN_POINT('Ctrl Pts',(156.408397941047,-20.6382004576847,-7.47160753709239));
#79652=CARTESIAN_POINT('Ctrl Pts',(150.570403331342,-22.2915836339634,-7.01742228506429));
#79653=CARTESIAN_POINT('Ctrl Pts',(144.50626195617,-21.5466300695094,-6.21332634097831));
#79654=CARTESIAN_POINT('Ctrl Pts',(141.323496046579,-20.3898842138693,-5.6263396106234));
#79655=CARTESIAN_POINT('Ctrl Pts',(158.782431135018,-19.6850146075777,-7.76943529933019));
#79656=CARTESIAN_POINT('Ctrl Pts',(156.446860908466,-20.7920792075491,-7.62520489711443));
#79657=CARTESIAN_POINT('Ctrl Pts',(150.553817907383,-22.4210857940535,-7.16682494531145));
#79658=CARTESIAN_POINT('Ctrl Pts',(144.463812566542,-21.6299226567794,-6.34863932743533));
#79659=CARTESIAN_POINT('Ctrl Pts',(141.277191350935,-20.4492386022585,-5.74981169034824));
#79660=CARTESIAN_POINT('Ctrl Pts',(158.773699287417,-19.6992370289032,-7.99834618950407));
#79661=CARTESIAN_POINT('Ctrl Pts',(156.432983097402,-20.8042024238531,-7.84408931627594));
#79662=CARTESIAN_POINT('Ctrl Pts',(150.52991533843,-22.4257371082516,-7.35943202981176));
#79663=CARTESIAN_POINT('Ctrl Pts',(144.438077279159,-21.6247079944755,-6.50990685306575));
#79664=CARTESIAN_POINT('Ctrl Pts',(141.252831675805,-20.439567890367,-5.8920280968923));
#79665=CARTESIAN_POINT('Ctrl Pts',(158.752212389381,-19.667957345521,-8.09754482210139));
#79666=CARTESIAN_POINT('Ctrl Pts',(156.415119735462,-20.7729290836652,-7.9397431968995));
#79667=CARTESIAN_POINT('Ctrl Pts',(150.519347812559,-22.3964776400363,-7.44565874710829));
#79668=CARTESIAN_POINT('Ctrl Pts',(144.431524035381,-21.6001740912584,-6.58404508740963));
#79669=CARTESIAN_POINT('Ctrl Pts',(141.247787610619,-20.4180572183915,-5.9583317898271));
#79670=CARTESIAN_POINT('',(141.349059636028,-20.3468534916256,-5.57756265769613));
#79671=CARTESIAN_POINT('',(141.247787610619,-20.4180572183915,-5.9583317898271));
#79672=CARTESIAN_POINT('Origin',(141.4,-20.0629605711151,-5.85470862826489));
#79673=CARTESIAN_POINT('',(158.752212389381,-19.667957345521,-8.09754482210139));
#79674=CARTESIAN_POINT('Ctrl Pts',(141.247787610619,-20.4180572183915,-5.9583317898271));
#79675=CARTESIAN_POINT('Ctrl Pts',(144.431524035381,-21.6001740912584,-6.58404508740963));
#79676=CARTESIAN_POINT('Ctrl Pts',(150.519347812559,-22.3964776400363,-7.44565874710829));
#79677=CARTESIAN_POINT('Ctrl Pts',(156.415119735462,-20.7729290836652,-7.9397431968995));
#79678=CARTESIAN_POINT('Ctrl Pts',(158.752212389381,-19.667957345521,-8.09754482210139));
#79679=CARTESIAN_POINT('',(158.677501178099,-19.4360368307872,-7.58006858494935));
#79680=CARTESIAN_POINT('Origin',(158.6,-19.325905913425,-7.95671795563007));
#79681=CARTESIAN_POINT('Ctrl Pts',(158.677501178099,-19.4360368307872,-7.58006858494935));
#79682=CARTESIAN_POINT('Ctrl Pts',(156.381203869213,-20.5467887998532,-7.43235132396155));
#79683=CARTESIAN_POINT('Ctrl Pts',(150.574304154351,-22.2091125962071,-6.96984150173096));
#79684=CARTESIAN_POINT('Ctrl Pts',(144.528109095539,-21.489093256477,-6.16328954336215));
#79685=CARTESIAN_POINT('Ctrl Pts',(141.349059636028,-20.3468534916256,-5.57756265769614));
#79686=CARTESIAN_POINT('Origin',(158.6,-19.325905913425,-7.95671795563007));
#79687=CARTESIAN_POINT('Origin',(158.6,-19.325905913425,-7.95671795563007));
#79688=CARTESIAN_POINT('Origin',(158.6,-19.325905913425,-7.95671795563007));
#79689=CARTESIAN_POINT('Origin',(141.4,-20.0629605711152,-5.85470862826492));
#79690=CARTESIAN_POINT('Origin',(141.4,-20.0629605711152,-5.85470862826492));
#79691=CARTESIAN_POINT('Origin',(141.4,-20.0629605711152,-5.85470862826492));
#79692=CARTESIAN_POINT('Ctrl Pts',(158.900200939034,-12.1398501039078,-0.679362733740278));
#79693=CARTESIAN_POINT('Ctrl Pts',(158.895624695094,-12.2718610342254,-1.6639602424403));
#79694=CARTESIAN_POINT('Ctrl Pts',(158.866156735235,-13.1195350868023,-3.5297780686351));
#79695=CARTESIAN_POINT('Ctrl Pts',(158.781809789108,-15.6744147877999,-6.02623579432656));
#79696=CARTESIAN_POINT('Ctrl Pts',(158.714949565508,-17.9804329801161,-7.16216082908653));
#79697=CARTESIAN_POINT('Ctrl Pts',(158.677501178099,-19.4360368307873,-7.58006858494936));
#79698=CARTESIAN_POINT('Ctrl Pts',(158.932009582291,-12.1040229474429,-0.683975632031794));
#79699=CARTESIAN_POINT('Ctrl Pts',(158.928823828706,-12.2365720458806,-1.6752039782715));
#79700=CARTESIAN_POINT('Ctrl Pts',(158.908274004578,-13.0876839935197,-3.55279470897501));
#79701=CARTESIAN_POINT('Ctrl Pts',(158.847731308557,-15.6548618184882,-6.05617268140067));
#79702=CARTESIAN_POINT('Ctrl Pts',(158.796981635531,-17.9712788484845,-7.18581362478422));
#79703=CARTESIAN_POINT('Ctrl Pts',(158.767483782269,-19.4310494383886,-7.59712554091854));
#79704=CARTESIAN_POINT('Ctrl Pts',(158.982413200833,-12.0208578366741,-0.694683492639026));
#79705=CARTESIAN_POINT('Ctrl Pts',(158.981559128024,-12.1539655941479,-1.70140637942233));
#79706=CARTESIAN_POINT('Ctrl Pts',(158.976089839473,-13.008692313497,-3.60767284657375));
#79707=CARTESIAN_POINT('Ctrl Pts',(158.95907327965,-15.5928048186195,-6.14441085756493));
#79708=CARTESIAN_POINT('Ctrl Pts',(158.943647189037,-17.930100045174,-7.28217025236132));
#79709=CARTESIAN_POINT('Ctrl Pts',(158.934105219764,-19.4029639732492,-7.69317824821817));
#79710=CARTESIAN_POINT('Ctrl Pts',(159.,-11.9254048139712,-0.706973474004925));
#79711=CARTESIAN_POINT('Ctrl Pts',(159.00000343706,-12.0584886535462,-1.73156000225523));
#79712=CARTESIAN_POINT('Ctrl Pts',(158.999868909971,-12.9129618935636,-3.67269437413062));
#79713=CARTESIAN_POINT('Ctrl Pts',(158.999967124078,-15.5043856184253,-6.26523215881831));
#79714=CARTESIAN_POINT('Ctrl Pts',(158.999862355834,-17.8605181164538,-7.43934347766123));
#79715=CARTESIAN_POINT('Ctrl Pts',(159.,-19.3516469022511,-7.8686833920918));
#79716=CARTESIAN_POINT('Ctrl Pts',(159.,-11.877667246487,-0.713119888211845));
#79717=CARTESIAN_POINT('Ctrl Pts',(159.,-12.0107375354121,-1.74664149672305));
#79718=CARTESIAN_POINT('Ctrl Pts',(159.,-12.8650862984908,-3.70517076769771));
#79719=CARTESIAN_POINT('Ctrl Pts',(159.,-15.4601181289741,-6.3256760822434));
#79720=CARTESIAN_POINT('Ctrl Pts',(159.,-17.8256365211145,-7.51804459699146));
#79721=CARTESIAN_POINT('Ctrl Pts',(159.,-19.325905913425,-7.95671795563007));
#79722=CARTESIAN_POINT('Ctrl Pts',(159.,-11.9468127170547,-1.12856807664395));
#79723=CARTESIAN_POINT('Ctrl Pts',(159.,-11.9599365154734,-0.989641976314142));
#79724=CARTESIAN_POINT('Ctrl Pts',(158.993800259316,-11.9710158214162,-0.846323791321935));
#79725=CARTESIAN_POINT('Ctrl Pts',(158.9865805553,-11.9795659353751,-0.699999999999998));
#79726=CARTESIAN_POINT('Ctrl Pts',(158.900103499445,-12.142660775718,-0.699999790428384));
#79727=CARTESIAN_POINT('Ctrl Pts',(158.895418508844,-12.2777930760653,-1.676995454828));
#79728=CARTESIAN_POINT('Ctrl Pts',(158.865988301576,-13.1246369637148,-3.5347632818444));
#79729=CARTESIAN_POINT('Ctrl Pts',(158.781809789108,-15.6744147877999,-6.02623579432656));
#79730=CARTESIAN_POINT('Ctrl Pts',(158.714949565508,-17.9804329801161,-7.16216082908653));
#79731=CARTESIAN_POINT('Ctrl Pts',(158.677501178099,-19.4360368307873,-7.58006858494936));
#79732=CARTESIAN_POINT('Origin',(158.6,-1.33226762955019E-14,0.));
#79733=CARTESIAN_POINT('',(158.752212389381,-16.8466581969835,-12.9841782907193));
#79734=CARTESIAN_POINT('Origin',(158.752212389381,-1.33226762955019E-14,
0.));
#79735=CARTESIAN_POINT('Origin',(158.6,-16.5536728370359,-12.7583664943589));
#79736=CARTESIAN_POINT('Origin',(150.,-1.33226762955019E-14,0.));
#79737=CARTESIAN_POINT('',(141.247787610619,-15.3690953033625,-14.7033903521377));
#79738=CARTESIAN_POINT('Origin',(141.247787610619,-1.33226762955019E-14,
0.));
#79739=CARTESIAN_POINT('Ctrl Pts',(158.752212389381,-16.8466581969835,-12.9841782907193));
#79740=CARTESIAN_POINT('Ctrl Pts',(155.636136052898,-17.4010840024374,-14.3652699144507));
#79741=CARTESIAN_POINT('Ctrl Pts',(149.593137985275,-17.579849295519,-15.751170402598));
#79742=CARTESIAN_POINT('Ctrl Pts',(143.635603997599,-16.2188068453664,-15.236558438444));
#79743=CARTESIAN_POINT('Ctrl Pts',(141.247787610619,-15.3690953033625,-14.7033903521377));
#79744=CARTESIAN_POINT('Origin',(141.4,15.1018066893909,14.4476792155788));
#79745=CARTESIAN_POINT('',(141.349059636029,15.0037376985771,14.8321106819798));
#79746=CARTESIAN_POINT('Origin',(141.4,15.1018066893909,14.4476792155788));
#79747=CARTESIAN_POINT('Origin',(141.4,15.1018066893909,14.4476792155788));
#79748=CARTESIAN_POINT('Origin',(141.4,-1.33226762955019E-14,0.));
#79749=CARTESIAN_POINT('',(141.247787610619,15.2162633908048,-14.8614974586287));
#79750=CARTESIAN_POINT('Origin',(141.247787610619,-1.33226762955019E-14,
0.));
#79751=CARTESIAN_POINT('Ctrl Pts',(141.247876919405,15.2163388788849,-14.861235898812));
#79752=CARTESIAN_POINT('Ctrl Pts',(141.22873525388,15.2139885279162,-14.8523270535713));
#79753=CARTESIAN_POINT('Ctrl Pts',(141.210454198939,15.2112149322114,-14.8418980810186));
#79754=CARTESIAN_POINT('Ctrl Pts',(141.193142866351,15.2080592513282,-14.8301614587166));
#79755=CARTESIAN_POINT('Ctrl Pts',(141.174821340599,15.2047194224462,-14.8177399523627));
#79756=CARTESIAN_POINT('Ctrl Pts',(141.157585042068,15.2009515579434,-14.8038535449713));
#79757=CARTESIAN_POINT('Ctrl Pts',(141.141554659755,15.1968195474827,-14.7886990858493));
#79758=CARTESIAN_POINT('Ctrl Pts',(141.137492013077,15.1957723548302,-14.78485842804));
#79759=CARTESIAN_POINT('Ctrl Pts',(141.133506822801,15.1947018474329,-14.7809360712854));
#79760=CARTESIAN_POINT('Ctrl Pts',(141.129601091572,15.1936092126671,-14.7769347253191));
#79761=CARTESIAN_POINT('Ctrl Pts',(141.119160212917,15.1906883596087,-14.7662382474395));
#79762=CARTESIAN_POINT('Ctrl Pts',(141.109327841191,15.1876223158867,-14.7550201038241));
#79763=CARTESIAN_POINT('Ctrl Pts',(141.100132514679,15.1844291701405,-14.7433390210815));
#79764=CARTESIAN_POINT('Ctrl Pts',(141.086531189282,15.1797060084038,-14.7260608736248));
#79765=CARTESIAN_POINT('Ctrl Pts',(141.074321828766,15.174703784537,-14.7077723961334));
#79766=CARTESIAN_POINT('Ctrl Pts',(141.063480762247,15.1694660242742,-14.6887294572671));
#79767=CARTESIAN_POINT('Ctrl Pts',(141.054049647683,15.16490946916,-14.6721631777643));
#79768=CARTESIAN_POINT('Ctrl Pts',(141.045654236058,15.1601750629473,-14.6550246634294));
#79769=CARTESIAN_POINT('Ctrl Pts',(141.038293602696,15.1553017479839,-14.6374559888653));
#79770=CARTESIAN_POINT('Ctrl Pts',(141.029041027279,15.1491758194103,-14.6153715460741));
#79771=CARTESIAN_POINT('Ctrl Pts',(141.021440949803,15.1428400855676,-14.5926510795041));
#79772=CARTESIAN_POINT('Ctrl Pts',(141.015509436114,15.136348614769,-14.5695453782632));
#79773=CARTESIAN_POINT('Ctrl Pts',(141.009419316295,15.1296835648275,-14.5458218404885));
#79774=CARTESIAN_POINT('Ctrl Pts',(141.00508754459,15.1228546122063,-14.5216910386975));
#79775=CARTESIAN_POINT('Ctrl Pts',(141.002573366043,15.1159363340423,-14.49739370543));
#79776=CARTESIAN_POINT('Ctrl Pts',(141.000971764569,15.1115291989497,-14.4819156301688));
#79777=CARTESIAN_POINT('Ctrl Pts',(141.000108619828,15.107086124888,-14.466369412116));
#79778=CARTESIAN_POINT('Ctrl Pts',(141.000009604167,15.1026288544304,-14.4508143759284));
#79779=CARTESIAN_POINT('Ctrl Pts',(141.000003279229,15.1023441322152,-14.4498207489088));
#79780=CARTESIAN_POINT('Ctrl Pts',(141.000000075317,15.1020593463359,-14.4488271007131));
#79781=CARTESIAN_POINT('Ctrl Pts',(141.,15.1017745018534,-14.4478334468441));
#79782=CARTESIAN_POINT('Ctrl Pts',(141.35099653485,15.2408614483528,-14.8966735002126));
#79783=CARTESIAN_POINT('Ctrl Pts',(141.336701303935,13.5087019185352,-14.3969423499975));
#79784=CARTESIAN_POINT('Ctrl Pts',(141.316047042782,10.3381326773466,-14.5625362559193));
#79785=CARTESIAN_POINT('Ctrl Pts',(141.322570864061,6.83352626350921,-17.0857188547403));
#79786=CARTESIAN_POINT('Ctrl Pts',(141.339649269185,5.6669453478891,-19.2522948677962));
#79787=CARTESIAN_POINT('Ctrl Pts',(141.349059636028,5.34311579305376,-20.4096733396571));
#79788=CARTESIAN_POINT('Ctrl Pts',(141.255191724905,15.2441284491303,-14.885307719899));
#79789=CARTESIAN_POINT('Ctrl Pts',(141.243707662421,13.5104732523515,-14.3817947784593));
#79790=CARTESIAN_POINT('Ctrl Pts',(141.227457326275,10.3319387958253,-14.5433723731474));
#79791=CARTESIAN_POINT('Ctrl Pts',(141.232569272891,6.81927577968571,-17.0740089239655));
#79792=CARTESIAN_POINT('Ctrl Pts',(141.246087054468,5.65358888354726,-19.2467556492176));
#79793=CARTESIAN_POINT('Ctrl Pts',(141.253636400131,5.3313202619847,-20.4063602098348));
#79794=CARTESIAN_POINT('Ctrl Pts',(141.073170497156,15.2707026715556,-14.7928569386893));
#79795=CARTESIAN_POINT('Ctrl Pts',(141.069346965783,13.5170488865775,-14.281399620174));
#79796=CARTESIAN_POINT('Ctrl Pts',(141.064107532769,10.2987202534751,-14.4421866702062));
#79797=CARTESIAN_POINT('Ctrl Pts',(141.06574654537,6.74104576546749,-17.0060750592228));
#79798=CARTESIAN_POINT('Ctrl Pts',(141.070147256206,5.56325958287866,-19.2064921422837));
#79799=CARTESIAN_POINT('Ctrl Pts',(141.07265579263,5.23842562118253,-20.3802679548135));
#79800=CARTESIAN_POINT('Ctrl Pts',(141.,15.3238638924386,-14.6079109289053));
#79801=CARTESIAN_POINT('Ctrl Pts',(141.000060996961,13.5281487514328,-14.0892322818945));
#79802=CARTESIAN_POINT('Ctrl Pts',(141.000108117533,10.2380708838251,-14.2612526730691));
#79803=CARTESIAN_POINT('Ctrl Pts',(141.000092006021,6.59932930492569,-16.8806996527026));
#79804=CARTESIAN_POINT('Ctrl Pts',(141.000039764716,5.38921055259142,-19.1282901366736));
#79805=CARTESIAN_POINT('Ctrl Pts',(141.,5.05377615726458,-20.3284035968646));
#79806=CARTESIAN_POINT('Ctrl Pts',(141.,15.3505314006851,-14.5151356096189));
#79807=CARTESIAN_POINT('Ctrl Pts',(141.,13.5336359395806,-13.9928838398087));
#79808=CARTESIAN_POINT('Ctrl Pts',(141.,10.207722942927,-14.170516626171));
#79809=CARTESIAN_POINT('Ctrl Pts',(141.,6.52826244821434,-16.8178412826011));
#79810=CARTESIAN_POINT('Ctrl Pts',(141.,5.30196057289897,-19.0890348724825));
#79811=CARTESIAN_POINT('Ctrl Pts',(141.,4.96115388172977,-20.3023878438239));
#79812=CARTESIAN_POINT('',(141.35099653485,15.2408614483528,-14.8966735002126));
#79813=CARTESIAN_POINT('',(141.349059636025,5.34311579305105,-20.4096733396652));
#79814=CARTESIAN_POINT('Ctrl Pts',(141.35099653485,15.2408614483528,-14.8966735002126));
#79815=CARTESIAN_POINT('Ctrl Pts',(141.336701303935,13.5087019185352,-14.3969423499975));
#79816=CARTESIAN_POINT('Ctrl Pts',(141.316047042782,10.3381326773466,-14.5625362559193));
#79817=CARTESIAN_POINT('Ctrl Pts',(141.322570864061,6.83352626350921,-17.0857188547403));
#79818=CARTESIAN_POINT('Ctrl Pts',(141.339649269185,5.6669453478891,-19.2522948677962));
#79819=CARTESIAN_POINT('Ctrl Pts',(141.349059636028,5.34311579305376,-20.4096733396571));
#79820=CARTESIAN_POINT('Origin',(141.4,4.96115388172977,-20.3023878438239));
#79821=CARTESIAN_POINT('Ctrl Pts',(141.247876919405,15.2163388788849,-14.861235898812));
#79822=CARTESIAN_POINT('Ctrl Pts',(141.255953752135,15.2173306212471,-14.8649949923886));
#79823=CARTESIAN_POINT('Ctrl Pts',(141.264106131882,15.2185702064193,-14.8685407992313));
#79824=CARTESIAN_POINT('Ctrl Pts',(141.272320148205,15.2200504233193,-14.871870224676));
#79825=CARTESIAN_POINT('Ctrl Pts',(141.292428564115,15.2236740851054,-14.8800208624333));
#79826=CARTESIAN_POINT('Ctrl Pts',(141.312754763776,15.2287111252545,-14.8868154844369));
#79827=CARTESIAN_POINT('Ctrl Pts',(141.333095923651,15.235003560998,-14.8922467653303));
#79828=CARTESIAN_POINT('Ctrl Pts',(141.339062655196,15.2368493394624,-14.8938399387398));
#79829=CARTESIAN_POINT('Ctrl Pts',(141.345030990552,15.2388032249876,-14.8953156859215));
#79830=CARTESIAN_POINT('Ctrl Pts',(141.35099653485,15.2408614483528,-14.8966735002126));
#79831=CARTESIAN_POINT('Origin',(141.4,4.9611538817242,-20.3023878438437));
#79832=CARTESIAN_POINT('',(141.247787610619,5.04896191502906,-20.6617221419649));
#79833=CARTESIAN_POINT('Origin',(141.4,4.9611538817242,-20.3023878438437));
#79834=CARTESIAN_POINT('Origin',(141.4,4.9611538817242,-20.3023878438437));
#79835=CARTESIAN_POINT('Ctrl Pts',(141.349059636029,5.34311579304662,20.4096733396826));
#79836=CARTESIAN_POINT('Ctrl Pts',(141.335218967465,5.81940089586465,18.7074132579652));
#79837=CARTESIAN_POINT('Ctrl Pts',(141.315835564103,7.57351425655429,16.1431928920643));
#79838=CARTESIAN_POINT('Ctrl Pts',(141.323072531631,11.4530715742573,14.4578903667645));
#79839=CARTESIAN_POINT('Ctrl Pts',(141.339832522948,13.8621755940359,14.5396739647276));
#79840=CARTESIAN_POINT('Ctrl Pts',(141.349059636029,15.0037376985838,14.8321106819815));
#79841=CARTESIAN_POINT('Ctrl Pts',(141.253636400131,5.3313202619776,20.4063602098605));
#79842=CARTESIAN_POINT('Ctrl Pts',(141.242532901944,5.80530956055776,18.7008260202169));
#79843=CARTESIAN_POINT('Ctrl Pts',(141.227292561886,7.56035473475804,16.127958124196));
#79844=CARTESIAN_POINT('Ctrl Pts',(141.232962203118,11.4502288056669,14.4398010920777));
#79845=CARTESIAN_POINT('Ctrl Pts',(141.246234067441,13.8640790658792,14.5253853175715));
#79846=CARTESIAN_POINT('Ctrl Pts',(141.253636400131,15.0067662095263,14.8202388875135));
#79847=CARTESIAN_POINT('Ctrl Pts',(141.072655743307,5.23842566295351,20.3802679665741));
#79848=CARTESIAN_POINT('Ctrl Pts',(141.068966214323,5.71618803681672,18.6538908486876));
#79849=CARTESIAN_POINT('Ctrl Pts',(141.064055656561,7.4910368399319,16.0473906113304));
#79850=CARTESIAN_POINT('Ctrl Pts',(141.065873289163,11.4314294069665,14.338120013169));
#79851=CARTESIAN_POINT('Ctrl Pts',(141.07019605713,13.8746384568555,14.4271208562175));
#79852=CARTESIAN_POINT('Ctrl Pts',(141.072655743307,15.0306169635106,14.7267436832411));
#79853=CARTESIAN_POINT('Ctrl Pts',(141.,5.05377615725719,20.3284035968911));
#79854=CARTESIAN_POINT('Ctrl Pts',(141.000058485526,5.54712953739624,18.5632893438755));
#79855=CARTESIAN_POINT('Ctrl Pts',(141.000106861946,7.36766145302611,15.9024052867507));
#79856=CARTESIAN_POINT('Ctrl Pts',(141.00008824024,11.3953681399887,14.1524456691714));
#79857=CARTESIAN_POINT('Ctrl Pts',(141.000038990354,13.8944854484153,14.237366601642));
#79858=CARTESIAN_POINT('Ctrl Pts',(141.,15.078025854662,14.5409003356704));
#79859=CARTESIAN_POINT('Ctrl Pts',(141.,4.96115388172226,20.3023878438507));
#79860=CARTESIAN_POINT('Ctrl Pts',(141.,5.46240877807393,18.5178010571043));
#79861=CARTESIAN_POINT('Ctrl Pts',(141.,7.30575619982316,15.829756813564));
#79862=CARTESIAN_POINT('Ctrl Pts',(141.,11.3772954300569,14.0593422845694));
#79863=CARTESIAN_POINT('Ctrl Pts',(141.,13.9043899707623,14.1422165793403));
#79864=CARTESIAN_POINT('Ctrl Pts',(141.,15.1018066893979,14.4476792155806));
#79865=CARTESIAN_POINT('',(141.349059636029,5.34311579304848,20.409673339676));
#79866=CARTESIAN_POINT('Origin',(141.4,4.96115388172422,20.3023878438437));
#79867=CARTESIAN_POINT('Ctrl Pts',(141.349059636029,5.34311579304662,20.4096733396826));
#79868=CARTESIAN_POINT('Ctrl Pts',(141.335218967465,5.81940089586465,18.7074132579652));
#79869=CARTESIAN_POINT('Ctrl Pts',(141.315835564103,7.57351425655429,16.1431928920643));
#79870=CARTESIAN_POINT('Ctrl Pts',(141.323072531631,11.4530715742573,14.4578903667645));
#79871=CARTESIAN_POINT('Ctrl Pts',(141.339832522948,13.8621755940359,14.5396739647276));
#79872=CARTESIAN_POINT('Ctrl Pts',(141.349059636029,15.0037376985838,14.8321106819815));
#79873=CARTESIAN_POINT('Origin',(141.4,-1.33226762955019E-14,0.));
#79874=CARTESIAN_POINT('',(141.247787610619,-1.43945131843131E-14,-21.2696680343435));
#79875=CARTESIAN_POINT('Origin',(141.247787610619,-1.33226762955019E-14,
0.));
#79876=CARTESIAN_POINT('',(141.247787610619,-5.04896191502908,-20.6617221419649));
#79877=CARTESIAN_POINT('Origin',(141.247787610619,-1.33226762955019E-14,
0.));
#79878=CARTESIAN_POINT('Origin',(141.4,-4.96115388172423,-20.3023878438437));
#79879=CARTESIAN_POINT('Ctrl Pts',(141.349059636022,5.34311579304833,-20.4096733396733));
#79880=CARTESIAN_POINT('Ctrl Pts',(143.733307993271,5.39101415465342,-21.3712117896625));
#79881=CARTESIAN_POINT('Ctrl Pts',(149.658408037072,5.16960571323526,-22.7127474895427));
#79882=CARTESIAN_POINT('Ctrl Pts',(155.615836707894,4.06453754820481,-21.8062184147703));
#79883=CARTESIAN_POINT('Ctrl Pts',(158.677501178099,3.15348645839909,-20.6221359368264));
#79884=CARTESIAN_POINT('Ctrl Pts',(141.323496046572,5.32238907381596,-20.4713275147431));
#79885=CARTESIAN_POINT('Ctrl Pts',(143.710531696096,5.37490885125263,-21.442760228086));
#79886=CARTESIAN_POINT('Ctrl Pts',(149.650520965098,5.16730000482056,-22.8055621649135));
#79887=CARTESIAN_POINT('Ctrl Pts',(155.638467167389,4.07505154866372,-21.9056675808993));
#79888=CARTESIAN_POINT('Ctrl Pts',(158.718387254585,3.16878056711168,-20.7189599683332));
#79889=CARTESIAN_POINT('Ctrl Pts',(141.277191290685,5.24513644961913,-20.5844661011509));
#79890=CARTESIAN_POINT('Ctrl Pts',(143.667118372743,5.29894213621821,-21.5758871460273));
#79891=CARTESIAN_POINT('Ctrl Pts',(149.627591019706,5.10019046858563,-22.9858529525798));
#79892=CARTESIAN_POINT('Ctrl Pts',(155.668404314076,4.01854645839451,-22.1145901623949));
#79893=CARTESIAN_POINT('Ctrl Pts',(158.782431558123,3.11397975410549,-20.9324408777992));
#79894=CARTESIAN_POINT('Ctrl Pts',(141.252831675798,5.11713793346298,-20.647199083878));
#79895=CARTESIAN_POINT('Ctrl Pts',(143.641727065429,5.16024074772474,-21.6486584244251));
#79896=CARTESIAN_POINT('Ctrl Pts',(149.602896580072,4.93867763731753,-23.0827372938334));
#79897=CARTESIAN_POINT('Ctrl Pts',(155.652810905033,3.83759211483587,-22.2322540085573));
#79898=CARTESIAN_POINT('Ctrl Pts',(158.773699287417,2.92284752607858,-21.0592127969533));
#79899=CARTESIAN_POINT('Ctrl Pts',(141.247787610613,5.04896191502895,-20.6617221419621));
#79900=CARTESIAN_POINT('Ctrl Pts',(143.635551134689,5.08584243475458,-21.6641557734155));
#79901=CARTESIAN_POINT('Ctrl Pts',(149.593041994931,4.85101624224383,-23.1002153730525));
#79902=CARTESIAN_POINT('Ctrl Pts',(155.636155285455,3.7401410057494,-22.2524085311578));
#79903=CARTESIAN_POINT('Ctrl Pts',(158.752212389381,2.82129914853753,-21.0817231128206));
#79904=CARTESIAN_POINT('',(158.677501178099,3.15348645839909,-20.6221359368264));
#79905=CARTESIAN_POINT('Ctrl Pts',(141.349059636022,5.34311579304833,-20.4096733396733));
#79906=CARTESIAN_POINT('Ctrl Pts',(143.733307993271,5.39101415465342,-21.3712117896625));
#79907=CARTESIAN_POINT('Ctrl Pts',(149.658408037072,5.16960571323526,-22.7127474895427));
#79908=CARTESIAN_POINT('Ctrl Pts',(155.615836707894,4.06453754820481,-21.8062184147703));
#79909=CARTESIAN_POINT('Ctrl Pts',(158.677501178099,3.15348645839909,-20.6221359368264));
#79910=CARTESIAN_POINT('',(158.752212389117,2.82129914861524,-21.0817231129196));
#79911=CARTESIAN_POINT('Origin',(158.6,2.77223307638906,-20.715084449989));
#79912=CARTESIAN_POINT('Ctrl Pts',(158.752212389381,2.82129914853753,-21.0817231128206));
#79913=CARTESIAN_POINT('Ctrl Pts',(155.636155285455,3.7401410057494,-22.2524085311578));
#79914=CARTESIAN_POINT('Ctrl Pts',(149.593041994931,4.85101624224383,-23.1002153730525));
#79915=CARTESIAN_POINT('Ctrl Pts',(143.635551134689,5.08584243475458,-21.6641557734155));
#79916=CARTESIAN_POINT('Ctrl Pts',(141.247787610613,5.04896191502895,-20.6617221419621));
#79917=CARTESIAN_POINT('Origin',(145.,2.27826388829055E-15,-3.94606880756866E-15));
#79918=CARTESIAN_POINT('',(158.666552508001,16.5975280245508,-13.3571303467592));
#79919=CARTESIAN_POINT('Ctrl Pts',(158.666552508001,16.5975280245508,-13.3571303467592));
#79920=CARTESIAN_POINT('Ctrl Pts',(157.50927066846,16.8048308622113,-13.8504196237403));
#79921=CARTESIAN_POINT('Ctrl Pts',(156.319421579519,16.9470311407289,-14.2561892671813));
#79922=CARTESIAN_POINT('Ctrl Pts',(154.047891554349,17.106405695156,-14.879398590719));
#79923=CARTESIAN_POINT('Ctrl Pts',(152.772096807936,17.134559363704,-15.1462275817564));
#79924=CARTESIAN_POINT('Ctrl Pts',(150.200551186099,17.0444810496483,-15.4961705020678));
#79925=CARTESIAN_POINT('Ctrl Pts',(148.904844084702,16.9260018151287,-15.5795423661919));
#79926=CARTESIAN_POINT('Ctrl Pts',(146.670814422246,16.6120168378012,-15.5916116419199));
#79927=CARTESIAN_POINT('Ctrl Pts',(145.518850226888,16.3987593974049,-15.5359787024709));
#79928=CARTESIAN_POINT('Ctrl Pts',(143.328786142491,15.8712047472997,-15.2906232802717));
#79929=CARTESIAN_POINT('Ctrl Pts',(142.287870643948,15.5641003826617,-15.1099149063184));
#79930=CARTESIAN_POINT('Ctrl Pts',(141.35099653485,15.2408614483528,-14.8966735002126));
#79931=CARTESIAN_POINT('Ctrl Pts',(158.900103530181,6.67754771095066,-10.1658521326993));
#79932=CARTESIAN_POINT('Ctrl Pts',(158.895223267973,7.62986165675312,-9.77859311949994));
#79933=CARTESIAN_POINT('Ctrl Pts',(158.871922952968,9.21993802553689,-9.63677986027857));
#79934=CARTESIAN_POINT('Ctrl Pts',(158.790452736159,12.8229465544963,-10.3829880519117));
#79935=CARTESIAN_POINT('Ctrl Pts',(158.717904052866,15.1374358047924,-11.8431673784125));
#79936=CARTESIAN_POINT('Ctrl Pts',(158.666552508001,16.5975280245508,-13.3571303467592));
#79937=CARTESIAN_POINT('Ctrl Pts',(158.671029640456,6.8062177826491,-10.388715006927));
#79938=CARTESIAN_POINT('Ctrl Pts',(158.642904819311,6.59953105450665,-10.508045645058));
#79939=CARTESIAN_POINT('Ctrl Pts',(158.629834412239,6.39554171986892,-10.6258189423229));
#79940=CARTESIAN_POINT('Ctrl Pts',(158.629834412239,6.00445828013107,-10.8516110715312));
#79941=CARTESIAN_POINT('Ctrl Pts',(158.642904819311,5.80046894549333,-10.9693843687961));
#79942=CARTESIAN_POINT('Ctrl Pts',(158.671029640456,5.59378221735088,-11.088715006927));
#79943=CARTESIAN_POINT('Ctrl Pts',(158.677501178099,3.1534864583991,-20.6221359368264));
#79944=CARTESIAN_POINT('Ctrl Pts',(158.714950329284,2.78759580372903,-19.1525621743689));
#79945=CARTESIAN_POINT('Ctrl Pts',(158.78180847253,2.61832563918518,-16.587611867211));
#79946=CARTESIAN_POINT('Ctrl Pts',(158.865988864041,3.50112315200686,-13.1336286227407));
#79947=CARTESIAN_POINT('Ctrl Pts',(158.895418550926,4.68658266172985,-11.4713730865155));
#79948=CARTESIAN_POINT('Ctrl Pts',(158.900103499456,5.46511278637019,-10.8658525960876));
#79949=CARTESIAN_POINT('Ctrl Pts',(141.349059636028,-5.34311579304847,20.409673339676));
#79950=CARTESIAN_POINT('Ctrl Pts',(143.73334632516,-5.3910149247217,21.3712272484474));
#79951=CARTESIAN_POINT('Ctrl Pts',(149.658864136875,-5.16954303562603,22.712735436463));
#79952=CARTESIAN_POINT('Ctrl Pts',(155.615771953615,-4.0645568169564,21.8062434581409));
#79953=CARTESIAN_POINT('Ctrl Pts',(158.677501178082,-3.15348645840435,20.6221359368332));
#79954=CARTESIAN_POINT('Ctrl Pts',(141.323496046579,-5.32238907381611,20.4713275147458));
#79955=CARTESIAN_POINT('Ctrl Pts',(143.710570072796,-5.37490969562005,21.4427758459423));
#79956=CARTESIAN_POINT('Ctrl Pts',(149.650978989839,-5.16723835490521,22.8055509934857));
#79957=CARTESIAN_POINT('Ctrl Pts',(155.638402027003,-4.07507071631589,21.9056926797915));
#79958=CARTESIAN_POINT('Ctrl Pts',(158.718387254567,-3.1687805671169,20.7189599683401));
#79959=CARTESIAN_POINT('Ctrl Pts',(141.277191290691,-5.24513644961929,20.5844661011536));
#79960=CARTESIAN_POINT('Ctrl Pts',(143.667156795929,-5.29894300125937,21.5759030852388));
#79961=CARTESIAN_POINT('Ctrl Pts',(149.62805219905,-5.10012952348203,22.9858444313653));
#79962=CARTESIAN_POINT('Ctrl Pts',(155.668338452323,-4.01856559000118,22.1146151648783));
#79963=CARTESIAN_POINT('Ctrl Pts',(158.782431558105,-3.11397975411071,20.932440877806));
#79964=CARTESIAN_POINT('Ctrl Pts',(141.252831675805,-5.11713793346311,20.6471990838808));
#79965=CARTESIAN_POINT('Ctrl Pts',(143.641765472029,-5.16024144069435,21.6486745250236));
#79966=CARTESIAN_POINT('Ctrl Pts',(149.603358255898,-4.93861512596577,23.0827304755921));
#79967=CARTESIAN_POINT('Ctrl Pts',(155.652744898167,-3.83761146170504,22.2322788184048));
#79968=CARTESIAN_POINT('Ctrl Pts',(158.773699287399,-2.92284752608386,21.05921279696));
#79969=CARTESIAN_POINT('Ctrl Pts',(141.247787610619,-5.04896191502906,20.6617221419649));
#79970=CARTESIAN_POINT('Ctrl Pts',(143.635589523091,-5.08584302768751,21.6641718896778));
#79971=CARTESIAN_POINT('Ctrl Pts',(149.593503211666,-4.8509528836708,23.1002087288997));
#79972=CARTESIAN_POINT('Ctrl Pts',(155.636089380771,-3.74016043927591,22.2524332911802));
#79973=CARTESIAN_POINT('Ctrl Pts',(158.752212389363,-2.82129914854284,21.0817231128274));
#79974=CARTESIAN_POINT('',(158.67750117809,-3.15348645840273,20.6221359368338));
#79975=CARTESIAN_POINT('',(158.752212389372,-2.82129914854284,21.0817231128274));
#79976=CARTESIAN_POINT('Origin',(158.599999999982,-2.77223307639427,20.7150844499956));
#79977=CARTESIAN_POINT('',(141.247787610619,-5.04896191502906,20.6617221419649));
#79978=CARTESIAN_POINT('Ctrl Pts',(158.752212389363,-2.82129914854284,21.0817231128274));
#79979=CARTESIAN_POINT('Ctrl Pts',(155.636089380771,-3.74016043927591,22.2524332911802));
#79980=CARTESIAN_POINT('Ctrl Pts',(149.593503211666,-4.8509528836708,23.1002087288997));
#79981=CARTESIAN_POINT('Ctrl Pts',(143.635589523091,-5.08584302768751,21.6641718896778));
#79982=CARTESIAN_POINT('Ctrl Pts',(141.247787610619,-5.04896191502906,20.6617221419649));
#79983=CARTESIAN_POINT('',(141.349059636028,-5.34311579304848,20.409673339676));
#79984=CARTESIAN_POINT('Origin',(141.4,-4.96115388172421,20.3023878438437));
#79985=CARTESIAN_POINT('Ctrl Pts',(141.349059636028,-5.34311579304847,20.409673339676));
#79986=CARTESIAN_POINT('Ctrl Pts',(143.73334632516,-5.3910149247217,21.3712272484474));
#79987=CARTESIAN_POINT('Ctrl Pts',(149.658864136875,-5.16954303562603,22.712735436463));
#79988=CARTESIAN_POINT('Ctrl Pts',(155.615771953615,-4.0645568169564,21.8062434581409));
#79989=CARTESIAN_POINT('Ctrl Pts',(158.677501178082,-3.15348645840435,20.6221359368332));
#79990=CARTESIAN_POINT('Origin',(158.6,-2.77223307638907,20.715084449989));
#79991=CARTESIAN_POINT('Origin',(158.6,-2.77223307638907,20.715084449989));
#79992=CARTESIAN_POINT('Origin',(158.6,-2.77223307638907,20.715084449989));
#79993=CARTESIAN_POINT('Origin',(141.4,-1.33226762955019E-14,0.));
#79994=CARTESIAN_POINT('Origin',(141.4,-4.96115388171863,20.3023878438451));
#79995=CARTESIAN_POINT('',(141.247787610619,-1.43945131843131E-14,21.2696680343435));
#79996=CARTESIAN_POINT('Origin',(141.247787610619,-1.33226762955019E-14,
0.));
#79997=CARTESIAN_POINT('',(141.247787610619,5.04896191502908,20.6617221419649));
#79998=CARTESIAN_POINT('Origin',(141.247787610619,-1.33226762955019E-14,
0.));
#79999=CARTESIAN_POINT('Origin',(141.4,4.96115388172422,20.3023878438437));
#80000=CARTESIAN_POINT('Origin',(141.4,4.96115388172422,20.3023878438437));
#80001=CARTESIAN_POINT('Origin',(141.4,4.96115388172422,20.3023878438437));
#80002=CARTESIAN_POINT('Origin',(141.4,-4.96115388172422,20.3023878438437));
#80003=CARTESIAN_POINT('Origin',(141.4,-4.96115388172422,20.3023878438437));
#80004=CARTESIAN_POINT('Origin',(158.6,-1.33226762955019E-14,0.));
#80005=CARTESIAN_POINT('',(158.752212389381,2.82129914853756,21.0817231128206));
#80006=CARTESIAN_POINT('Origin',(158.6,2.77223307638908,20.715084449989));
#80007=CARTESIAN_POINT('Origin',(158.752212389381,-1.33226762955019E-14,
0.));
#80008=CARTESIAN_POINT('Ctrl Pts',(158.677501178099,-3.15348645840112,20.6221359368345));
#80009=CARTESIAN_POINT('Ctrl Pts',(158.727434715347,-2.66561920225437,18.6626518394888));
#80010=CARTESIAN_POINT('Ctrl Pts',(158.796878817868,-2.62551409303562,16.0423039572083));
#80011=CARTESIAN_POINT('Ctrl Pts',(158.873834541859,-3.79508706413997,12.7048043001723));
#80012=CARTESIAN_POINT('Ctrl Pts',(158.895624701124,-4.69489971286054,11.4597227292409));
#80013=CARTESIAN_POINT('Ctrl Pts',(158.900200939034,-5.48157966614798,10.8530999549913));
#80014=CARTESIAN_POINT('Ctrl Pts',(158.767483782269,-3.13622100502129,20.6263452063032));
#80015=CARTESIAN_POINT('Ctrl Pts',(158.806816107544,-2.63795921299991,18.6664469798841));
#80016=CARTESIAN_POINT('Ctrl Pts',(158.858744902204,-2.58820404280957,16.038441954263));
#80017=CARTESIAN_POINT('Ctrl Pts',(158.913599302885,-3.76138733398961,12.6865202525314));
#80018=CARTESIAN_POINT('Ctrl Pts',(158.928823832904,-4.667517865037,11.4347834317933));
#80019=CARTESIAN_POINT('Ctrl Pts',(158.932009582291,-5.45967120081001,10.8243791764931));
#80020=CARTESIAN_POINT('Ctrl Pts',(158.934105907542,-3.03899473697404,20.6500486997849));
#80021=CARTESIAN_POINT('Ctrl Pts',(158.946829133056,-2.53165268785646,18.6752334990121));
#80022=CARTESIAN_POINT('Ctrl Pts',(158.962229996933,-2.48139926659165,16.0241625590793));
#80023=CARTESIAN_POINT('Ctrl Pts',(158.977498208529,-3.68016331100197,12.6412561719165));
#80024=CARTESIAN_POINT('Ctrl Pts',(158.981559195614,-4.60352272666583,11.3763453557565));
#80025=CARTESIAN_POINT('Ctrl Pts',(158.982413267298,-5.40881538133814,10.7577100281132));
#80026=CARTESIAN_POINT('Ctrl Pts',(159.,-2.8613437392394,20.6933595184701));
#80027=CARTESIAN_POINT('Ctrl Pts',(158.999816465792,-2.36299341845418,18.6852310271012));
#80028=CARTESIAN_POINT('Ctrl Pts',(159.00000550089,-2.33816142167315,16.002483772038));
#80029=CARTESIAN_POINT('Ctrl Pts',(158.999898545632,-3.58351118144698,12.5866613751783));
#80030=CARTESIAN_POINT('Ctrl Pts',(159.000003437055,-4.52967045815757,11.3087366794436));
#80031=CARTESIAN_POINT('Ctrl Pts',(159.,-5.3504454186931,10.6811902563167));
#80032=CARTESIAN_POINT('Ctrl Pts',(159.,-2.7722330763911,20.7150844499973));
#80033=CARTESIAN_POINT('Ctrl Pts',(159.,-2.27856657179338,18.6901782082677));
#80034=CARTESIAN_POINT('Ctrl Pts',(159.,-2.26648621108045,15.9916186244315));
#80035=CARTESIAN_POINT('Ctrl Pts',(159.,-3.53520136827782,12.5593409061046));
#80036=CARTESIAN_POINT('Ctrl Pts',(159.,-4.49273395195947,11.274923739443));
#80037=CARTESIAN_POINT('Ctrl Pts',(159.,-5.32125368410558,10.6429215172639));
#80038=CARTESIAN_POINT('Ctrl Pts',(158.677501178099,-3.15348645840112,20.6221359368345));
#80039=CARTESIAN_POINT('Ctrl Pts',(158.727434715347,-2.66561920225437,18.6626518394888));
#80040=CARTESIAN_POINT('Ctrl Pts',(158.796878817868,-2.62551409303562,16.0423039572083));
#80041=CARTESIAN_POINT('Ctrl Pts',(158.873680868674,-3.79275153931752,12.7114689662397));
#80042=CARTESIAN_POINT('Ctrl Pts',(158.895421398181,-4.68652311545549,11.47132952343));
#80043=CARTESIAN_POINT('Ctrl Pts',(158.900103530303,-5.46511233344139,10.8658520071604));
#80044=CARTESIAN_POINT('Ctrl Pts',(158.9865805553,-5.38356518503845,10.7246084263455));
#80045=CARTESIAN_POINT('Ctrl Pts',(158.993842168384,-5.25180960442613,10.7907474151572));
#80046=CARTESIAN_POINT('Ctrl Pts',(159.,-5.12249077216374,10.852623256312));
#80047=CARTESIAN_POINT('Ctrl Pts',(159.,-4.99603773425354,10.9105273455464));
#80048=CARTESIAN_POINT('Origin',(145.,-2.27826388829055E-15,3.94606880756866E-15));
#80049=CARTESIAN_POINT('',(141.349059636029,-15.0037376985771,14.8321106819798));
#80050=CARTESIAN_POINT('Ctrl Pts',(141.349059636029,-15.0037376985771,14.8321106819798));
#80051=CARTESIAN_POINT('Ctrl Pts',(141.33521896633,-13.2913945321224,14.3934556036328));
#80052=CARTESIAN_POINT('Ctrl Pts',(141.315835569127,-10.1936589673169,14.6304522270412));
#80053=CARTESIAN_POINT('Ctrl Pts',(141.323072510929,-6.79436563204128,17.1475934885668));
#80054=CARTESIAN_POINT('Ctrl Pts',(141.339832523646,-5.66063919517391,19.2748332843158));
#80055=CARTESIAN_POINT('Ctrl Pts',(141.349059636029,-5.34311579304661,20.4096733396827));
#80056=CARTESIAN_POINT('',(158.677501178099,-16.2825503723881,13.0420673518771));
#80057=CARTESIAN_POINT('Ctrl Pts',(158.677501178099,-16.2825503723881,13.0420673518771));
#80058=CARTESIAN_POINT('Ctrl Pts',(156.381204089245,-16.70999941537,14.0778653056355));
#80059=CARTESIAN_POINT('Ctrl Pts',(150.57430608297,-17.1406167755042,15.7487354943353));
#80060=CARTESIAN_POINT('Ctrl Pts',(144.528108790922,-16.0821118403393,15.5284558259971));
#80061=CARTESIAN_POINT('Ctrl Pts',(141.349059636029,-15.0037376985771,14.8321106819798));
#80062=CARTESIAN_POINT('Ctrl Pts',(158.900103499495,-6.67754798826902,10.1658528042907));
#80063=CARTESIAN_POINT('Ctrl Pts',(158.895418523778,-7.59121514189452,9.79438361628517));
#80064=CARTESIAN_POINT('Ctrl Pts',(158.865989166098,-9.62348190950228,9.59886873927354));
#80065=CARTESIAN_POINT('Ctrl Pts',(158.781809873649,-13.0560745106574,10.5613269702318));
#80066=CARTESIAN_POINT('Ctrl Pts',(158.71495181987,-15.192764113758,11.9903680096648));
#80067=CARTESIAN_POINT('Ctrl Pts',(158.677501178099,-16.2825503723881,13.0420673518771));
#80068=CARTESIAN_POINT('Ctrl Pts',(158.671029640456,-6.8062177826491,10.388715006927));
#80069=CARTESIAN_POINT('Ctrl Pts',(158.642904819311,-6.59953105450666,10.508045645058));
#80070=CARTESIAN_POINT('Ctrl Pts',(158.629834412239,-6.39554171986892,10.6258189423229));
#80071=CARTESIAN_POINT('Ctrl Pts',(158.629834412239,-6.00445828013107,10.8516110715312));
#80072=CARTESIAN_POINT('Ctrl Pts',(158.642904819311,-5.80046894549334,10.9693843687961));
#80073=CARTESIAN_POINT('Ctrl Pts',(158.671029640456,-5.59378221735089,11.088715006927));
#80074=CARTESIAN_POINT('Ctrl Pts',(141.349059636029,-15.0037376985771,14.8321106819798));
#80075=CARTESIAN_POINT('Ctrl Pts',(141.33521896633,-13.2913945321224,14.3934556036328));
#80076=CARTESIAN_POINT('Ctrl Pts',(141.315835569127,-10.1936589673169,14.6304522270412));
#80077=CARTESIAN_POINT('Ctrl Pts',(141.323072510929,-6.79436563204128,17.1475934885668));
#80078=CARTESIAN_POINT('Ctrl Pts',(141.339832523646,-5.66063919517391,19.2748332843158));
#80079=CARTESIAN_POINT('Ctrl Pts',(141.349059636029,-5.34311579304661,20.4096733396827));
#80080=CARTESIAN_POINT('Ctrl Pts',(141.253636400131,-15.0067662095196,14.8202388875118));
#80081=CARTESIAN_POINT('Ctrl Pts',(141.242532901033,-13.2927354844066,14.3779585301123));
#80082=CARTESIAN_POINT('Ctrl Pts',(141.227292565972,-10.1870450315371,14.6114383647593));
#80083=CARTESIAN_POINT('Ctrl Pts',(141.232962186589,-6.78012124239336,17.1360869354699));
#80084=CARTESIAN_POINT('Ctrl Pts',(141.246234068,-5.64731312794512,19.2693374158744));
#80085=CARTESIAN_POINT('Ctrl Pts',(141.253636400131,-5.33132026197759,20.4063602098605));
#80086=CARTESIAN_POINT('Ctrl Pts',(141.072655743307,-15.0306169635039,14.7267436832394));
#80087=CARTESIAN_POINT('Ctrl Pts',(141.068966214021,-13.2966491937667,14.2773094401772));
#80088=CARTESIAN_POINT('Ctrl Pts',(141.064055657944,-10.1519304760416,14.5111235521553));
#80089=CARTESIAN_POINT('Ctrl Pts',(141.065873283708,-6.7014625547525,17.0689656062841));
#80090=CARTESIAN_POINT('Ctrl Pts',(141.070196057316,-5.55693391244503,19.229349887082));
#80091=CARTESIAN_POINT('Ctrl Pts',(141.072655743307,-5.2384256629535,20.3802679665741));
#80092=CARTESIAN_POINT('Ctrl Pts',(141.,-15.0780258546551,14.5409003356686));
#80093=CARTESIAN_POINT('Ctrl Pts',(141.000058485531,-13.3027152352978,14.0855997320663));
#80094=CARTESIAN_POINT('Ctrl Pts',(141.000106861922,-10.088057220255,14.3317846690823));
#80095=CARTESIAN_POINT('Ctrl Pts',(141.000088240326,-6.55869452112261,16.94489840218));
#80096=CARTESIAN_POINT('Ctrl Pts',(141.000038990351,-5.38267841094074,19.151660760626));
#80097=CARTESIAN_POINT('Ctrl Pts',(141.,-5.05377615725718,20.3284035968911));
#80098=CARTESIAN_POINT('Ctrl Pts',(141.,-15.1018066893909,14.4476792155788));
#80099=CARTESIAN_POINT('Ctrl Pts',(141.,-13.3056816013333,13.9894852586423));
#80100=CARTESIAN_POINT('Ctrl Pts',(141.,-10.0560944361583,14.2418489097857));
#80101=CARTESIAN_POINT('Ctrl Pts',(141.,-6.48710099582796,16.8826952544151));
#80102=CARTESIAN_POINT('Ctrl Pts',(141.,-5.29532381288502,19.1126633184215));
#80103=CARTESIAN_POINT('Ctrl Pts',(141.,-4.96115388172225,20.3023878438507));
#80104=CARTESIAN_POINT('Origin',(141.4,-15.1018066893909,14.4476792155788));
#80105=CARTESIAN_POINT('Ctrl Pts',(158.677501178099,-16.2825503723881,13.0420673518771));
#80106=CARTESIAN_POINT('Ctrl Pts',(156.381204089245,-16.70999941537,14.0778653056355));
#80107=CARTESIAN_POINT('Ctrl Pts',(150.57430608297,-17.1406167755042,15.7487354943353));
#80108=CARTESIAN_POINT('Ctrl Pts',(144.528108790922,-16.0821118403393,15.5284558259971));
#80109=CARTESIAN_POINT('Ctrl Pts',(141.349059636029,-15.0037376985771,14.8321106819798));
#80110=CARTESIAN_POINT('Ctrl Pts',(158.718387254585,-16.3587553890136,13.1037244543038));
#80111=CARTESIAN_POINT('Ctrl Pts',(156.40839816239,-16.7897021217783,14.1374020171573));
#80112=CARTESIAN_POINT('Ctrl Pts',(150.570405308055,-17.2230583865255,15.7963671706555));
#80113=CARTESIAN_POINT('Ctrl Pts',(144.506261651197,-16.1542133839155,15.5532657677844));
#80114=CARTESIAN_POINT('Ctrl Pts',(141.323496046579,-15.0674951400532,14.8449879041224));
#80115=CARTESIAN_POINT('Ctrl Pts',(158.782430907772,-16.5710356244403,13.1630045703251));
#80116=CARTESIAN_POINT('Ctrl Pts',(156.446860905015,-16.9996606910382,14.1938657398615));
#80117=CARTESIAN_POINT('Ctrl Pts',(150.55381965956,-17.4171960553922,15.8338176194597));
#80118=CARTESIAN_POINT('Ctrl Pts',(144.463812293556,-16.3130441322027,15.5577426677024));
#80119=CARTESIAN_POINT('Ctrl Pts',(141.277191383292,-15.2041022649956,14.8346541704741));
#80120=CARTESIAN_POINT('Ctrl Pts',(158.773699287417,-16.7763895028246,13.0608666074492));
#80121=CARTESIAN_POINT('Ctrl Pts',(156.43298332169,-17.1952817892374,14.0949230473093));
#80122=CARTESIAN_POINT('Ctrl Pts',(150.529917358464,-17.5863244008899,15.7415426364467));
#80123=CARTESIAN_POINT('Ctrl Pts',(144.438076973949,-16.4500986002098,15.47259297736));
#80124=CARTESIAN_POINT('Ctrl Pts',(141.252831675805,-15.322429956904,14.7551709869885));
#80125=CARTESIAN_POINT('Ctrl Pts',(158.752212389381,-16.8466581969835,12.9841782907193));
#80126=CARTESIAN_POINT('Ctrl Pts',(156.415119959402,-17.2624838100278,14.0200125997633));
#80127=CARTESIAN_POINT('Ctrl Pts',(150.519349704889,-17.6463691673189,15.6730897992142));
#80128=CARTESIAN_POINT('Ctrl Pts',(144.431523730316,-16.5020372424295,15.4142768773742));
#80129=CARTESIAN_POINT('Ctrl Pts',(141.247787610619,-15.3690953033625,14.7033903521377));
#80130=CARTESIAN_POINT('',(141.247787610619,-15.3690953033625,14.7033903521377));
#80131=CARTESIAN_POINT('Origin',(141.4,-15.1018066893909,14.4476792155788));
#80132=CARTESIAN_POINT('',(158.752212389381,-16.8466581969835,12.9841782907193));
#80133=CARTESIAN_POINT('Ctrl Pts',(141.247787610619,-15.3690953033625,14.7033903521377));
#80134=CARTESIAN_POINT('Ctrl Pts',(144.431523730316,-16.5020372424295,15.4142768773742));
#80135=CARTESIAN_POINT('Ctrl Pts',(150.519349704889,-17.6463691673189,15.6730897992142));
#80136=CARTESIAN_POINT('Ctrl Pts',(156.415119959402,-17.2624838100278,14.0200125997633));
#80137=CARTESIAN_POINT('Ctrl Pts',(158.752212389381,-16.8466581969835,12.9841782907193));
#80138=CARTESIAN_POINT('Origin',(158.6,-16.5536728370359,12.7583664943589));
#80139=CARTESIAN_POINT('Origin',(158.6,-16.5536728370359,12.7583664943589));
#80140=CARTESIAN_POINT('Origin',(158.6,-16.5536728370359,12.7583664943589));
#80141=CARTESIAN_POINT('Origin',(158.6,-16.5536728370359,12.7583664943589));
#80142=CARTESIAN_POINT('Origin',(141.4,-15.1018066893909,14.4476792155788));
#80143=CARTESIAN_POINT('Origin',(141.4,-15.1018066893909,14.4476792155788));
#80144=CARTESIAN_POINT('Ctrl Pts',(158.900200939034,-6.65827043776022,10.173737221248));
#80145=CARTESIAN_POINT('Ctrl Pts',(158.895624704489,-7.57696047183815,9.79576406212931));
#80146=CARTESIAN_POINT('Ctrl Pts',(158.866157601674,-9.61661358482785,9.59694294254089));
#80147=CARTESIAN_POINT('Ctrl Pts',(158.781809873649,-13.0560745106574,10.5613269702318));
#80148=CARTESIAN_POINT('Ctrl Pts',(158.71495181987,-15.192764113758,11.9903680096648));
#80149=CARTESIAN_POINT('Ctrl Pts',(158.677501178099,-16.2825503723881,13.0420673518771));
#80150=CARTESIAN_POINT('Ctrl Pts',(158.932009582291,-6.64435174663334,10.1404035444583));
#80151=CARTESIAN_POINT('Ctrl Pts',(158.928823835247,-7.569053326187,9.75958103968309));
#80152=CARTESIAN_POINT('Ctrl Pts',(158.908274661215,-9.62062110267634,9.5578506046531));
#80153=CARTESIAN_POINT('Ctrl Pts',(158.847731347736,-13.0722241734835,10.5294251241165));
#80154=CARTESIAN_POINT('Ctrl Pts',(158.796983411277,-15.2086711883374,11.9706134855125));
#80155=CARTESIAN_POINT('Ctrl Pts',(158.767483782269,-16.2948284333693,13.0292196653766));
#80156=CARTESIAN_POINT('Ctrl Pts',(158.982413165375,-6.61204246539703,10.0630265031676));
#80157=CARTESIAN_POINT('Ctrl Pts',(158.981559094319,-7.55044201207679,9.67494055595002));
#80158=CARTESIAN_POINT('Ctrl Pts',(158.976089907337,-9.62865081747194,9.46200255793715));
#80159=CARTESIAN_POINT('Ctrl Pts',(158.959073130834,-13.1176119648907,10.4315631799996));
#80160=CARTESIAN_POINT('Ctrl Pts',(158.943647396539,-15.2715289040604,11.8867723722053));
#80161=CARTESIAN_POINT('Ctrl Pts',(158.934104852847,-16.3639699937563,12.9568703674407));
#80162=CARTESIAN_POINT('Ctrl Pts',(159.,-6.57495939527851,9.97421678230863));
#80163=CARTESIAN_POINT('Ctrl Pts',(159.000003437053,-7.52881731858658,9.57717831922963));
#80164=CARTESIAN_POINT('Ctrl Pts',(158.999868817248,-9.63709524450697,9.34658683117197));
#80165=CARTESIAN_POINT('Ctrl Pts',(158.999966995003,-13.1780366342351,10.2945794162384));
#80166=CARTESIAN_POINT('Ctrl Pts',(158.999862347547,-15.3728522317907,11.7479258592004));
#80167=CARTESIAN_POINT('Ctrl Pts',(159.,-16.4903031630138,12.82467612637));
#80168=CARTESIAN_POINT('Ctrl Pts',(159.,-6.55641356238179,9.92980162904894));
#80169=CARTESIAN_POINT('Ctrl Pts',(159.,-7.51800270098316,9.52828389982869));
#80170=CARTESIAN_POINT('Ctrl Pts',(159.,-9.64128250186339,9.28888713869177));
#80171=CARTESIAN_POINT('Ctrl Pts',(159.,-13.2082488270869,10.226020745615));
#80172=CARTESIAN_POINT('Ctrl Pts',(159.,-15.423567841049,11.6783667562433));
#80173=CARTESIAN_POINT('Ctrl Pts',(159.,-16.5536728370359,12.7583664943589));
#80174=CARTESIAN_POINT('Ctrl Pts',(159.,-6.95077498280114,9.78195926890241));
#80175=CARTESIAN_POINT('Ctrl Pts',(159.,-6.83500808409849,9.86421985098201));
#80176=CARTESIAN_POINT('Ctrl Pts',(158.993725391353,-6.71717606475048,9.94487738541079));
#80177=CARTESIAN_POINT('Ctrl Pts',(158.9865805553,-6.59600075033666,10.0246084263455));
#80178=CARTESIAN_POINT('Origin',(158.6,-1.33226762955019E-14,0.));
#80179=CARTESIAN_POINT('',(158.752212389381,-19.8232298288527,7.70962628430587));
#80180=CARTESIAN_POINT('Origin',(158.752212389381,-1.33226762955019E-14,
0.));
#80181=CARTESIAN_POINT('Ctrl Pts',(159.,-19.325905913425,7.95671795563007));
#80182=CARTESIAN_POINT('Ctrl Pts',(159.,-19.3270536862574,7.95616651092987));
#80183=CARTESIAN_POINT('Ctrl Pts',(158.999997281692,-19.3282014128002,7.95561496081234));
#80184=CARTESIAN_POINT('Ctrl Pts',(158.999597040786,-19.4126972786059,7.91500032696912));
#80185=CARTESIAN_POINT('Ctrl Pts',(158.984861677683,-19.4971388133457,7.87369754969672));
#80186=CARTESIAN_POINT('Ctrl Pts',(158.930181269471,-19.6379934364656,7.80372244999901));
#80187=CARTESIAN_POINT('Ctrl Pts',(158.896925699168,-19.6933659744141,7.77581497074402));
#80188=CARTESIAN_POINT('Ctrl Pts',(158.827213134256,-19.7716384126688,7.73606875989221));
#80189=CARTESIAN_POINT('Ctrl Pts',(158.792347045386,-19.801086988096,7.72099850711088));
#80190=CARTESIAN_POINT('Ctrl Pts',(158.752212389381,-19.8232298288527,7.70962628430587));
#80191=CARTESIAN_POINT('Origin',(150.,-1.33226762955019E-14,0.));
#80192=CARTESIAN_POINT('',(141.247787610619,-20.4785660328528,5.7469219177978));
#80193=CARTESIAN_POINT('Origin',(141.247787610619,-1.33226762955019E-14,
0.));
#80194=CARTESIAN_POINT('',(141.35099653485,-20.521328407243,5.75063643972612));
#80195=CARTESIAN_POINT('Ctrl Pts',(141.35099653485,-20.521328407243,5.75063643972611));
#80196=CARTESIAN_POINT('Ctrl Pts',(141.330560580639,-20.5137747709527,5.74685599072201));
#80197=CARTESIAN_POINT('Ctrl Pts',(141.310156338475,-20.5056601604638,5.74483752080369));
#80198=CARTESIAN_POINT('Ctrl Pts',(141.289960851433,-20.4970796083446,5.74467654273788));
#80199=CARTESIAN_POINT('Ctrl Pts',(141.275805040356,-20.491065161925,5.74456370688092));
#80200=CARTESIAN_POINT('Ctrl Pts',(141.261752355578,-20.4848213996491,5.74536409896549));
#80201=CARTESIAN_POINT('Ctrl Pts',(141.247876819781,-20.4783773106294,5.74711800167204));
#80202=CARTESIAN_POINT('',(158.666552508001,-19.866378214229,7.69531573590557));
#80203=CARTESIAN_POINT('Ctrl Pts',(141.35099653485,-20.521328407243,5.75063643972611));
#80204=CARTESIAN_POINT('Ctrl Pts',(142.287870643948,-20.8676203492237,5.9239488652769));
#80205=CARTESIAN_POINT('Ctrl Pts',(143.328786142491,-21.1776705740628,6.09955485968982));
#80206=CARTESIAN_POINT('Ctrl Pts',(145.518850226888,-21.6539319276962,6.43375287746594));
#80207=CARTESIAN_POINT('Ctrl Pts',(146.670814422246,-21.8087401867444,6.59062276867075));
#80208=CARTESIAN_POINT('Ctrl Pts',(148.904844084701,-21.9552803760225,6.86857637330707));
#80209=CARTESIAN_POINT('Ctrl Pts',(150.200551186099,-21.94231784099,7.01286833228401));
#80210=CARTESIAN_POINT('Ctrl Pts',(152.772096807936,-21.6842975391536,7.26584990074203));
#80211=CARTESIAN_POINT('Ctrl Pts',(154.047891554348,-21.4391400201751,7.37488260408839));
#80212=CARTESIAN_POINT('Ctrl Pts',(156.319421579519,-20.8197376369026,7.54846485300654));
#80213=CARTESIAN_POINT('Ctrl Pts',(157.50927066846,-20.3972306783393,7.62820062110565));
#80214=CARTESIAN_POINT('Ctrl Pts',(158.666552508001,-19.866378214229,7.69531573590557));
#80215=CARTESIAN_POINT('Ctrl Pts',(158.752121561149,-19.8231768430188,7.7098368527046));
#80216=CARTESIAN_POINT('Ctrl Pts',(158.731582665339,-19.8345398203132,7.70394690811282));
#80217=CARTESIAN_POINT('Ctrl Pts',(158.710372605511,-19.8455141791982,7.69970518087406));
#80218=CARTESIAN_POINT('Ctrl Pts',(158.688685765167,-19.8559681294348,7.69722256756614));
#80219=CARTESIAN_POINT('Ctrl Pts',(158.681360078093,-19.8594994123191,7.69638395539713));
#80220=CARTESIAN_POINT('Ctrl Pts',(158.673979887952,-19.8629712282948,7.69574647752882));
#80221=CARTESIAN_POINT('Ctrl Pts',(158.666552508001,-19.866378214229,7.69531573590557));
#80222=CARTESIAN_POINT('Origin',(141.4,-1.33226762955019E-14,0.));
#80223=CARTESIAN_POINT('Ctrl Pts',(141.,-20.0630774021743,5.85460310441089));
#80224=CARTESIAN_POINT('Ctrl Pts',(141.000000075299,-20.0640803349356,5.85435296787516));
#80225=CARTESIAN_POINT('Ctrl Pts',(141.000003279031,-20.0650832335206,5.85410278338991));
#80226=CARTESIAN_POINT('Ctrl Pts',(141.000009603626,-20.0660860819175,5.8538525543453));
#80227=CARTESIAN_POINT('Ctrl Pts',(141.000164915114,-20.0907127771228,5.84770774279479));
#80228=CARTESIAN_POINT('Ctrl Pts',(141.002197860735,-20.115303347739,5.84154284904989));
#80229=CARTESIAN_POINT('Ctrl Pts',(141.006018562783,-20.1396170949448,5.8354021009403));
#80230=CARTESIAN_POINT('Ctrl Pts',(141.009765993263,-20.1634645649167,5.82937911711517));
#80231=CARTESIAN_POINT('Ctrl Pts',(141.015233878042,-20.1870465859547,5.82337854097395));
#80232=CARTESIAN_POINT('Ctrl Pts',(141.022381274184,-20.2101270862119,5.81746117552719));
#80233=CARTESIAN_POINT('Ctrl Pts',(141.026987855897,-20.2250027427908,5.81364736320695));
#80234=CARTESIAN_POINT('Ctrl Pts',(141.032292956913,-20.2396698582708,5.80986852991932));
#80235=CARTESIAN_POINT('Ctrl Pts',(141.038293871982,-20.2540606729038,5.8061477103125));
#80236=CARTESIAN_POINT('Ctrl Pts',(141.046754898227,-20.2743510884317,5.80090151835933));
#80237=CARTESIAN_POINT('Ctrl Pts',(141.056582702942,-20.2940579908126,5.7957799083375));
#80238=CARTESIAN_POINT('Ctrl Pts',(141.067780349377,-20.3129632930785,5.79084165904802));
#80239=CARTESIAN_POINT('Ctrl Pts',(141.077521560447,-20.329409654443,5.78654570909808));
#80240=CARTESIAN_POINT('Ctrl Pts',(141.088299997981,-20.3452493754742,5.7823886538782));
#80241=CARTESIAN_POINT('Ctrl Pts',(141.100132190866,-20.360320826308,5.77843162140958));
#80242=CARTESIAN_POINT('Ctrl Pts',(141.109327618073,-20.3720336533709,5.77535640074913));
#80243=CARTESIAN_POINT('Ctrl Pts',(141.119160111107,-20.3832819963207,5.77240258164491));
#80244=CARTESIAN_POINT('Ctrl Pts',(141.129601129032,-20.3940059513244,5.76958386172458));
#80245=CARTESIAN_POINT('Ctrl Pts',(141.145068430555,-20.4098923952289,5.76540821609));
#80246=CARTESIAN_POINT('Ctrl Pts',(141.161781511794,-20.4245352294047,5.76154855185975));
#80247=CARTESIAN_POINT('Ctrl Pts',(141.179618019521,-20.4377389671605,5.75803884263087));
#80248=CARTESIAN_POINT('Ctrl Pts',(141.196458208456,-20.4502051652447,5.75472518014572));
#80249=CARTESIAN_POINT('Ctrl Pts',(141.214300716487,-20.4613887103233,5.75172342846531));
#80250=CARTESIAN_POINT('Ctrl Pts',(141.233038698374,-20.4710926786894,5.74909543745987));
#80251=CARTESIAN_POINT('Ctrl Pts',(141.237924600173,-20.4736229744694,5.7484101925889));
#80252=CARTESIAN_POINT('Ctrl Pts',(141.242871325276,-20.4760524869387,5.74775054600602));
#80253=CARTESIAN_POINT('Ctrl Pts',(141.247876819781,-20.4783773106294,5.74711800167204));
#80254=CARTESIAN_POINT('Origin',(141.4,-1.33226762955019E-14,0.));
#80255=CARTESIAN_POINT('Origin',(141.4,-15.1018066893949,-14.4476792155747));
#80256=CARTESIAN_POINT('Origin',(141.4,-15.101806689391,-14.4476792155788));
#80257=CARTESIAN_POINT('',(141.349059636029,-15.0037376985772,-14.8321106819798));
#80258=CARTESIAN_POINT('Origin',(141.4,-15.101806689391,-14.4476792155788));
#80259=CARTESIAN_POINT('Origin',(141.4,-15.101806689391,-14.4476792155788));
#80260=CARTESIAN_POINT('Ctrl Pts',(141.349059636029,-20.3468534916256,-5.57756265769617));
#80261=CARTESIAN_POINT('Ctrl Pts',(141.339649255539,-19.5064478919129,-4.71842755492015));
#80262=CARTESIAN_POINT('Ctrl Pts',(141.322571162744,-18.2134451385918,-2.62488542022268));
#80263=CARTESIAN_POINT('Ctrl Pts',(141.316047048714,-17.7805825851918,1.67182024814345));
#80264=CARTESIAN_POINT('Ctrl Pts',(141.336701199134,-19.2224592489608,4.50039869290468));
#80265=CARTESIAN_POINT('Ctrl Pts',(141.35099653485,-20.521328407243,5.75063643972612));
#80266=CARTESIAN_POINT('Ctrl Pts',(141.253636400131,-20.3380864714991,-5.58612132234199));
#80267=CARTESIAN_POINT('Ctrl Pts',(141.246087043521,-19.4949725518084,-4.72722498340188));
#80268=CARTESIAN_POINT('Ctrl Pts',(141.232569467112,-18.1961787455388,-2.63137152277999));
#80269=CARTESIAN_POINT('Ctrl Pts',(141.227457267469,-17.7608890108664,1.67603859357766));
#80270=CARTESIAN_POINT('Ctrl Pts',(141.243707578229,-19.210226704618,4.50950650312373));
#80271=CARTESIAN_POINT('Ctrl Pts',(141.255191724905,-20.5131188531463,5.75914863555041));
#80272=CARTESIAN_POINT('Ctrl Pts',(141.072655152543,-20.2690429983793,-5.6535239202469));
#80273=CARTESIAN_POINT('Ctrl Pts',(141.070146612482,-19.4149390686586,-4.78532029212865));
#80274=CARTESIAN_POINT('Ctrl Pts',(141.065746086537,-18.0982320829347,-2.66515413199565));
#80275=CARTESIAN_POINT('Ctrl Pts',(141.064107045096,-17.6566508607726,1.69786347454426));
#80276=CARTESIAN_POINT('Ctrl Pts',(141.06934629075,-19.1265700376063,4.56539823894889));
#80277=CARTESIAN_POINT('Ctrl Pts',(141.073169850154,-20.446341636345,5.82838756610875));
#80278=CARTESIAN_POINT('Ctrl Pts',(141.,-20.1318020119142,-5.7875032612156));
#80279=CARTESIAN_POINT('Ctrl Pts',(141.000039764774,-19.260189201668,-4.8969505320422));
#80280=CARTESIAN_POINT('Ctrl Pts',(141.000091672766,-17.9187953505145,-2.72519747653006));
#80281=CARTESIAN_POINT('Ctrl Pts',(141.000107636033,-17.4696319962042,1.73580630515009));
#80282=CARTESIAN_POINT('Ctrl Pts',(141.000060997409,-18.965697576164,4.67109484420677));
#80283=CARTESIAN_POINT('Ctrl Pts',(141.,-20.3127539068717,5.96689995053431));
#80284=CARTESIAN_POINT('Ctrl Pts',(141.,-20.0629605711152,-5.85470862826492));
#80285=CARTESIAN_POINT('Ctrl Pts',(141.,-19.1825681430686,-4.95288358249382));
#80286=CARTESIAN_POINT('Ctrl Pts',(141.,-17.8288251260465,-2.75531450942628));
#80287=CARTESIAN_POINT('Ctrl Pts',(141.,-17.3758782127324,1.7548920617158));
#80288=CARTESIAN_POINT('Ctrl Pts',(141.,-18.885000871452,4.72402098820429));
#80289=CARTESIAN_POINT('Ctrl Pts',(141.,-20.2457418776487,6.03638234977462));
#80290=CARTESIAN_POINT('Ctrl Pts',(141.349059636029,-20.3468534916256,-5.57756265769617));
#80291=CARTESIAN_POINT('Ctrl Pts',(141.339649255539,-19.5064478919129,-4.71842755492015));
#80292=CARTESIAN_POINT('Ctrl Pts',(141.322571162744,-18.2134451385918,-2.62488542022268));
#80293=CARTESIAN_POINT('Ctrl Pts',(141.316047048714,-17.7805825851918,1.67182024814345));
#80294=CARTESIAN_POINT('Ctrl Pts',(141.336701199134,-19.2224592489608,4.50039869290468));
#80295=CARTESIAN_POINT('Ctrl Pts',(141.35099653485,-20.521328407243,5.75063643972612));
#80296=CARTESIAN_POINT('Origin',(145.,-4.5565277765811E-15,5.58013715681605E-31));
#80297=CARTESIAN_POINT('Ctrl Pts',(158.671029640456,-12.4,-0.699999999999999));
#80298=CARTESIAN_POINT('Ctrl Pts',(158.642904819311,-12.4,-0.461338723738069));
#80299=CARTESIAN_POINT('Ctrl Pts',(158.629834412239,-12.4,-0.22579212920825));
#80300=CARTESIAN_POINT('Ctrl Pts',(158.629834412239,-12.4,0.225792129208253));
#80301=CARTESIAN_POINT('Ctrl Pts',(158.642904819311,-12.4,0.461338723738072));
#80302=CARTESIAN_POINT('Ctrl Pts',(158.671029640456,-12.4,0.700000000000002));
#80303=CARTESIAN_POINT('Ctrl Pts',(158.666552508001,-19.866378214229,7.69531573590557));
#80304=CARTESIAN_POINT('Ctrl Pts',(158.70506309762,-18.3356178296977,7.31472446391733));
#80305=CARTESIAN_POINT('Ctrl Pts',(158.774612832515,-15.8996513054051,6.19397172155974));
#80306=CARTESIAN_POINT('Ctrl Pts',(158.863666938984,-13.1911946894156,3.6470723687705));
#80307=CARTESIAN_POINT('Ctrl Pts',(158.895220191772,-12.283511760518,1.71833536753634));
#80308=CARTESIAN_POINT('Ctrl Pts',(158.900103498665,-12.1426607830635,0.699999789453026));
#80309=CARTESIAN_POINT('Origin',(158.6,2.77223307638906,-20.715084449989));
#80310=CARTESIAN_POINT('Origin',(158.6,2.77223307638906,-20.715084449989));
#80311=CARTESIAN_POINT('Origin',(158.6,2.772233076494,-20.7150844499749));
#80312=CARTESIAN_POINT('Ctrl Pts',(158.677501178099,3.1534864583991,-20.6221359368264));
#80313=CARTESIAN_POINT('Ctrl Pts',(158.714950329284,2.78759580372903,-19.1525621743689));
#80314=CARTESIAN_POINT('Ctrl Pts',(158.78180847253,2.61832563918518,-16.587611867211));
#80315=CARTESIAN_POINT('Ctrl Pts',(158.866157302936,3.50288956619025,-13.1267174512618));
#80316=CARTESIAN_POINT('Ctrl Pts',(158.895624735314,4.69490559037239,-11.4597181969879));
#80317=CARTESIAN_POINT('Ctrl Pts',(158.900200939034,5.48157966614797,-10.8530999549913));
#80318=CARTESIAN_POINT('Ctrl Pts',(158.767483782269,3.13622100501922,-20.6263452062951));
#80319=CARTESIAN_POINT('Ctrl Pts',(158.796982237153,2.76253465697509,-19.1564608553406));
#80320=CARTESIAN_POINT('Ctrl Pts',(158.84773035255,2.58262323448792,-16.5856470391604));
#80321=CARTESIAN_POINT('Ctrl Pts',(158.908274443688,3.46703104228078,-13.1106418265079));
#80322=CARTESIAN_POINT('Ctrl Pts',(158.928823856706,4.66752378344207,-11.4347788712878));
#80323=CARTESIAN_POINT('Ctrl Pts',(158.932009582291,5.45967120081,-10.8243791764932));
#80324=CARTESIAN_POINT('Ctrl Pts',(158.934105907542,3.03899473697194,-20.6500486997768));
#80325=CARTESIAN_POINT('Ctrl Pts',(158.943648071429,2.65849837827092,-19.1689769173166));
#80326=CARTESIAN_POINT('Ctrl Pts',(158.959073295874,2.47517804757704,-16.5760237552371));
#80327=CARTESIAN_POINT('Ctrl Pts',(158.976090240053,3.38000941312232,-13.0696719567789));
#80328=CARTESIAN_POINT('Ctrl Pts',(158.981559201995,4.60352874323852,-11.3763407337543));
#80329=CARTESIAN_POINT('Ctrl Pts',(158.982413267298,5.40881538133813,-10.7577100281132));
#80330=CARTESIAN_POINT('Ctrl Pts',(159.,2.86134373923733,-20.6933595184618));
#80331=CARTESIAN_POINT('Ctrl Pts',(158.999862353026,2.4875909963964,-19.1873034363753));
#80332=CARTESIAN_POINT('Ctrl Pts',(158.999967281116,2.32633340922194,-16.5598617104212));
#80333=CARTESIAN_POINT('Ctrl Pts',(158.999869016155,3.27583397038329,-13.0192774694505));
#80334=CARTESIAN_POINT('Ctrl Pts',(159.000003437029,4.52967659040301,-11.308731990864));
#80335=CARTESIAN_POINT('Ctrl Pts',(159.,5.35044541869309,-10.6811902563167));
#80336=CARTESIAN_POINT('Ctrl Pts',(159.,2.77223307638906,-20.715084449989));
#80337=CARTESIAN_POINT('Ctrl Pts',(159.,2.40199310172352,-19.1964453917219));
#80338=CARTESIAN_POINT('Ctrl Pts',(159.,2.25185337892959,-16.5517472098717));
#80339=CARTESIAN_POINT('Ctrl Pts',(159.,3.22377088482673,-12.9940540491684));
#80340=CARTESIAN_POINT('Ctrl Pts',(159.,4.49274014206833,-11.2749190175729));
#80341=CARTESIAN_POINT('Ctrl Pts',(159.,5.32125368410557,-10.6429215172639));
#80342=CARTESIAN_POINT('Ctrl Pts',(158.9865805553,5.38356518503844,-10.7246084263456));
#80343=CARTESIAN_POINT('Ctrl Pts',(158.993847133043,5.25171952506417,-10.7907926334157));
#80344=CARTESIAN_POINT('Ctrl Pts',(159.,5.12244181219467,-10.8526456755632));
#80345=CARTESIAN_POINT('Ctrl Pts',(159.,4.99603773425355,-10.9105273455463));
#80346=CARTESIAN_POINT('Origin',(158.6,-2.77223307638909,-20.715084449989));
#80347=CARTESIAN_POINT('',(158.752212389381,-2.82129914853757,-21.0817231128207));
#80348=CARTESIAN_POINT('Origin',(158.6,-2.77223307638909,-20.715084449989));
#80349=CARTESIAN_POINT('',(158.677501178099,-3.15348645839912,-20.6221359368264));
#80350=CARTESIAN_POINT('Origin',(158.6,-2.77223307638909,-20.715084449989));
#80351=CARTESIAN_POINT('Origin',(158.6,-2.77223307638909,-20.715084449989));
#80352=CARTESIAN_POINT('Origin',(158.6,-1.33226762955019E-14,0.));
#80353=CARTESIAN_POINT('Origin',(158.752212389381,-1.33226762955019E-14,
0.));
#80354=CARTESIAN_POINT('Origin',(141.4,-4.96115388172423,-20.3023878438437));
#80355=CARTESIAN_POINT('',(141.349059636029,-5.34311579304849,-20.409673339676));
#80356=CARTESIAN_POINT('Origin',(141.4,-4.96115388172423,-20.3023878438437));
#80357=CARTESIAN_POINT('Origin',(141.4,-4.96115388172423,-20.3023878438437));
#80358=CARTESIAN_POINT('Ctrl Pts',(141.349059636029,-5.34311579304849,-20.409673339676));
#80359=CARTESIAN_POINT('Ctrl Pts',(141.335218967465,-5.81940089586769,-18.7074132579599));
#80360=CARTESIAN_POINT('Ctrl Pts',(141.315835564103,-7.57351425655799,-16.1431928920618));
#80361=CARTESIAN_POINT('Ctrl Pts',(141.323072531631,-11.4530715742594,-14.4578903667644));
#80362=CARTESIAN_POINT('Ctrl Pts',(141.339832522948,-13.8621755940366,-14.5396739647277));
#80363=CARTESIAN_POINT('Ctrl Pts',(141.349059636029,-15.0037376985838,-14.8321106819815));
#80364=CARTESIAN_POINT('Ctrl Pts',(141.253636400131,-5.33132026197946,-20.4063602098538));
#80365=CARTESIAN_POINT('Ctrl Pts',(141.242532901944,-5.8053095605608,-18.7008260202115));
#80366=CARTESIAN_POINT('Ctrl Pts',(141.227292561886,-7.56035473476176,-16.1279581241935));
#80367=CARTESIAN_POINT('Ctrl Pts',(141.232962203118,-11.450228805669,-14.4398010920776));
#80368=CARTESIAN_POINT('Ctrl Pts',(141.246234067441,-13.8640790658799,-14.5253853175717));
#80369=CARTESIAN_POINT('Ctrl Pts',(141.253636400131,-15.0067662095263,-14.8202388875135));
#80370=CARTESIAN_POINT('Ctrl Pts',(141.072655743307,-5.23842566295538,-20.3802679665673));
#80371=CARTESIAN_POINT('Ctrl Pts',(141.068966214323,-5.71618803681979,-18.6538908486823));
#80372=CARTESIAN_POINT('Ctrl Pts',(141.064055656561,-7.49103683993567,-16.0473906113278));
#80373=CARTESIAN_POINT('Ctrl Pts',(141.065873289163,-11.4314294069686,-14.3381200131689));
#80374=CARTESIAN_POINT('Ctrl Pts',(141.07019605713,-13.8746384568562,-14.4271208562177));
#80375=CARTESIAN_POINT('Ctrl Pts',(141.072655743307,-15.0306169635106,-14.7267436832411));
#80376=CARTESIAN_POINT('Ctrl Pts',(141.,-5.05377615725913,-20.3284035968842));
#80377=CARTESIAN_POINT('Ctrl Pts',(141.000058485526,-5.5471295373994,-18.56328934387));
#80378=CARTESIAN_POINT('Ctrl Pts',(141.000106861946,-7.36766145302996,-15.9024052867481));
#80379=CARTESIAN_POINT('Ctrl Pts',(141.00008824024,-11.3953681399908,-14.1524456691713));
#80380=CARTESIAN_POINT('Ctrl Pts',(141.000038990354,-13.894485448416,-14.2373666016421));
#80381=CARTESIAN_POINT('Ctrl Pts',(141.,-15.0780258546621,-14.5409003356704));
#80382=CARTESIAN_POINT('Ctrl Pts',(141.,-4.96115388172423,-20.3023878438437));
#80383=CARTESIAN_POINT('Ctrl Pts',(141.,-5.46240877807713,-18.5178010570987));
#80384=CARTESIAN_POINT('Ctrl Pts',(141.,-7.30575619982706,-15.8297568135614));
#80385=CARTESIAN_POINT('Ctrl Pts',(141.,-11.3772954300591,-14.0593422845693));
#80386=CARTESIAN_POINT('Ctrl Pts',(141.,-13.9043899707631,-14.1422165793404));
#80387=CARTESIAN_POINT('Ctrl Pts',(141.,-15.101806689398,-14.4476792155806));
#80388=CARTESIAN_POINT('Ctrl Pts',(141.349059636029,-5.34311579304849,-20.409673339676));
#80389=CARTESIAN_POINT('Ctrl Pts',(141.335218967465,-5.81940089586769,-18.7074132579599));
#80390=CARTESIAN_POINT('Ctrl Pts',(141.315835564103,-7.57351425655799,-16.1431928920618));
#80391=CARTESIAN_POINT('Ctrl Pts',(141.323072531631,-11.4530715742594,-14.4578903667644));
#80392=CARTESIAN_POINT('Ctrl Pts',(141.339832522948,-13.8621755940366,-14.5396739647277));
#80393=CARTESIAN_POINT('Ctrl Pts',(141.349059636029,-15.0037376985838,-14.8321106819815));
#80394=CARTESIAN_POINT('Ctrl Pts',(158.900200939034,-5.48157966614799,-10.8530999549913));
#80395=CARTESIAN_POINT('Ctrl Pts',(158.897912832915,-5.08824189615433,-11.1564096405293));
#80396=CARTESIAN_POINT('Ctrl Pts',(158.88362144023,-4.03672678766422,-12.2427659670136));
#80397=CARTESIAN_POINT('Ctrl Pts',(158.810747035823,-2.61048388416648,-15.5254965007178));
#80398=CARTESIAN_POINT('Ctrl Pts',(158.727433552289,-2.66563056571491,-18.6626974800134));
#80399=CARTESIAN_POINT('Ctrl Pts',(158.677501178099,-3.15348645839912,-20.6221359368264));
#80400=CARTESIAN_POINT('Ctrl Pts',(158.932009582291,-5.45967120081002,-10.8243791764931));
#80401=CARTESIAN_POINT('Ctrl Pts',(158.930416716534,-5.0635967549265,-11.1295795919493));
#80402=CARTESIAN_POINT('Ctrl Pts',(158.920419579202,-4.00460884206074,-12.2221779464896));
#80403=CARTESIAN_POINT('Ctrl Pts',(158.869091522408,-2.57107410020526,-15.5201625939366));
#80404=CARTESIAN_POINT('Ctrl Pts',(158.806815191411,-2.63797081857116,-18.6664926300546));
#80405=CARTESIAN_POINT('Ctrl Pts',(158.767483782269,-3.13622100501925,-20.6263452062951));
#80406=CARTESIAN_POINT('Ctrl Pts',(158.982413267298,-5.40881538133815,-10.7577100281132));
#80407=CARTESIAN_POINT('Ctrl Pts',(158.981986233852,-5.00617131286099,-11.0670259566527));
#80408=CARTESIAN_POINT('Ctrl Pts',(158.979315752845,-3.92851688456229,-12.1725091485516));
#80409=CARTESIAN_POINT('Ctrl Pts',(158.965306397489,-2.46407740130744,-15.5013408988429));
#80410=CARTESIAN_POINT('Ctrl Pts',(158.946828836705,-2.53166450492611,-18.6752794966304));
#80411=CARTESIAN_POINT('Ctrl Pts',(158.934105907542,-3.03899473697198,-20.6500486997768));
#80412=CARTESIAN_POINT('Ctrl Pts',(159.,-5.35044541869311,-10.6811902563167));
#80413=CARTESIAN_POINT('Ctrl Pts',(159.000001718518,-4.94006024071246,-10.9949617076022));
#80414=CARTESIAN_POINT('Ctrl Pts',(158.999924341368,-3.83925785222158,-12.1137637882646));
#80415=CARTESIAN_POINT('Ctrl Pts',(158.999990369809,-2.32581588321333,-15.4734143434277));
#80416=CARTESIAN_POINT('Ctrl Pts',(158.999816470067,-2.36300502608751,-18.6852778006565));
#80417=CARTESIAN_POINT('Ctrl Pts',(159.,-2.86134373923737,-20.6933595184618));
#80418=CARTESIAN_POINT('Ctrl Pts',(159.,-5.3212536841056,-10.6429215172639));
#80419=CARTESIAN_POINT('Ctrl Pts',(159.,-4.90699614204386,-10.958920855577));
#80420=CARTESIAN_POINT('Ctrl Pts',(159.,-3.79463799060448,-12.0843726444514));
#80421=CARTESIAN_POINT('Ctrl Pts',(159.,-2.25665265374671,-15.4594257282765));
#80422=CARTESIAN_POINT('Ctrl Pts',(159.,-2.27857807033076,-18.6902253726123));
#80423=CARTESIAN_POINT('Ctrl Pts',(159.,-2.77223307638909,-20.715084449989));
#80424=CARTESIAN_POINT('Ctrl Pts',(159.,-4.99603773425357,-10.9105273455463));
#80425=CARTESIAN_POINT('Ctrl Pts',(159.,-5.12516101956932,-10.8514005237735));
#80426=CARTESIAN_POINT('Ctrl Pts',(158.993725032458,-5.25393493275618,-10.7896805376406));
#80427=CARTESIAN_POINT('Ctrl Pts',(158.9865805553,-5.38356518503846,-10.7246084263455));
#80428=CARTESIAN_POINT('Ctrl Pts',(158.900103550624,-5.4651123177601,-10.8658519867657));
#80429=CARTESIAN_POINT('Ctrl Pts',(158.89777930271,-5.07845377874636,-11.1665389098911));
#80430=CARTESIAN_POINT('Ctrl Pts',(158.883475935982,-4.0338790882016,-12.2493204115292));
#80431=CARTESIAN_POINT('Ctrl Pts',(158.810747035823,-2.61048388416648,-15.5254965007178));
#80432=CARTESIAN_POINT('Ctrl Pts',(158.727433552289,-2.66563056571491,-18.6626974800134));
#80433=CARTESIAN_POINT('Ctrl Pts',(158.677501178099,-3.15348645839912,-20.6221359368264));
#80434=CARTESIAN_POINT('Ctrl Pts',(158.677501178099,-3.15348645839912,-20.6221359368264));
#80435=CARTESIAN_POINT('Ctrl Pts',(156.381252820875,-3.8367747771134,-21.5101977970519));
#80436=CARTESIAN_POINT('Ctrl Pts',(150.573818453124,-5.06857870929353,-22.7186262210414));
#80437=CARTESIAN_POINT('Ctrl Pts',(144.528057503898,-5.40698027635754,-21.6917246298));
#80438=CARTESIAN_POINT('Ctrl Pts',(141.349059636028,-5.34311579304849,-20.409673339676));
#80439=CARTESIAN_POINT('Ctrl Pts',(158.718387254585,-3.16878056711171,-20.7189599683332));
#80440=CARTESIAN_POINT('Ctrl Pts',(156.40844718459,-3.84848380462859,-21.6089906795293));
#80441=CARTESIAN_POINT('Ctrl Pts',(150.569916786281,-5.06860951212775,-22.8138364111194));
#80442=CARTESIAN_POINT('Ctrl Pts',(144.506210304216,-5.39241544501344,-21.7665711562495));
#80443=CARTESIAN_POINT('Ctrl Pts',(141.323496046579,-5.32238907381613,-20.4713275147458));
#80444=CARTESIAN_POINT('Ctrl Pts',(158.782431558123,-3.11397975410553,-20.9324408777992));
#80445=CARTESIAN_POINT('Ctrl Pts',(156.446911120439,-3.7924047836726,-21.8190528430106));
#80446=CARTESIAN_POINT('Ctrl Pts',(150.55332346432,-5.00397080232419,-23.0006901114954));
#80447=CARTESIAN_POINT('Ctrl Pts',(144.463760791778,-5.31687736639789,-21.9063608518568));
#80448=CARTESIAN_POINT('Ctrl Pts',(141.277191290691,-5.24513644961931,-20.5844661011536));
#80449=CARTESIAN_POINT('Ctrl Pts',(158.773699287417,-2.92284752607861,-21.0592127969533));
#80450=CARTESIAN_POINT('Ctrl Pts',(156.43303299597,-3.60890596901209,-21.9389937074074));
#80451=CARTESIAN_POINT('Ctrl Pts',(150.529425631837,-4.83949631712008,-23.1010209113533));
#80452=CARTESIAN_POINT('Ctrl Pts',(144.438025586964,-5.17460835353068,-21.9824782290565));
#80453=CARTESIAN_POINT('Ctrl Pts',(141.252831675805,-5.11713793346312,-20.6471990838808));
#80454=CARTESIAN_POINT('Ctrl Pts',(158.752212389381,-2.82129914853757,-21.0817231128207));
#80455=CARTESIAN_POINT('Ctrl Pts',(156.415169556785,-3.51043054281809,-21.9597371783211));
#80456=CARTESIAN_POINT('Ctrl Pts',(150.518854599309,-4.75019250343027,-23.1187933032084));
#80457=CARTESIAN_POINT('Ctrl Pts',(144.431472367678,-5.0981359422299,-21.9983003417061));
#80458=CARTESIAN_POINT('Ctrl Pts',(141.247787610619,-5.04896191502908,-20.6617221419648));
#80459=CARTESIAN_POINT('Ctrl Pts',(158.677501178099,-3.15348645839912,-20.6221359368264));
#80460=CARTESIAN_POINT('Ctrl Pts',(156.381252820875,-3.8367747771134,-21.5101977970519));
#80461=CARTESIAN_POINT('Ctrl Pts',(150.573818453124,-5.06857870929353,-22.7186262210414));
#80462=CARTESIAN_POINT('Ctrl Pts',(144.528057503898,-5.40698027635754,-21.6917246298));
#80463=CARTESIAN_POINT('Ctrl Pts',(141.349059636028,-5.34311579304849,-20.409673339676));
#80464=CARTESIAN_POINT('Ctrl Pts',(141.247787610619,-5.04896191502908,-20.6617221419648));
#80465=CARTESIAN_POINT('Ctrl Pts',(144.431472367678,-5.0981359422299,-21.9983003417061));
#80466=CARTESIAN_POINT('Ctrl Pts',(150.518854599309,-4.75019250343027,-23.1187933032084));
#80467=CARTESIAN_POINT('Ctrl Pts',(156.415169556785,-3.51043054281809,-21.9597371783211));
#80468=CARTESIAN_POINT('Ctrl Pts',(158.752212389381,-2.82129914853757,-21.0817231128207));
#80469=CARTESIAN_POINT('Ctrl Pts',(141.349059636028,-15.0037376985771,-14.8321106819798));
#80470=CARTESIAN_POINT('Ctrl Pts',(143.733360778358,-15.8125231475547,-15.3543726670707));
#80471=CARTESIAN_POINT('Ctrl Pts',(149.65850090184,-17.0849972509199,-15.8333433835003));
#80472=CARTESIAN_POINT('Ctrl Pts',(155.615817811053,-16.852473851153,-14.423110502624));
#80473=CARTESIAN_POINT('Ctrl Pts',(158.677501178099,-16.2825503723881,-13.0420673518771));
#80474=CARTESIAN_POINT('Ctrl Pts',(141.323496046579,-15.0674951400532,-14.8449879041224));
#80475=CARTESIAN_POINT('Ctrl Pts',(143.710584542891,-15.8825387030768,-15.3761994825331));
#80476=CARTESIAN_POINT('Ctrl Pts',(149.650613765711,-17.1665313127827,-15.8777540499385));
#80477=CARTESIAN_POINT('Ctrl Pts',(155.638448157872,-16.9333423839598,-14.481940459732));
#80478=CARTESIAN_POINT('Ctrl Pts',(158.718387254585,-16.3587553890136,-13.1037244543038));
#80479=CARTESIAN_POINT('Ctrl Pts',(141.277191383292,-15.2041022649956,-14.834654170474));
#80480=CARTESIAN_POINT('Ctrl Pts',(143.667171376152,-16.0358136453275,-15.3769737905696));
#80481=CARTESIAN_POINT('Ctrl Pts',(149.62768779964,-17.3562202641115,-15.909779931237));
#80482=CARTESIAN_POINT('Ctrl Pts',(155.668384443696,-17.1425271110913,-14.5374654411864));
#80483=CARTESIAN_POINT('Ctrl Pts',(158.782430907772,-16.5710356244403,-13.1630045703251));
#80484=CARTESIAN_POINT('Ctrl Pts',(141.252831675805,-15.322429956904,-14.7551709869884));
#80485=CARTESIAN_POINT('Ctrl Pts',(143.641779953398,-16.1681865034062,-15.2932407014948));
#80486=CARTESIAN_POINT('Ctrl Pts',(149.60298988863,-17.520882048225,-15.8183486395124));
#80487=CARTESIAN_POINT('Ctrl Pts',(155.652791642657,-17.3349041445575,-14.4395877746157));
#80488=CARTESIAN_POINT('Ctrl Pts',(158.773699287417,-16.7763895028246,-13.0608666074492));
#80489=CARTESIAN_POINT('Ctrl Pts',(141.247787610619,-15.3690953033625,-14.7033903521377));
#80490=CARTESIAN_POINT('Ctrl Pts',(143.635603997599,-16.2188068453664,-15.236558438444));
#80491=CARTESIAN_POINT('Ctrl Pts',(149.593137985275,-17.579849295519,-15.751170402598));
#80492=CARTESIAN_POINT('Ctrl Pts',(155.636136052898,-17.4010840024374,-14.3652699144507));
#80493=CARTESIAN_POINT('Ctrl Pts',(158.752212389381,-16.8466581969835,-12.9841782907193));
#80494=CARTESIAN_POINT('',(158.677501178099,-16.2825503723881,-13.0420673518771));
#80495=CARTESIAN_POINT('Ctrl Pts',(141.349059636028,-15.0037376985771,-14.8321106819798));
#80496=CARTESIAN_POINT('Ctrl Pts',(143.733360778358,-15.8125231475547,-15.3543726670707));
#80497=CARTESIAN_POINT('Ctrl Pts',(149.65850090184,-17.0849972509199,-15.8333433835003));
#80498=CARTESIAN_POINT('Ctrl Pts',(155.615817811053,-16.852473851153,-14.423110502624));
#80499=CARTESIAN_POINT('Ctrl Pts',(158.677501178099,-16.2825503723881,-13.0420673518771));
#80500=CARTESIAN_POINT('Origin',(158.6,-16.5536728370359,-12.7583664943589));
#80501=CARTESIAN_POINT('Origin',(158.6,-16.5536728370359,-12.7583664943589));
#80502=CARTESIAN_POINT('Origin',(158.6,-16.5536728370359,-12.7583664943589));
#80503=CARTESIAN_POINT('Origin',(150.,0.,0.));
#80504=CARTESIAN_POINT('',(150.,-3.77668789453883,-11.3901987931398));
#80505=CARTESIAN_POINT('Origin',(150.,-1.33226762955019E-14,0.));
#80506=CARTESIAN_POINT('',(150.,-1.33226762955019E-14,-23.));
#80507=CARTESIAN_POINT('Origin',(150.,-1.33226762955019E-14,0.));
#80508=CARTESIAN_POINT('Ctrl Pts',(158.677501178099,-16.2825503723881,-13.0420673518771));
#80509=CARTESIAN_POINT('Ctrl Pts',(158.71495181987,-15.192764113758,-11.9903680096648));
#80510=CARTESIAN_POINT('Ctrl Pts',(158.781809873649,-13.0560745106574,-10.5613269702318));
#80511=CARTESIAN_POINT('Ctrl Pts',(158.866157601674,-9.61661358482788,-9.59694294254089));
#80512=CARTESIAN_POINT('Ctrl Pts',(158.895624704489,-7.57696047183816,-9.79576406212931));
#80513=CARTESIAN_POINT('Ctrl Pts',(158.900200939034,-6.65827043776023,-10.173737221248));
#80514=CARTESIAN_POINT('Ctrl Pts',(158.767483782269,-16.2948284333693,-13.0292196653766));
#80515=CARTESIAN_POINT('Ctrl Pts',(158.796983411277,-15.2086711883374,-11.9706134855125));
#80516=CARTESIAN_POINT('Ctrl Pts',(158.847731347736,-13.0722241734835,-10.5294251241165));
#80517=CARTESIAN_POINT('Ctrl Pts',(158.908274661215,-9.62062110267638,-9.5578506046531));
#80518=CARTESIAN_POINT('Ctrl Pts',(158.928823835247,-7.56905332618701,-9.75958103968308));
#80519=CARTESIAN_POINT('Ctrl Pts',(158.932009582291,-6.64435174663334,-10.1404035444583));
#80520=CARTESIAN_POINT('Ctrl Pts',(158.934104852847,-16.3639699937563,-12.9568703674406));
#80521=CARTESIAN_POINT('Ctrl Pts',(158.943647396539,-15.2715289040604,-11.8867723722052));
#80522=CARTESIAN_POINT('Ctrl Pts',(158.959073130834,-13.1176119648907,-10.4315631799996));
#80523=CARTESIAN_POINT('Ctrl Pts',(158.976089907337,-9.62865081747197,-9.46200255793715));
#80524=CARTESIAN_POINT('Ctrl Pts',(158.981559094319,-7.55044201207681,-9.67494055595002));
#80525=CARTESIAN_POINT('Ctrl Pts',(158.982413165375,-6.61204246539703,-10.0630265031676));
#80526=CARTESIAN_POINT('Ctrl Pts',(159.,-16.4903031630138,-12.82467612637));
#80527=CARTESIAN_POINT('Ctrl Pts',(158.999862347547,-15.3728522317907,-11.7479258592004));
#80528=CARTESIAN_POINT('Ctrl Pts',(158.999966995003,-13.1780366342351,-10.2945794162384));
#80529=CARTESIAN_POINT('Ctrl Pts',(158.999868817248,-9.63709524450701,-9.34658683117197));
#80530=CARTESIAN_POINT('Ctrl Pts',(159.000003437053,-7.52881731858658,-9.57717831922963));
#80531=CARTESIAN_POINT('Ctrl Pts',(159.,-6.57495939527851,-9.97421678230863));
#80532=CARTESIAN_POINT('Ctrl Pts',(159.,-16.5536728370359,-12.7583664943589));
#80533=CARTESIAN_POINT('Ctrl Pts',(159.,-15.423567841049,-11.6783667562432));
#80534=CARTESIAN_POINT('Ctrl Pts',(159.,-13.2082488270869,-10.226020745615));
#80535=CARTESIAN_POINT('Ctrl Pts',(159.,-9.64128250186343,-9.28888713869177));
#80536=CARTESIAN_POINT('Ctrl Pts',(159.,-7.51800270098317,-9.52828389982868));
#80537=CARTESIAN_POINT('Ctrl Pts',(159.,-6.5564135623818,-9.92980162904894));
#80538=CARTESIAN_POINT('Ctrl Pts',(158.677501178099,-16.2825503723881,-13.0420673518771));
#80539=CARTESIAN_POINT('Ctrl Pts',(158.71495181987,-15.192764113758,-11.9903680096648));
#80540=CARTESIAN_POINT('Ctrl Pts',(158.781809873649,-13.0560745106574,-10.5613269702318));
#80541=CARTESIAN_POINT('Ctrl Pts',(158.865989166098,-9.62348190950231,-9.59886873927353));
#80542=CARTESIAN_POINT('Ctrl Pts',(158.895418523778,-7.59121514189453,-9.79438361628517));
#80543=CARTESIAN_POINT('Ctrl Pts',(158.900103499495,-6.67754798826903,-10.1658528042907));
#80544=CARTESIAN_POINT('Ctrl Pts',(158.9865805553,-6.59600075033667,-10.0246084263455));
#80545=CARTESIAN_POINT('Ctrl Pts',(158.993842160356,-6.71915644896929,-9.94357433044469));
#80546=CARTESIAN_POINT('Ctrl Pts',(159.,-6.83740198055336,-9.86251881797497));
#80547=CARTESIAN_POINT('Ctrl Pts',(159.,-6.95077498280114,-9.78195926890241));
#80548=CARTESIAN_POINT('Origin',(145.,-2.27826388829055E-15,-3.94606880756866E-15));
#80549=CARTESIAN_POINT('Ctrl Pts',(158.671029640456,-5.5937822173509,-11.088715006927));
#80550=CARTESIAN_POINT('Ctrl Pts',(158.642904819311,-5.80046894549335,-10.9693843687961));
#80551=CARTESIAN_POINT('Ctrl Pts',(158.629834412239,-6.00445828013108,-10.8516110715312));
#80552=CARTESIAN_POINT('Ctrl Pts',(158.629834412239,-6.39554171986893,-10.6258189423229));
#80553=CARTESIAN_POINT('Ctrl Pts',(158.642904819311,-6.59953105450667,-10.508045645058));
#80554=CARTESIAN_POINT('Ctrl Pts',(158.671029640456,-6.80621778264911,-10.388715006927));
#80555=CARTESIAN_POINT('Ctrl Pts',(158.666552508001,-19.866378214229,7.69531573590557));
#80556=CARTESIAN_POINT('Ctrl Pts',(158.70506309762,-18.3356178296977,7.31472446391733));
#80557=CARTESIAN_POINT('Ctrl Pts',(158.774612832515,-15.8996513054051,6.19397172155974));
#80558=CARTESIAN_POINT('Ctrl Pts',(158.863837927697,-13.1859943058499,3.64218218391035));
#80559=CARTESIAN_POINT('Ctrl Pts',(158.895432323316,-12.2774103837893,1.70534981330175));
#80560=CARTESIAN_POINT('Ctrl Pts',(158.900200939034,-12.1398501039082,0.679362733743279));
#80561=CARTESIAN_POINT('Ctrl Pts',(158.758824046361,-19.8625594015549,7.71040940270194));
#80562=CARTESIAN_POINT('Ctrl Pts',(158.789386050929,-18.3279118906777,7.33717508378105));
#80563=CARTESIAN_POINT('Ctrl Pts',(158.842478617173,-15.8812263896621,6.22396382322617));
#80564=CARTESIAN_POINT('Ctrl Pts',(158.906660488852,-13.1544214007013,3.66586377475453));
#80565=CARTESIAN_POINT('Ctrl Pts',(158.928689909036,-12.2421440184425,1.71687228995628));
#80566=CARTESIAN_POINT('Ctrl Pts',(158.932009582291,-12.1040229474433,0.683975632034815));
#80567=CARTESIAN_POINT('Ctrl Pts',(158.931293562486,-19.8383310071993,7.80617092405118));
#80568=CARTESIAN_POINT('Ctrl Pts',(158.941286887852,-18.2899779002915,7.43431238755036));
#80569=CARTESIAN_POINT('Ctrl Pts',(158.957561307978,-15.8208930349454,6.31415574843049));
#80570=CARTESIAN_POINT('Ctrl Pts',(158.975659787015,-13.0757115695514,3.72243477075486));
#80571=CARTESIAN_POINT('Ctrl Pts',(158.981523215389,-12.1595610473647,1.74372603630125));
#80572=CARTESIAN_POINT('Ctrl Pts',(158.982413190896,-12.0208578329538,0.694683493121148));
#80573=CARTESIAN_POINT('Ctrl Pts',(159.,-19.7925863683044,7.98697432975182));
#80574=CARTESIAN_POINT('Ctrl Pts',(158.999850139758,-18.2238049379904,7.59681086660833));
#80575=CARTESIAN_POINT('Ctrl Pts',(158.999964678301,-15.7334734686309,6.43919229122095));
#80576=CARTESIAN_POINT('Ctrl Pts',(158.999857039542,-12.9799611868347,3.78961117372722));
#80577=CARTESIAN_POINT('Ctrl Pts',(159.000003581543,-12.0640831050459,1.77463059337494));
#80578=CARTESIAN_POINT('Ctrl Pts',(159.,-11.9254048139716,0.706973474008048));
#80579=CARTESIAN_POINT('Ctrl Pts',(159.,-19.7696341894082,8.07769167309343));
#80580=CARTESIAN_POINT('Ctrl Pts',(159.,-18.1906199145079,7.67818903355298));
#80581=CARTESIAN_POINT('Ctrl Pts',(159.,-15.6897004416897,6.50174671393537));
#80582=CARTESIAN_POINT('Ctrl Pts',(159.,-12.9320743783783,3.82316018062639));
#80583=CARTESIAN_POINT('Ctrl Pts',(159.,-12.0163314172826,1.79008769222358));
#80584=CARTESIAN_POINT('Ctrl Pts',(159.,-11.8776672464874,0.713119888214995));
#80585=CARTESIAN_POINT('Ctrl Pts',(158.9865805553,-11.9795659353751,0.700000000000001));
#80586=CARTESIAN_POINT('Ctrl Pts',(158.993732330744,-11.9710962675166,0.844947063660498));
#80587=CARTESIAN_POINT('Ctrl Pts',(159.,-11.9601689398254,0.987181575154897));
#80588=CARTESIAN_POINT('Ctrl Pts',(159.,-11.9468127170547,1.12856807664393));
#80589=CARTESIAN_POINT('Origin',(158.6,2.77223307638908,20.715084449989));
#80590=CARTESIAN_POINT('',(158.677501178099,3.15348645839912,20.6221359368264));
#80591=CARTESIAN_POINT('Origin',(158.6,2.77223307638908,20.715084449989));
#80592=CARTESIAN_POINT('Origin',(158.6,2.77223307638908,20.715084449989));
#80593=CARTESIAN_POINT('Origin',(150.,-1.33226762955019E-14,0.));
#80594=CARTESIAN_POINT('Ctrl Pts',(141.247787610619,5.04896191502908,20.6617221419648));
#80595=CARTESIAN_POINT('Ctrl Pts',(144.431472367678,5.09813594222989,21.9983003417061));
#80596=CARTESIAN_POINT('Ctrl Pts',(150.518854599309,4.75019250343027,23.1187933032084));
#80597=CARTESIAN_POINT('Ctrl Pts',(156.415169556785,3.51043054281806,21.9597371783211));
#80598=CARTESIAN_POINT('Ctrl Pts',(158.752212389381,2.82129914853755,21.0817231128206));
#80599=CARTESIAN_POINT('',(150.,-1.33226762955019E-14,23.));
#80600=CARTESIAN_POINT('Origin',(150.,-1.33226762955019E-14,0.));
#80601=CARTESIAN_POINT('Ctrl Pts',(158.677501178099,3.1534864583991,20.6221359368264));
#80602=CARTESIAN_POINT('Ctrl Pts',(156.381252820875,3.83677477711337,21.5101977970519));
#80603=CARTESIAN_POINT('Ctrl Pts',(150.573818453124,5.06857870929353,22.7186262210413));
#80604=CARTESIAN_POINT('Ctrl Pts',(144.528057503898,5.40698027635753,21.6917246298));
#80605=CARTESIAN_POINT('Ctrl Pts',(141.349059636028,5.34311579304849,20.409673339676));
#80606=CARTESIAN_POINT('Ctrl Pts',(158.718387254585,3.16878056711168,20.7189599683332));
#80607=CARTESIAN_POINT('Ctrl Pts',(156.40844718459,3.84848380462856,21.6089906795292));
#80608=CARTESIAN_POINT('Ctrl Pts',(150.569916786281,5.06860951212774,22.8138364111194));
#80609=CARTESIAN_POINT('Ctrl Pts',(144.506210304216,5.39241544501344,21.7665711562495));
#80610=CARTESIAN_POINT('Ctrl Pts',(141.323496046579,5.32238907381613,20.4713275147458));
#80611=CARTESIAN_POINT('Ctrl Pts',(158.782431558123,3.1139797541055,20.9324408777991));
#80612=CARTESIAN_POINT('Ctrl Pts',(156.446911120439,3.79240478367256,21.8190528430106));
#80613=CARTESIAN_POINT('Ctrl Pts',(150.55332346432,5.00397080232418,23.0006901114954));
#80614=CARTESIAN_POINT('Ctrl Pts',(144.463760791778,5.31687736639788,21.9063608518568));
#80615=CARTESIAN_POINT('Ctrl Pts',(141.277191290691,5.2451364496193,20.5844661011536));
#80616=CARTESIAN_POINT('Ctrl Pts',(158.773699287417,2.92284752607859,21.0592127969533));
#80617=CARTESIAN_POINT('Ctrl Pts',(156.43303299597,3.60890596901206,21.9389937074074));
#80618=CARTESIAN_POINT('Ctrl Pts',(150.529425631836,4.83949631712007,23.1010209113533));
#80619=CARTESIAN_POINT('Ctrl Pts',(144.438025586964,5.17460835353068,21.9824782290565));
#80620=CARTESIAN_POINT('Ctrl Pts',(141.252831675805,5.11713793346312,20.6471990838808));
#80621=CARTESIAN_POINT('Ctrl Pts',(158.752212389381,2.82129914853755,21.0817231128206));
#80622=CARTESIAN_POINT('Ctrl Pts',(156.415169556785,3.51043054281806,21.9597371783211));
#80623=CARTESIAN_POINT('Ctrl Pts',(150.518854599309,4.75019250343027,23.1187933032084));
#80624=CARTESIAN_POINT('Ctrl Pts',(144.431472367678,5.09813594222989,21.9983003417061));
#80625=CARTESIAN_POINT('Ctrl Pts',(141.247787610619,5.04896191502908,20.6617221419648));
#80626=CARTESIAN_POINT('Ctrl Pts',(158.677501178099,3.1534864583991,20.6221359368264));
#80627=CARTESIAN_POINT('Ctrl Pts',(156.381252820875,3.83677477711337,21.5101977970519));
#80628=CARTESIAN_POINT('Ctrl Pts',(150.573818453124,5.06857870929353,22.7186262210413));
#80629=CARTESIAN_POINT('Ctrl Pts',(144.528057503898,5.40698027635753,21.6917246298));
#80630=CARTESIAN_POINT('Ctrl Pts',(141.349059636028,5.34311579304849,20.409673339676));
#80631=CARTESIAN_POINT('Ctrl Pts',(158.900200939034,5.48157966614799,10.8530999549913));
#80632=CARTESIAN_POINT('Ctrl Pts',(158.89791282087,5.08823982556231,11.1564112371993));
#80633=CARTESIAN_POINT('Ctrl Pts',(158.883621246827,4.03672055481242,12.2427746659606));
#80634=CARTESIAN_POINT('Ctrl Pts',(158.810747522317,2.61049296583572,15.52547614197));
#80635=CARTESIAN_POINT('Ctrl Pts',(158.727434679478,2.66561955271069,18.6626532470661));
#80636=CARTESIAN_POINT('Ctrl Pts',(158.677501178099,3.15348645839911,20.6221359368264));
#80637=CARTESIAN_POINT('Ctrl Pts',(158.932009582291,5.45967120081001,10.8243791764931));
#80638=CARTESIAN_POINT('Ctrl Pts',(158.930416708149,5.06359466992819,11.1295811985724));
#80639=CARTESIAN_POINT('Ctrl Pts',(158.920419452116,4.00460256967265,12.2221867084119));
#80640=CARTESIAN_POINT('Ctrl Pts',(158.869091858532,2.57108321899853,15.520142121643));
#80641=CARTESIAN_POINT('Ctrl Pts',(158.80681607929,2.63795957092305,18.6664483877589));
#80642=CARTESIAN_POINT('Ctrl Pts',(158.767483782269,3.13622100501924,20.6263452062951));
#80643=CARTESIAN_POINT('Ctrl Pts',(158.982413267298,5.40881538133815,10.7577100281132));
#80644=CARTESIAN_POINT('Ctrl Pts',(158.981986231604,5.00616919327914,11.0670275849405));
#80645=CARTESIAN_POINT('Ctrl Pts',(158.97931572272,3.92851048163637,12.1725180025924));
#80646=CARTESIAN_POINT('Ctrl Pts',(158.965306485669,2.46408671880266,15.5013202288941));
#80647=CARTESIAN_POINT('Ctrl Pts',(158.946829123917,2.53165305230235,18.6752349176023));
#80648=CARTESIAN_POINT('Ctrl Pts',(158.934105907542,3.03899473697196,20.6500486997768));
#80649=CARTESIAN_POINT('Ctrl Pts',(159.,5.3504454186931,10.6811902563167));
#80650=CARTESIAN_POINT('Ctrl Pts',(159.000001718527,4.94005808038019,10.9949633593446));
#80651=CARTESIAN_POINT('Ctrl Pts',(158.999924341255,3.83925127335527,12.1137726841572));
#80652=CARTESIAN_POINT('Ctrl Pts',(158.999990369687,2.32582552868827,15.4733935254209));
#80653=CARTESIAN_POINT('Ctrl Pts',(158.999816465924,2.36299377644097,18.6852324696217));
#80654=CARTESIAN_POINT('Ctrl Pts',(159.,2.86134373923735,20.6933595184618));
#80655=CARTESIAN_POINT('Ctrl Pts',(159.,5.32125368410559,10.6429215172639));
#80656=CARTESIAN_POINT('Ctrl Pts',(159.,4.90699396132686,10.9589225190473));
#80657=CARTESIAN_POINT('Ctrl Pts',(159.,3.79463132400802,12.0843815608045));
#80658=CARTESIAN_POINT('Ctrl Pts',(159.,2.25666246318025,15.4594048368281));
#80659=CARTESIAN_POINT('Ctrl Pts',(159.,2.27856692641562,18.6901796628404));
#80660=CARTESIAN_POINT('Ctrl Pts',(159.,2.77223307638908,20.715084449989));
#80661=CARTESIAN_POINT('',(158.9865805553,5.38356518503846,10.7246084263455));
#80662=CARTESIAN_POINT('Ctrl Pts',(159.,4.99603773425357,10.9105273455463));
#80663=CARTESIAN_POINT('Ctrl Pts',(159.,5.1251610195845,10.8514005237665));
#80664=CARTESIAN_POINT('Ctrl Pts',(158.993725032394,5.25393493391408,10.7896805370593));
#80665=CARTESIAN_POINT('Ctrl Pts',(158.9865805553,5.38356518503846,10.7246084263455));
#80666=CARTESIAN_POINT('',(158.90010356288,5.46511181578879,10.8658513339894));
#80667=CARTESIAN_POINT('Ctrl Pts',(158.900103547021,5.46511172075857,10.8658524512155));
#80668=CARTESIAN_POINT('Ctrl Pts',(158.914774492448,5.4567146376521,10.8513079356306));
#80669=CARTESIAN_POINT('Ctrl Pts',(158.927982071049,5.44773161858671,10.8357527140535));
#80670=CARTESIAN_POINT('Ctrl Pts',(158.939638804157,5.43827616160656,10.8193759337943));
#80671=CARTESIAN_POINT('Ctrl Pts',(158.951368187587,5.42876177370791,10.8028970856281));
#80672=CARTESIAN_POINT('Ctrl Pts',(158.961528099479,5.4187683334774,10.7855854386424));
#80673=CARTESIAN_POINT('Ctrl Pts',(158.969987633786,5.40839177262983,10.7676110683556));
#80674=CARTESIAN_POINT('Ctrl Pts',(158.971443507175,5.4066059817986,10.7645177057158));
#80675=CARTESIAN_POINT('Ctrl Pts',(158.972848903058,5.40480881173085,10.7614046810949));
#80676=CARTESIAN_POINT('Ctrl Pts',(158.974203003918,5.40300071689055,10.7582728269582));
#80677=CARTESIAN_POINT('Ctrl Pts',(158.978981150563,5.39662058483742,10.7472216129857));
#80678=CARTESIAN_POINT('Ctrl Pts',(158.983100437627,5.39013241397557,10.7359837622485));
#80679=CARTESIAN_POINT('Ctrl Pts',(158.986559824909,5.38356357140903,10.7246063109672));
#80680=CARTESIAN_POINT('Ctrl Pts',(158.90010355061,5.46511231785056,10.8658519868838));
#80681=CARTESIAN_POINT('Ctrl Pts',(158.89777928969,5.07845172105258,11.1665405189834));
#80682=CARTESIAN_POINT('Ctrl Pts',(158.883475744701,4.03387290090986,12.2493290179738));
#80683=CARTESIAN_POINT('Ctrl Pts',(158.810747522317,2.61049296583572,15.52547614197));
#80684=CARTESIAN_POINT('Ctrl Pts',(158.727434679478,2.66561955271069,18.6626532470661));
#80685=CARTESIAN_POINT('Ctrl Pts',(158.677501178099,3.15348645839911,20.6221359368264));
#80686=CARTESIAN_POINT('Ctrl Pts',(141.349059636028,15.0037376985771,14.8321106819798));
#80687=CARTESIAN_POINT('Ctrl Pts',(143.733360778358,15.8125231475547,15.3543726670707));
#80688=CARTESIAN_POINT('Ctrl Pts',(149.65850090184,17.0849972509199,15.8333433835003));
#80689=CARTESIAN_POINT('Ctrl Pts',(155.615817811053,16.852473851153,14.423110502624));
#80690=CARTESIAN_POINT('Ctrl Pts',(158.677501178099,16.2825503723881,13.0420673518771));
#80691=CARTESIAN_POINT('Ctrl Pts',(141.323496046579,15.0674951400532,14.8449879041224));
#80692=CARTESIAN_POINT('Ctrl Pts',(143.710584542892,15.8825387030768,15.3761994825331));
#80693=CARTESIAN_POINT('Ctrl Pts',(149.650613765711,17.1665313127827,15.8777540499385));
#80694=CARTESIAN_POINT('Ctrl Pts',(155.638448157872,16.9333423839598,14.481940459732));
#80695=CARTESIAN_POINT('Ctrl Pts',(158.718387254585,16.3587553890136,13.1037244543038));
#80696=CARTESIAN_POINT('Ctrl Pts',(141.277191383292,15.2041022649956,14.834654170474));
#80697=CARTESIAN_POINT('Ctrl Pts',(143.667171376152,16.0358136453275,15.3769737905696));
#80698=CARTESIAN_POINT('Ctrl Pts',(149.62768779964,17.3562202641115,15.909779931237));
#80699=CARTESIAN_POINT('Ctrl Pts',(155.668384443696,17.1425271110913,14.5374654411864));
#80700=CARTESIAN_POINT('Ctrl Pts',(158.782430907772,16.5710356244403,13.1630045703251));
#80701=CARTESIAN_POINT('Ctrl Pts',(141.252831675805,15.322429956904,14.7551709869884));
#80702=CARTESIAN_POINT('Ctrl Pts',(143.641779953398,16.1681865034062,15.2932407014948));
#80703=CARTESIAN_POINT('Ctrl Pts',(149.60298988863,17.520882048225,15.8183486395124));
#80704=CARTESIAN_POINT('Ctrl Pts',(155.652791642657,17.3349041445575,14.4395877746158));
#80705=CARTESIAN_POINT('Ctrl Pts',(158.773699287417,16.7763895028246,13.0608666074492));
#80706=CARTESIAN_POINT('Ctrl Pts',(141.247787610619,15.3690953033624,14.7033903521377));
#80707=CARTESIAN_POINT('Ctrl Pts',(143.635603997599,16.2188068453664,15.236558438444));
#80708=CARTESIAN_POINT('Ctrl Pts',(149.593137985275,17.579849295519,15.751170402598));
#80709=CARTESIAN_POINT('Ctrl Pts',(155.636136052898,17.4010840024374,14.3652699144507));
#80710=CARTESIAN_POINT('Ctrl Pts',(158.752212389381,16.8466581969835,12.9841782907193));
#80711=CARTESIAN_POINT('',(158.677501178099,16.2825503723881,13.0420673518771));
#80712=CARTESIAN_POINT('Ctrl Pts',(141.349059636028,15.0037376985771,14.8321106819798));
#80713=CARTESIAN_POINT('Ctrl Pts',(143.733360778358,15.8125231475547,15.3543726670707));
#80714=CARTESIAN_POINT('Ctrl Pts',(149.65850090184,17.0849972509199,15.8333433835003));
#80715=CARTESIAN_POINT('Ctrl Pts',(155.615817811053,16.852473851153,14.423110502624));
#80716=CARTESIAN_POINT('Ctrl Pts',(158.677501178099,16.2825503723881,13.0420673518771));
#80717=CARTESIAN_POINT('',(158.752212389381,16.8466581969835,12.9841782907193));
#80718=CARTESIAN_POINT('Origin',(158.6,16.5536728370359,12.7583664943589));
#80719=CARTESIAN_POINT('Ctrl Pts',(158.752212389381,16.8466581969835,12.9841782907193));
#80720=CARTESIAN_POINT('Ctrl Pts',(155.636136052898,17.4010840024374,14.3652699144507));
#80721=CARTESIAN_POINT('Ctrl Pts',(149.593137985275,17.579849295519,15.751170402598));
#80722=CARTESIAN_POINT('Ctrl Pts',(143.635603997599,16.2188068453664,15.236558438444));
#80723=CARTESIAN_POINT('Ctrl Pts',(141.247787610619,15.3690953033624,14.7033903521377));
#80724=CARTESIAN_POINT('Origin',(158.6,16.5536728370359,12.7583664943589));
#80725=CARTESIAN_POINT('Origin',(158.6,16.5536728370359,12.7583664943589));
#80726=CARTESIAN_POINT('Origin',(158.6,16.5536728370359,12.7583664943589));
#80727=CARTESIAN_POINT('Origin',(150.,0.,0.));
#80728=CARTESIAN_POINT('',(150.,3.77668789453883,11.3901987931398));
#80729=CARTESIAN_POINT('',(150.,5.38356518503846,10.7246084263455));
#80730=CARTESIAN_POINT('Ctrl Pts',(158.677501178099,16.2825503723881,13.0420673518771));
#80731=CARTESIAN_POINT('Ctrl Pts',(158.71495181987,15.192764113758,11.9903680096648));
#80732=CARTESIAN_POINT('Ctrl Pts',(158.781809873649,13.0560745106574,10.5613269702317));
#80733=CARTESIAN_POINT('Ctrl Pts',(158.866157601674,9.61661358482787,9.59694294254089));
#80734=CARTESIAN_POINT('Ctrl Pts',(158.895624704489,7.57696047183815,9.79576406212931));
#80735=CARTESIAN_POINT('Ctrl Pts',(158.900200939034,6.65827043776023,10.173737221248));
#80736=CARTESIAN_POINT('Ctrl Pts',(158.767483782269,16.2948284333693,13.0292196653766));
#80737=CARTESIAN_POINT('Ctrl Pts',(158.796983411277,15.2086711883374,11.9706134855125));
#80738=CARTESIAN_POINT('Ctrl Pts',(158.847731347736,13.0722241734834,10.5294251241164));
#80739=CARTESIAN_POINT('Ctrl Pts',(158.908274661215,9.62062110267636,9.5578506046531));
#80740=CARTESIAN_POINT('Ctrl Pts',(158.928823835247,7.569053326187,9.75958103968308));
#80741=CARTESIAN_POINT('Ctrl Pts',(158.932009582291,6.64435174663334,10.1404035444583));
#80742=CARTESIAN_POINT('Ctrl Pts',(158.934104852847,16.3639699937563,12.9568703674406));
#80743=CARTESIAN_POINT('Ctrl Pts',(158.943647396539,15.2715289040604,11.8867723722052));
#80744=CARTESIAN_POINT('Ctrl Pts',(158.959073130834,13.1176119648907,10.4315631799996));
#80745=CARTESIAN_POINT('Ctrl Pts',(158.976089907337,9.62865081747196,9.46200255793715));
#80746=CARTESIAN_POINT('Ctrl Pts',(158.981559094319,7.5504420120768,9.67494055595002));
#80747=CARTESIAN_POINT('Ctrl Pts',(158.982413165375,6.61204246539703,10.0630265031676));
#80748=CARTESIAN_POINT('Ctrl Pts',(159.,16.4903031630138,12.82467612637));
#80749=CARTESIAN_POINT('Ctrl Pts',(158.999862347547,15.3728522317907,11.7479258592004));
#80750=CARTESIAN_POINT('Ctrl Pts',(158.999966995003,13.1780366342351,10.2945794162384));
#80751=CARTESIAN_POINT('Ctrl Pts',(158.999868817248,9.63709524450698,9.34658683117197));
#80752=CARTESIAN_POINT('Ctrl Pts',(159.000003437053,7.52881731858657,9.57717831922963));
#80753=CARTESIAN_POINT('Ctrl Pts',(159.,6.57495939527851,9.97421678230863));
#80754=CARTESIAN_POINT('Ctrl Pts',(159.,16.5536728370359,12.7583664943589));
#80755=CARTESIAN_POINT('Ctrl Pts',(159.,15.423567841049,11.6783667562432));
#80756=CARTESIAN_POINT('Ctrl Pts',(159.,13.2082488270869,10.2260207456149));
#80757=CARTESIAN_POINT('Ctrl Pts',(159.,9.64128250186341,9.28888713869177));
#80758=CARTESIAN_POINT('Ctrl Pts',(159.,7.51800270098316,9.52828389982868));
#80759=CARTESIAN_POINT('Ctrl Pts',(159.,6.55641356238179,9.92980162904894));
#80760=CARTESIAN_POINT('',(158.90010356288,6.67754738108544,10.1658513339903));
#80761=CARTESIAN_POINT('Ctrl Pts',(158.677501178099,16.2825503723881,13.0420673518771));
#80762=CARTESIAN_POINT('Ctrl Pts',(158.71495181987,15.192764113758,11.9903680096648));
#80763=CARTESIAN_POINT('Ctrl Pts',(158.781809873649,13.0560745106574,10.5613269702317));
#80764=CARTESIAN_POINT('Ctrl Pts',(158.865989166098,9.6234819095023,9.59886873927354));
#80765=CARTESIAN_POINT('Ctrl Pts',(158.895418523778,7.59121514189453,9.79438361628517));
#80766=CARTESIAN_POINT('Ctrl Pts',(158.900103499495,6.67754798826903,10.1658528042907));
#80767=CARTESIAN_POINT('',(158.9865805553,6.59600075033667,10.0246084263455));
#80768=CARTESIAN_POINT('Ctrl Pts',(158.986559783722,6.59599971918856,10.0246059568635));
#80769=CARTESIAN_POINT('Ctrl Pts',(158.983100403821,6.60256843395615,10.0359834218172));
#80770=CARTESIAN_POINT('Ctrl Pts',(158.978981130879,6.60905654044642,10.0472212590995));
#80771=CARTESIAN_POINT('Ctrl Pts',(158.974203007079,6.61543699190686,10.0582722491853));
#80772=CARTESIAN_POINT('Ctrl Pts',(158.966341570957,6.62593473405238,10.0764544178129));
#80773=CARTESIAN_POINT('Ctrl Pts',(158.956755276001,6.63606717349649,10.0940017110898));
#80774=CARTESIAN_POINT('Ctrl Pts',(158.945583009388,6.64573620403175,10.1107496127464));
#80775=CARTESIAN_POINT('Ctrl Pts',(158.934457797467,6.65536451111572,10.1274269765807));
#80776=CARTESIAN_POINT('Ctrl Pts',(158.921759191497,6.66453378582656,10.1433127600992));
#80777=CARTESIAN_POINT('Ctrl Pts',(158.907581310123,6.67313882951052,10.1582194335511));
#80778=CARTESIAN_POINT('Ctrl Pts',(158.905132791899,6.67462491940831,10.1607938140703));
#80779=CARTESIAN_POINT('Ctrl Pts',(158.902640065462,6.6760941505975,10.1633389084979));
#80780=CARTESIAN_POINT('Ctrl Pts',(158.900103510001,6.67754593940625,10.1658536372963));
#80781=CARTESIAN_POINT('Ctrl Pts',(158.9865805553,6.59600075033667,10.0246084263455));
#80782=CARTESIAN_POINT('Ctrl Pts',(158.993842160356,6.71915644896927,9.9435743304447));
#80783=CARTESIAN_POINT('Ctrl Pts',(159.,6.83740198055335,9.86251881797498));
#80784=CARTESIAN_POINT('Ctrl Pts',(159.,6.95077498280114,9.78195926890241));
#80785=CARTESIAN_POINT('Origin',(158.6,-1.33226762955019E-14,0.));
#80786=CARTESIAN_POINT('Origin',(158.752212389381,-1.33226762955019E-14,
0.));
#80787=CARTESIAN_POINT('Ctrl Pts',(158.900200939034,12.1398501039078,0.679362733740281));
#80788=CARTESIAN_POINT('Ctrl Pts',(158.897912817069,12.2058555689279,1.1716614870554));
#80789=CARTESIAN_POINT('Ctrl Pts',(158.883620879071,12.6209295917709,2.62549313766));
#80790=CARTESIAN_POINT('Ctrl Pts',(158.810748226743,14.7506827036296,5.50198934279456));
#80791=CARTESIAN_POINT('Ctrl Pts',(158.727432361316,17.4952316963631,7.02285824374443));
#80792=CARTESIAN_POINT('Ctrl Pts',(158.677501178099,19.4360368307974,7.58006858495228));
#80793=CARTESIAN_POINT('Ctrl Pts',(158.932009582291,12.1040229474429,0.683975632031796));
#80794=CARTESIAN_POINT('Ctrl Pts',(158.930416705502,12.1702974965225,1.17958980410979));
#80795=CARTESIAN_POINT('Ctrl Pts',(158.92041914514,12.5870409518039,2.64301417293013));
#80796=CARTESIAN_POINT('Ctrl Pts',(158.86909234575,14.7263584434607,5.53345251032764));
#80797=CARTESIAN_POINT('Ctrl Pts',(158.806814253289,17.4846886516532,7.04870965268586));
#80798=CARTESIAN_POINT('Ctrl Pts',(158.767483782269,19.4310494383988,7.59712554092142));
#80799=CARTESIAN_POINT('Ctrl Pts',(158.982413200833,12.0208578366741,0.694683492639028));
#80800=CARTESIAN_POINT('Ctrl Pts',(158.981986164429,12.0874117152711,1.19804493497253));
#80801=CARTESIAN_POINT('Ctrl Pts',(158.979315439178,12.5059806562226,2.68407756599458));
#80802=CARTESIAN_POINT('Ctrl Pts',(158.965306441318,14.6565598452237,5.61670311382474));
#80803=CARTESIAN_POINT('Ctrl Pts',(158.946827845463,17.439145402284,7.14516758702218));
#80804=CARTESIAN_POINT('Ctrl Pts',(158.934105219764,19.4029639732595,7.69317824822104));
#80805=CARTESIAN_POINT('Ctrl Pts',(159.,11.9254048139712,0.706973474004927));
#80806=CARTESIAN_POINT('Ctrl Pts',(159.00000171853,11.9919467336188,1.21926673705316));
#80807=CARTESIAN_POINT('Ctrl Pts',(158.9999242729,12.4104763709029,2.73200584808425));
#80808=CARTESIAN_POINT('Ctrl Pts',(158.999990134689,14.5632439214126,5.72247751494749));
#80809=CARTESIAN_POINT('Ctrl Pts',(158.999816474445,17.3634751876538,7.29623017279508));
#80810=CARTESIAN_POINT('Ctrl Pts',(159.,19.3516469022616,7.8686833920948));
#80811=CARTESIAN_POINT('Ctrl Pts',(159.,11.877667246487,0.713119888211847));
#80812=CARTESIAN_POINT('Ctrl Pts',(159.,11.9442023908097,1.22988069138113));
#80813=CARTESIAN_POINT('Ctrl Pts',(159.,12.3627130409043,2.75595242400335));
#80814=CARTESIAN_POINT('Ctrl Pts',(159.,14.5165477492305,5.77538011759181));
#80815=CARTESIAN_POINT('Ctrl Pts',(159.,17.3255467234756,7.37182014405471));
#80816=CARTESIAN_POINT('Ctrl Pts',(159.,19.3259059134355,7.95671795563314));
#80817=CARTESIAN_POINT('',(158.9865805553,11.9795659353751,0.7));
#80818=CARTESIAN_POINT('Ctrl Pts',(159.,11.9468127170547,1.12856807664394));
#80819=CARTESIAN_POINT('Ctrl Pts',(159.,11.9599365154716,0.989641976333897));
#80820=CARTESIAN_POINT('Ctrl Pts',(158.993800259318,11.9710158214142,0.846323791357046));
#80821=CARTESIAN_POINT('Ctrl Pts',(158.9865805553,11.9795659353751,0.7));
#80822=CARTESIAN_POINT('Ctrl Pts',(158.900103546958,12.142660119676,0.700000641937268));
#80823=CARTESIAN_POINT('Ctrl Pts',(158.914774473624,12.1258656790557,0.700000471216242));
#80824=CARTESIAN_POINT('Ctrl Pts',(158.927982030209,12.1079029737679,0.700002383279373));
#80825=CARTESIAN_POINT('Ctrl Pts',(158.939638744862,12.0889925608362,0.70000265930596));
#80826=CARTESIAN_POINT('Ctrl Pts',(158.951368136716,12.0699642453974,0.700002937053517));
#80827=CARTESIAN_POINT('Ctrl Pts',(158.961528053397,12.0499751764678,0.700001686941725));
#80828=CARTESIAN_POINT('Ctrl Pts',(158.969987594995,12.0292206127076,0.700000867127216));
#80829=CARTESIAN_POINT('Ctrl Pts',(158.971443459613,12.0256488074655,0.700000726039319));
#80830=CARTESIAN_POINT('Ctrl Pts',(158.972848847494,12.0220542851633,0.700000608661327));
#80831=CARTESIAN_POINT('Ctrl Pts',(158.974202941169,12.0184379939656,0.700000537646669));
#80832=CARTESIAN_POINT('Ctrl Pts',(158.978981100364,12.0056772704263,0.700000287058879));
#80833=CARTESIAN_POINT('Ctrl Pts',(158.983100399885,11.9927008953147,0.700000282335583));
#80834=CARTESIAN_POINT('Ctrl Pts',(158.98655979805,11.9795632865321,0.700000341049772));
#80835=CARTESIAN_POINT('Origin',(145.,2.27826388829055E-15,3.94606880756866E-15));
#80836=CARTESIAN_POINT('',(158.671029640456,5.59378221735089,11.088715006927));
#80837=CARTESIAN_POINT('Origin',(145.,-0.606217782649103,0.350000000000003));
#80838=CARTESIAN_POINT('',(158.671029640456,6.80621778264911,10.388715006927));
#80839=CARTESIAN_POINT('Ctrl Pts',(158.671029640456,5.59378221735089,11.088715006927));
#80840=CARTESIAN_POINT('Ctrl Pts',(158.642904819311,5.80046894549334,10.9693843687961));
#80841=CARTESIAN_POINT('Ctrl Pts',(158.629834412239,6.00445828013108,10.8516110715312));
#80842=CARTESIAN_POINT('Ctrl Pts',(158.629834412239,6.39554171986893,10.6258189423229));
#80843=CARTESIAN_POINT('Ctrl Pts',(158.642904819311,6.59953105450666,10.508045645058));
#80844=CARTESIAN_POINT('Ctrl Pts',(158.671029640456,6.80621778264911,10.388715006927));
#80845=CARTESIAN_POINT('Origin',(145.,0.606217782649109,-0.349999999999996));
#80846=CARTESIAN_POINT('Origin',(150.,-1.33226762955019E-14,0.));
#80847=CARTESIAN_POINT('Ctrl Pts',(158.666552508001,19.8663782142289,-7.69531573590556));
#80848=CARTESIAN_POINT('Ctrl Pts',(158.70506309762,18.3356178296976,-7.31472446391732));
#80849=CARTESIAN_POINT('Ctrl Pts',(158.774612832515,15.8996513054051,-6.19397172155973));
#80850=CARTESIAN_POINT('Ctrl Pts',(158.863837927697,13.1859943058499,-3.64218218391034));
#80851=CARTESIAN_POINT('Ctrl Pts',(158.895432323316,12.2774103837893,-1.70534981330175));
#80852=CARTESIAN_POINT('Ctrl Pts',(158.900200939034,12.1398501039082,-0.679362733743279));
#80853=CARTESIAN_POINT('Ctrl Pts',(158.758824046361,19.8625594015549,-7.71040940270194));
#80854=CARTESIAN_POINT('Ctrl Pts',(158.789386050929,18.3279118906777,-7.33717508378104));
#80855=CARTESIAN_POINT('Ctrl Pts',(158.842478617173,15.881226389662,-6.22396382322616));
#80856=CARTESIAN_POINT('Ctrl Pts',(158.906660488852,13.1544214007013,-3.66586377475453));
#80857=CARTESIAN_POINT('Ctrl Pts',(158.928689909036,12.2421440184425,-1.71687228995627));
#80858=CARTESIAN_POINT('Ctrl Pts',(158.932009582291,12.1040229474433,-0.683975632034815));
#80859=CARTESIAN_POINT('Ctrl Pts',(158.931293562486,19.8383310071993,-7.80617092405117));
#80860=CARTESIAN_POINT('Ctrl Pts',(158.941286887852,18.2899779002915,-7.43431238755035));
#80861=CARTESIAN_POINT('Ctrl Pts',(158.957561307978,15.8208930349454,-6.31415574843048));
#80862=CARTESIAN_POINT('Ctrl Pts',(158.975659787015,13.0757115695514,-3.72243477075485));
#80863=CARTESIAN_POINT('Ctrl Pts',(158.981523215389,12.1595610473647,-1.74372603630125));
#80864=CARTESIAN_POINT('Ctrl Pts',(158.982413190896,12.0208578329538,-0.694683493121147));
#80865=CARTESIAN_POINT('Ctrl Pts',(159.,19.7925863683043,-7.98697432975181));
#80866=CARTESIAN_POINT('Ctrl Pts',(158.999850139758,18.2238049379903,-7.59681086660832));
#80867=CARTESIAN_POINT('Ctrl Pts',(158.999964678301,15.7334734686309,-6.43919229122094));
#80868=CARTESIAN_POINT('Ctrl Pts',(158.999857039542,12.9799611868347,-3.78961117372721));
#80869=CARTESIAN_POINT('Ctrl Pts',(159.000003581543,12.0640831050459,-1.77463059337493));
#80870=CARTESIAN_POINT('Ctrl Pts',(159.,11.9254048139716,-0.706973474008048));
#80871=CARTESIAN_POINT('Ctrl Pts',(159.,19.7696341894082,-8.07769167309342));
#80872=CARTESIAN_POINT('Ctrl Pts',(159.,18.1906199145078,-7.67818903355296));
#80873=CARTESIAN_POINT('Ctrl Pts',(159.,15.6897004416897,-6.50174671393536));
#80874=CARTESIAN_POINT('Ctrl Pts',(159.,12.9320743783783,-3.82316018062639));
#80875=CARTESIAN_POINT('Ctrl Pts',(159.,12.0163314172826,-1.79008769222358));
#80876=CARTESIAN_POINT('Ctrl Pts',(159.,11.8776672464874,-0.713119888214994));
#80877=CARTESIAN_POINT('',(158.9865805553,11.9795659353751,-0.7));
#80878=CARTESIAN_POINT('Ctrl Pts',(158.986559794035,11.9795632850285,-0.700000341243359));
#80879=CARTESIAN_POINT('Ctrl Pts',(158.983092985643,11.9927290439857,-0.700000368005174));
#80880=CARTESIAN_POINT('Ctrl Pts',(158.978970927741,12.0057044345014,-0.700000397309323));
#80881=CARTESIAN_POINT('Ctrl Pts',(158.974202995356,12.0184378742667,-0.70000053399841));
#80882=CARTESIAN_POINT('Ctrl Pts',(158.968537668188,12.0335679340913,-0.700000696414387));
#80883=CARTESIAN_POINT('Ctrl Pts',(158.96196068147,12.0483567216063,-0.700000957224616));
#80884=CARTESIAN_POINT('Ctrl Pts',(158.954513252864,12.0627266959769,-0.700000963176014));
#80885=CARTESIAN_POINT('Ctrl Pts',(158.94418889197,12.0826477733461,-0.700000971426428));
#80886=CARTESIAN_POINT('Ctrl Pts',(158.932243096067,12.1016692830457,-0.700000125593031));
#80887=CARTESIAN_POINT('Ctrl Pts',(158.918794292536,12.1195876530585,-0.699998810214277));
#80888=CARTESIAN_POINT('Ctrl Pts',(158.912855160605,12.1275005921721,-0.699998229329298));
#80889=CARTESIAN_POINT('Ctrl Pts',(158.906622332495,12.1351980550099,-0.699997625884579));
#80890=CARTESIAN_POINT('Ctrl Pts',(158.90010351009,12.142660453513,-0.699997406838467));
#80891=CARTESIAN_POINT('Ctrl Pts',(158.9865805553,11.9795659353751,-0.7));
#80892=CARTESIAN_POINT('Ctrl Pts',(158.993732330744,11.9710962675166,-0.84494706366045));
#80893=CARTESIAN_POINT('Ctrl Pts',(159.,11.9601689398254,-0.987181575154915));
#80894=CARTESIAN_POINT('Ctrl Pts',(159.,11.9468127170547,-1.12856807664394));
#80895=CARTESIAN_POINT('',(158.752212389381,19.8232298288527,-7.70962628430587));
#80896=CARTESIAN_POINT('Ctrl Pts',(159.,19.325905913425,-7.95671795563006));
#80897=CARTESIAN_POINT('Ctrl Pts',(159.,19.3270536862555,-7.95616651093077));
#80898=CARTESIAN_POINT('Ctrl Pts',(158.999997281692,19.3282014128021,-7.95561496081141));
#80899=CARTESIAN_POINT('Ctrl Pts',(158.999597040786,19.4126972786048,-7.91500032696979));
#80900=CARTESIAN_POINT('Ctrl Pts',(158.984861677683,19.4971388133456,-7.87369754969679));
#80901=CARTESIAN_POINT('Ctrl Pts',(158.930181269471,19.6379934364655,-7.80372244999905));
#80902=CARTESIAN_POINT('Ctrl Pts',(158.896925699169,19.693365974414,-7.77581497074403));
#80903=CARTESIAN_POINT('Ctrl Pts',(158.827213134256,19.7716384126688,-7.7360687598922));
#80904=CARTESIAN_POINT('Ctrl Pts',(158.792347045386,19.801086988096,-7.72099850711087));
#80905=CARTESIAN_POINT('Ctrl Pts',(158.752212389381,19.8232298288527,-7.70962628430586));
#80906=CARTESIAN_POINT('Ctrl Pts',(158.752121561149,19.8231768430187,-7.70983685270459));
#80907=CARTESIAN_POINT('Ctrl Pts',(158.731582665339,19.8345398203133,-7.70394690811278));
#80908=CARTESIAN_POINT('Ctrl Pts',(158.710372605511,19.8455141791983,-7.69970518087401));
#80909=CARTESIAN_POINT('Ctrl Pts',(158.688685765167,19.855968129435,-7.69722256756609));
#80910=CARTESIAN_POINT('Ctrl Pts',(158.681360078093,19.8594994123192,-7.69638395539709));
#80911=CARTESIAN_POINT('Ctrl Pts',(158.673979887952,19.8629712282948,-7.6957464775288));
#80912=CARTESIAN_POINT('Ctrl Pts',(158.666552508001,19.8663782142289,-7.69531573590556));
#80913=CARTESIAN_POINT('Origin',(158.6,-1.33226762955019E-14,0.));
#80914=CARTESIAN_POINT('',(158.752212389381,16.5883471303194,-13.312607474691));
#80915=CARTESIAN_POINT('Ctrl Pts',(159.,16.5536728370359,-12.7583664943589));
#80916=CARTESIAN_POINT('Ctrl Pts',(159.,16.553769172696,-12.759636406475));
#80917=CARTESIAN_POINT('Ctrl Pts',(158.999997280881,16.5538653938821,-12.7609063311805));
#80918=CARTESIAN_POINT('Ctrl Pts',(158.999596995634,16.5609397485414,-12.8543856334112));
#80919=CARTESIAN_POINT('Ctrl Pts',(158.984862761909,16.5673910141555,-12.9481615592624));
#80920=CARTESIAN_POINT('Ctrl Pts',(158.930184920107,16.5772181880231,-13.1051327735338));
#80921=CARTESIAN_POINT('Ctrl Pts',(158.896928735048,16.5807360420776,-13.1670432887789));
#80922=CARTESIAN_POINT('Ctrl Pts',(158.827214610095,16.5854512069735,-13.2547053638027));
#80923=CARTESIAN_POINT('Ctrl Pts',(158.79234789486,16.5871243179067,-13.2877445744541));
#80924=CARTESIAN_POINT('Ctrl Pts',(158.752212389381,16.5883471303194,-13.3126074746909));
#80925=CARTESIAN_POINT('Origin',(158.752212389381,-1.33226762955019E-14,
0.));
#80926=CARTESIAN_POINT('Ctrl Pts',(158.900200939034,6.65827043776022,-10.173737221248));
#80927=CARTESIAN_POINT('Ctrl Pts',(158.895432347252,7.61557664745235,-9.77987635534187));
#80928=CARTESIAN_POINT('Ctrl Pts',(158.872079379635,9.21302007886553,-9.6353471052812));
#80929=CARTESIAN_POINT('Ctrl Pts',(158.790452736159,12.8229465544963,-10.3829880519117));
#80930=CARTESIAN_POINT('Ctrl Pts',(158.717904052866,15.1374358047924,-11.8431673784125));
#80931=CARTESIAN_POINT('Ctrl Pts',(158.666552508001,16.5975280245508,-13.3571303467592));
#80932=CARTESIAN_POINT('Ctrl Pts',(158.932009582291,6.64435174663333,-10.1404035444583));
#80933=CARTESIAN_POINT('Ctrl Pts',(158.928689925699,7.60792219083362,-9.74357356362834));
#80934=CARTESIAN_POINT('Ctrl Pts',(158.912373874526,9.21463386586497,-9.59692459386624));
#80935=CARTESIAN_POINT('Ctrl Pts',(158.854097225383,12.8389771728877,-10.3494393282083));
#80936=CARTESIAN_POINT('Ctrl Pts',(158.799576633228,15.1545020279223,-11.8229195053978));
#80937=CARTESIAN_POINT('Ctrl Pts',(158.758824046361,16.6086901170957,-13.346276324573));
#80938=CARTESIAN_POINT('Ctrl Pts',(158.982413154157,6.61204246376521,-10.0630264992596));
#80939=CARTESIAN_POINT('Ctrl Pts',(158.981523183117,7.5898866548263,-9.658627764774));
#80940=CARTESIAN_POINT('Ctrl Pts',(158.977169550385,9.21740359778035,-9.50343043578347));
#80941=CARTESIAN_POINT('Ctrl Pts',(158.960909074438,12.8825188461311,-10.2499676480619));
#80942=CARTESIAN_POINT('Ctrl Pts',(158.944618652234,15.2177709380972,-11.7373117187695));
#80943=CARTESIAN_POINT('Ctrl Pts',(158.931293156547,16.6795080761494,-13.2774129196461));
#80944=CARTESIAN_POINT('Ctrl Pts',(159.,6.5749593952785,-9.97421678230864));
#80945=CARTESIAN_POINT('Ctrl Pts',(159.000003581526,7.56891173967652,-9.56048922231216));
#80946=CARTESIAN_POINT('Ctrl Pts',(158.999889253475,9.22002580642617,-9.39151272309116));
#80947=CARTESIAN_POINT('Ctrl Pts',(159.000005852929,12.9391234929089,-10.1137449872823));
#80948=CARTESIAN_POINT('Ctrl Pts',(158.99980017042,15.3167203543368,-11.5959080168584));
#80949=CARTESIAN_POINT('Ctrl Pts',(159.,16.8132158530914,-13.1473954366732));
#80950=CARTESIAN_POINT('Ctrl Pts',(159.,6.55641356238178,-9.92980162904894));
#80951=CARTESIAN_POINT('Ctrl Pts',(159.,7.55842209562936,-9.51140652163949));
#80952=CARTESIAN_POINT('Ctrl Pts',(159.,9.22130514590203,-9.33555705053295));
#80953=CARTESIAN_POINT('Ctrl Pts',(159.,12.9674322311801,-10.0455672242374));
#80954=CARTESIAN_POINT('Ctrl Pts',(159.,15.3662005373164,-11.5250819761712));
#80955=CARTESIAN_POINT('Ctrl Pts',(159.,16.880303287541,-13.0821595950062));
#80956=CARTESIAN_POINT('Ctrl Pts',(159.,6.95077498280114,-9.78195926890241));
#80957=CARTESIAN_POINT('Ctrl Pts',(159.,6.8350080840985,-9.86421985098201));
#80958=CARTESIAN_POINT('Ctrl Pts',(158.993725391353,6.71717606475046,-9.94487738541081));
#80959=CARTESIAN_POINT('Ctrl Pts',(158.9865805553,6.59600075033666,-10.0246084263455));
#80960=CARTESIAN_POINT('Ctrl Pts',(158.666552508001,16.5975280245508,-13.3571303467592));
#80961=CARTESIAN_POINT('Ctrl Pts',(158.688478427472,16.5936004546458,-13.3477844635065));
#80962=CARTESIAN_POINT('Ctrl Pts',(158.709985159363,16.5909492224783,-13.3370544028067));
#80963=CARTESIAN_POINT('Ctrl Pts',(158.730884621661,16.589528599894,-13.3251222380001));
#80964=CARTESIAN_POINT('Ctrl Pts',(158.738037395233,16.589042396396,-13.3210384930759));
#80965=CARTESIAN_POINT('Ctrl Pts',(158.745118989822,16.5887006767687,-13.3168136370273));
#80966=CARTESIAN_POINT('Ctrl Pts',(158.752121583121,16.5885026141289,-13.3124540709826));
#80967=CARTESIAN_POINT('Origin',(150.,-1.33226762955019E-14,0.));
#80968=CARTESIAN_POINT('Origin',(141.,11.0305012887935,-3.26619676656572));
#80969=CARTESIAN_POINT('',(141.,10.6441309582779,-3.16266914852471));
#80970=CARTESIAN_POINT('',(141.,10.9269736707525,-3.65256709708134));
#80971=CARTESIAN_POINT('Origin',(141.,10.9029500033804,-2.19674332223564));
#80972=CARTESIAN_POINT('',(141.,10.7994223853394,-2.58311365275127));
#80973=CARTESIAN_POINT('Origin',(141.,11.185792715855,-2.68664127079228));
#80974=CARTESIAN_POINT('',(141.,11.289320333896,-2.30027094027665));
#80975=CARTESIAN_POINT('Origin',(141.,12.1586535775562,-2.53320808086892));
#80976=CARTESIAN_POINT('',(150.,11.7525454562834,-2.42439173773414));
#80977=CARTESIAN_POINT('Origin',(141.,10.5406033402369,-3.54903947904034));
#80978=CARTESIAN_POINT('',(150.,11.3901987931398,-3.77668789453883));
#80979=CARTESIAN_POINT('Origin',(150.,0.,0.));
#80980=CARTESIAN_POINT('Origin',(141.,9.96288198200727,-4.9437822173509));
#80981=CARTESIAN_POINT('Origin',(150.,0.,0.));
#80982=CARTESIAN_POINT('',(150.,11.9795659353751,-0.7));
#80983=CARTESIAN_POINT('Origin',(150.,0.,0.));
#80984=CARTESIAN_POINT('',(150.,8.96580705540569,-7.97585756174453));
#80985=CARTESIAN_POINT('Origin',(141.,7.35391052434009,-8.34386001800126));
#80986=CARTESIAN_POINT('',(150.,7.97585756174453,-8.9658070554057));
#80987=CARTESIAN_POINT('Origin',(141.,9.26309883354377,-8.27314933988261));
#80988=CARTESIAN_POINT('Origin',(141.,5.59378221735088,-11.088715006927));
#80989=CARTESIAN_POINT('Origin',(141.,6.1562177826491,-9.26288198200727));
#80990=CARTESIAN_POINT('Origin',(150.,0.,0.));
#80991=CARTESIAN_POINT('Origin',(141.,3.54903947904032,-10.5406033402369));
#80992=CARTESIAN_POINT('Origin',(150.,0.,0.));
#80993=CARTESIAN_POINT('Origin',(141.,0.699999999999998,-11.1));
#80994=CARTESIAN_POINT('Origin',(150.,0.,0.));
#80995=CARTESIAN_POINT('Origin',(150.,0.,0.));
#80996=CARTESIAN_POINT('',(150.,-2.42439173773414,-11.7525454562834));
#80997=CARTESIAN_POINT('Origin',(141.,-3.54903947904034,-10.5406033402369));
#80998=CARTESIAN_POINT('Origin',(141.,-2.53320808086892,-12.1586535775562));
#80999=CARTESIAN_POINT('Origin',(141.,-6.80621778264911,-10.388715006927));
#81000=CARTESIAN_POINT('Origin',(141.,-4.9437822173509,-9.96288198200727));
#81001=CARTESIAN_POINT('Origin',(150.,0.,0.));
#81002=CARTESIAN_POINT('Origin',(141.,-7.3539105243401,-8.34386001800125));
#81003=CARTESIAN_POINT('Origin',(150.,0.,0.));
#81004=CARTESIAN_POINT('Origin',(141.,-9.26288198200727,-6.1562177826491));
#81005=CARTESIAN_POINT('Origin',(150.,0.,0.));
#81006=CARTESIAN_POINT('',(150.,-11.3901987931398,-3.77668789453882));
#81007=CARTESIAN_POINT('Origin',(141.,-10.9029500033804,-2.19674332223563));
#81008=CARTESIAN_POINT('',(150.,-11.7525454562834,-2.42439173773412));
#81009=CARTESIAN_POINT('Origin',(141.,-11.7963069144127,-3.8855042376736));
#81010=CARTESIAN_POINT('Origin',(141.,-12.4,0.700000000000002));
#81011=CARTESIAN_POINT('Origin',(141.,-11.1,-0.699999999999999));
#81012=CARTESIAN_POINT('Origin',(150.,0.,0.));
#81013=CARTESIAN_POINT('Origin',(141.,-10.9029500033804,2.19674332223564));
#81014=CARTESIAN_POINT('Origin',(150.,0.,0.));
#81015=CARTESIAN_POINT('Origin',(141.,-9.96288198200727,4.9437822173509));
#81016=CARTESIAN_POINT('Origin',(150.,0.,0.));
#81017=CARTESIAN_POINT('Origin',(150.,0.,0.));
#81018=CARTESIAN_POINT('',(150.,-8.9658070554057,7.97585756174453));
#81019=CARTESIAN_POINT('Origin',(141.,-7.35391052434009,8.34386001800126));
#81020=CARTESIAN_POINT('',(150.,-7.97585756174453,8.9658070554057));
#81021=CARTESIAN_POINT('Origin',(141.,-9.26309883354377,8.27314933988261));
#81022=CARTESIAN_POINT('Origin',(141.,-5.59378221735089,11.088715006927));
#81023=CARTESIAN_POINT('Origin',(141.,-6.1562177826491,9.26288198200727));
#81024=CARTESIAN_POINT('Origin',(150.,0.,0.));
#81025=CARTESIAN_POINT('Origin',(141.,-3.54903947904033,10.5406033402369));
#81026=CARTESIAN_POINT('Origin',(150.,0.,0.));
#81027=CARTESIAN_POINT('Origin',(141.,-0.699999999999999,11.1));
#81028=CARTESIAN_POINT('Origin',(150.,0.,0.));
#81029=CARTESIAN_POINT('Origin',(150.,0.,0.));
#81030=CARTESIAN_POINT('',(150.,2.42439173773413,11.7525454562834));
#81031=CARTESIAN_POINT('Origin',(141.,3.54903947904033,10.5406033402369));
#81032=CARTESIAN_POINT('Origin',(141.,2.53320808086891,12.1586535775562));
#81033=CARTESIAN_POINT('Origin',(141.,6.80621778264911,10.388715006927));
#81034=CARTESIAN_POINT('',(141.,5.59378221735089,11.088715006927));
#81035=CARTESIAN_POINT('',(141.,6.80621778264911,10.388715006927));
#81036=CARTESIAN_POINT('Origin',(141.,6.15621778264911,9.26288198200727));
#81037=CARTESIAN_POINT('',(150.,6.59600075033667,10.0246084263455));
#81038=CARTESIAN_POINT('Origin',(141.,5.59378221735089,11.088715006927));
#81039=CARTESIAN_POINT('Origin',(150.,0.,0.));
#81040=CARTESIAN_POINT('',(150.,7.97585756174453,8.9658070554057));
#81041=CARTESIAN_POINT('Origin',(141.,8.34386001800126,7.35391052434009));
#81042=CARTESIAN_POINT('',(150.,8.9658070554057,7.97585756174453));
#81043=CARTESIAN_POINT('Origin',(141.,8.27314933988261,9.26309883354377));
#81044=CARTESIAN_POINT('Origin',(141.,10.388715006927,6.80621778264911));
#81045=CARTESIAN_POINT('',(150.,10.0246084263455,6.59600075033667));
#81046=CARTESIAN_POINT('Origin',(141.,9.96288198200727,4.94378221735089));
#81047=CARTESIAN_POINT('',(150.,10.7246084263455,5.38356518503845));
#81048=CARTESIAN_POINT('Origin',(150.,0.,0.));
#81049=CARTESIAN_POINT('Origin',(141.,10.5406033402369,3.54903947904033));
#81050=CARTESIAN_POINT('Origin',(150.,0.,0.));
#81051=CARTESIAN_POINT('Origin',(150.,0.,0.));
#81052=CARTESIAN_POINT('',(150.,11.9795659353751,0.7));
#81053=CARTESIAN_POINT('Origin',(141.,11.1,-0.7));
#81054=CARTESIAN_POINT('',(141.,12.4,-0.7));
#81055=CARTESIAN_POINT('Origin',(141.,12.4,-0.7));
#81056=CARTESIAN_POINT('',(141.,12.4,0.7));
#81057=CARTESIAN_POINT('Origin',(141.,12.4,0.7));
#90341=UNCERTAINTY_MEASURE_WITH_UNIT(LENGTH_MEASURE(0.01),#90375,
'DISTANCE_ACCURACY_VALUE',
'Maximum model space distance between geometric entities at asserted c
onnectivities');
#90355=UNCERTAINTY_MEASURE_WITH_UNIT(LENGTH_MEASURE(0.01),#90375,
'DISTANCE_ACCURACY_VALUE',
'Maximum model space distance between geometric entities at asserted c
onnectivities');
#90360=(
GEOMETRIC_REPRESENTATION_CONTEXT(3)
GLOBAL_UNCERTAINTY_ASSIGNED_CONTEXT((#90341))
GLOBAL_UNIT_ASSIGNED_CONTEXT((#90375,#90377,#90378))
REPRESENTATION_CONTEXT('','3D')
);
#90374=(
GEOMETRIC_REPRESENTATION_CONTEXT(3)
GLOBAL_UNCERTAINTY_ASSIGNED_CONTEXT((#90355))
GLOBAL_UNIT_ASSIGNED_CONTEXT((#90375,#90377,#90378))
REPRESENTATION_CONTEXT('','3D')
);
#90375=(
LENGTH_UNIT()
NAMED_UNIT(*)
SI_UNIT(.MILLI.,.METRE.)
);
#90377=(
NAMED_UNIT(*)
PLANE_ANGLE_UNIT()
SI_UNIT($,.RADIAN.)
);
#90378=(
NAMED_UNIT(*)
SI_UNIT($,.STERADIAN.)
SOLID_ANGLE_UNIT()
);
#90383=SHAPE_DEFINITION_REPRESENTATION(#90401,#90444);
#90401=PRODUCT_DEFINITION_SHAPE('',$,#90463);
#90444=SHAPE_REPRESENTATION('',(#43275),#90360);
#90458=PRODUCT_DEFINITION_CONTEXT('part definition',#90514,'design');
#90463=PRODUCT_DEFINITION('2026-10-11-12-53-09-512',
'04_Inner_Ball_Race',#90481,#90458);
#90481=PRODUCT_DEFINITION_FORMATION('',$,#90520);
#90514=APPLICATION_CONTEXT(
'Core Data for Automotive Mechanical Design Process');
#90515=PRODUCT_CONTEXT('part definition',#90514,'mechanical');
#90520=PRODUCT('2026-10-11-12-53-09-512','04_Inner_Ball_Race',$,(#90515));
#90674=COLOUR_RGB('Sky Blue',0.24,0.69,0.87);
#90675=FILL_AREA_STYLE_COLOUR('',#90674);
#90676=FILL_AREA_STYLE('',(#90675));
#90677=SURFACE_STYLE_FILL_AREA(#90676);
#90678=SURFACE_SIDE_STYLE('',(#90677));
#90679=SURFACE_STYLE_USAGE(.BOTH.,#90678);
#90680=PRESENTATION_STYLE_ASSIGNMENT((#90679));
ENDSEC;
END-ISO-10303-21;
